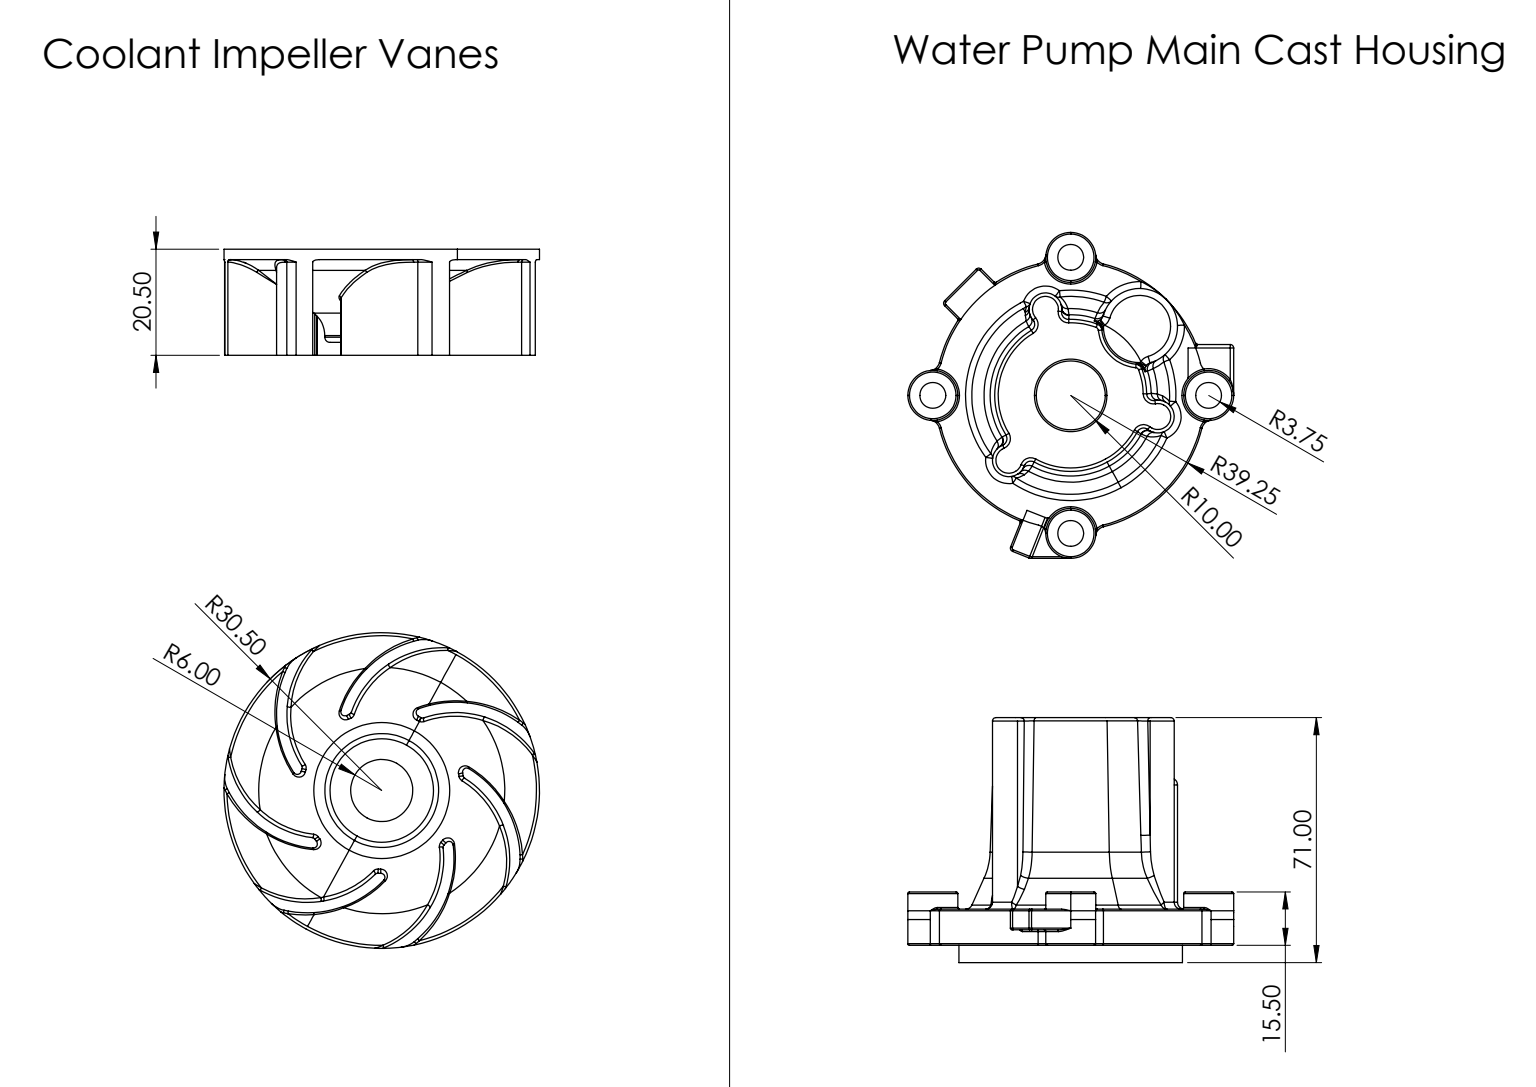
ISO-10303-21;
HEADER;
FILE_DESCRIPTION (('STEP AP214'),
    '1' );
FILE_NAME ('Coolant Impeller Vanes.step',
    '2026-10-09T13:19:41',
    ( '' ),
    ( '' ),
    'SwSTEP 2.0',
    'SolidWorks 2026',
    '' );
FILE_SCHEMA (( 'AUTOMOTIVE_DESIGN' ));
ENDSEC;

DATA;
#1=CARTESIAN_POINT ( 'NONE',  ( 13.86303783279999990, -99.69348480060000384, -10.38524229410000110 ) ) ;
#3=CARTESIAN_POINT ( 'NONE',  ( -4.209215656141860329, -99.16821844303207456, -18.57953415105935946 ) ) ;
#9=DIRECTION ( 'NONE',  ( 0.4377874319499604483, 0.000000000000000000, 0.8990785084889187928 ) ) ;
#10=CARTESIAN_POINT ( 'NONE',  ( 6.195449712719999447, -93.01125874769999768, -25.86806793289999717 ) ) ;
#12=CARTESIAN_POINT ( 'NONE',  ( -0.4517124965758896882, -92.59735406128710622, -30.49666433008702171 ) ) ;
#16=CARTESIAN_POINT ( 'NONE',  ( 0.000000000000000000, -101.2530993010000060, 0.000000000000000000 ) ) ;
#17=AXIS2_PLACEMENT_3D ( 'NONE', #8871, #7009, #22746 ) ;
#25=ORIENTED_EDGE ( 'NONE', *, *, #2852, .T. ) ;
#26=CARTESIAN_POINT ( 'NONE',  ( -13.83118819819999956, -93.00000000000000000, 21.42307711379999802 ) ) ;
#27=CARTESIAN_POINT ( 'NONE',  ( -6.649694310500000149, -97.57347470069998963, -20.16533349119999841 ) ) ;
#28=CARTESIAN_POINT ( 'NONE',  ( 7.286238495500000134, -101.2500498790000023, 13.33737010350000141 ) ) ;
#34=CARTESIAN_POINT ( 'NONE',  ( 6.962673371610000217, -93.00000450890000536, -28.64060071930000007 ) ) ;
#36=DIRECTION ( 'NONE',  ( 0.000000000000000000, 1.000000000000000000, 0.000000000000000000 ) ) ;
#37=CARTESIAN_POINT ( 'NONE',  ( -13.16349300034329239, -92.74292563041959170, 27.51314017236756015 ) ) ;
#41=CARTESIAN_POINT ( 'NONE',  ( -14.41816450560000007, -92.76166464580001048, 26.16031912729999931 ) ) ;
#42=DIRECTION ( 'NONE',  ( 0.4794255386042040601, 0.000000000000000000, 0.8775825618903719816 ) ) ;
#45=DIRECTION ( 'NONE',  ( 0.000000000000000000, -1.000000000000000000, 0.000000000000000000 ) ) ;
#48=CARTESIAN_POINT ( 'NONE',  ( 0.8512941674849999751, -100.5027207520000019, -16.22949194299999931 ) ) ;
#56=CARTESIAN_POINT ( 'NONE',  ( 28.37844821513105131, -92.77481473400868595, 11.17671000879152565 ) ) ;
#58=CARTESIAN_POINT ( 'NONE',  ( -4.347883707720000324, -95.85308664729998895, 22.07540195419999662 ) ) ;
#60=AXIS2_PLACEMENT_3D ( 'NONE', #11546, #27165, #75 ) ;
#61=CARTESIAN_POINT ( 'NONE',  ( 23.72908286170881098, -92.68577957607949713, -19.16202722645927281 ) ) ;
#62=CARTESIAN_POINT ( 'NONE',  ( 18.43702196799999982, -93.96464232210000489, 16.73647664110000122 ) ) ;
#67=CARTESIAN_POINT ( 'NONE',  ( -7.081475122079999629, -101.0678230150000019, 14.15032671260000008 ) ) ;
#70=CARTESIAN_POINT ( 'NONE',  ( -13.19299550116862640, -100.0559847774924549, -11.12607270767140477 ) ) ;
#75=DIRECTION ( 'NONE',  ( 1.000000000000000000, 0.000000000000000000, 0.000000000000000000 ) ) ;
#78=CARTESIAN_POINT ( 'NONE',  ( 11.12836528380000090, -101.0356131030000029, -10.75380786670000077 ) ) ;
#79=CARTESIAN_POINT ( 'NONE',  ( 16.21749840157504963, -94.69376227371040500, 17.23632262694635386 ) ) ;
#81=EDGE_CURVE ( 'NONE', #22088, #1149, #28672, .T. ) ;
#82=CARTESIAN_POINT ( 'NONE',  ( 26.66586753799999698, -92.50000000000000000, 13.56661073689999952 ) ) ;
#83=FACE_OUTER_BOUND ( 'NONE', #27486, .T. ) ;
#85=CARTESIAN_POINT ( 'NONE',  ( 21.68645939410062340, -94.27895761509498129, 13.53905968357343781 ) ) ;
#88=CIRCLE ( 'NONE', #11209, 30.50000000000000000 ) ;
#91=EDGE_CURVE ( 'NONE', #19757, #9289, #15248, .T. ) ;
#92=EDGE_LOOP ( 'NONE', ( #10026, #14439, #14720, #4638 ) ) ;
#95=CARTESIAN_POINT ( 'NONE',  ( -26.59811871830000030, -93.01125874769999768, -0.2839302173490000358 ) ) ;
#97=CARTESIAN_POINT ( 'NONE',  ( -13.14566783280000095, -99.53431386179998697, -11.42099844400000030 ) ) ;
#99=EDGE_LOOP ( 'NONE', ( #14663, #18599, #4684, #25899 ) ) ;
#104=AXIS2_PLACEMENT_3D ( 'NONE', #11589, #3684, #25016 ) ;
#106=ORIENTED_EDGE ( 'NONE', *, *, #502, .T. ) ;
#111=PLANE ( 'NONE',  #8405 ) ;
#112=CARTESIAN_POINT ( 'NONE',  ( 24.26002557130000170, -94.09272382170000526, -9.010767759849999337 ) ) ;
#115=CARTESIAN_POINT ( 'NONE',  ( -16.09522089960879399, -99.28262727489575923, 7.457865879375452423 ) ) ;
#116=B_SPLINE_SURFACE_WITH_KNOTS ( 'NONE', 5, 5, ( 
 ( #14625, #23526, #3562, #12417, #21334, #1390 ),
 ( #10232, #9826, #23801, #19147, #20920, #18734 ),
 ( #5874, #28035, #8074, #16964, #25852, #14753 ),
 ( #26709, #28718, #17525, #19703, #28300, #6299 ),
 ( #19988, #58, #13133, #10789, #8906, #15459 ),
 ( #11070, #6601, #22187, #4412, #6443, #17235 ) ),
 .UNSPECIFIED., .F., .F., .F.,
 ( 6, 6 ),
 ( 6, 6 ),
 ( 15.82769160610000014, 30.79604198849999719 ),
 ( 0.000000000000000000, 0.5000000000000000000 ),
 .UNSPECIFIED. ) ;
#118=CARTESIAN_POINT ( 'NONE',  ( -15.38823321699999980, -101.6484610359999863, 4.383952149800000697 ) ) ;
#124=ORIENTED_EDGE ( 'NONE', *, *, #22234, .T. ) ;
#126=CARTESIAN_POINT ( 'NONE',  ( 26.73456646982424445, -92.62800705135703083, -14.68054035958608772 ) ) ;
#129=EDGE_CURVE ( 'NONE', #4293, #10101, #28625, .T. ) ;
#130=EDGE_CURVE ( 'NONE', #14037, #19059, #13032, .T. ) ;
#137=CARTESIAN_POINT ( 'NONE',  ( 25.95077523760000204, -92.66001738319999959, 10.56845450099999972 ) ) ;
#139=VERTEX_POINT ( 'NONE', #26948 ) ;
#145=CARTESIAN_POINT ( 'NONE',  ( -12.45428620100000039, -94.22485739629999557, -21.30780079690000406 ) ) ;
#148=DIRECTION ( 'NONE',  ( 0.000000000000000000, 1.000000000000000000, 0.000000000000000000 ) ) ;
#149=CARTESIAN_POINT ( 'NONE',  ( -17.00715350810000004, -99.92967567080000890, 3.484608414699999823 ) ) ;
#154=CARTESIAN_POINT ( 'NONE',  ( 0.9512194931930000319, -99.70407914540000149, -17.16990763940000164 ) ) ;
#158=CARTESIAN_POINT ( 'NONE',  ( -7.593124578350000320, -94.98812656910000385, -22.45811535680000048 ) ) ;
#159=CIRCLE ( 'NONE', #18770, 16.00000000000000000 ) ;
#161=CARTESIAN_POINT ( 'NONE',  ( -23.83924287751435500, -92.80442066021429071, -19.02474555443098936 ) ) ;
#164=CARTESIAN_POINT ( 'NONE',  ( -14.62576901236522886, -101.1449112445098564, 4.605366063130757581 ) ) ;
#168=B_SPLINE_CURVE_WITH_KNOTS ( 'NONE', 3,
 ( #1213, #18961, #8023, #3928, #12792, #23335 ),
 .UNSPECIFIED., .F., .F.,
 ( 4, 2, 4 ),
 ( 0.000000000000000000, 0.5000000000000000000, 1.000000000000000000 ),
 .UNSPECIFIED. ) ;
#170=CIRCLE ( 'NONE', #22027, 0.8000000000000003775 ) ;
#179=CARTESIAN_POINT ( 'NONE',  ( 16.44117324919999845, -94.63960161729998788, 17.12038106740000032 ) ) ;
#180=CIRCLE ( 'NONE', #4826, 30.50000000000000000 ) ;
#181=CARTESIAN_POINT ( 'NONE',  ( 7.155402402981435372, -93.74885977083570765, -25.65720728536609840 ) ) ;
#182=CARTESIAN_POINT ( 'NONE',  ( -24.61280144410000048, -93.91547326130000783, -2.656926711870000180 ) ) ;
#185=CARTESIAN_POINT ( 'NONE',  ( 11.60289000694941208, -98.08323605844854853, -16.85433682801441435 ) ) ;
#186=ORIENTED_EDGE ( 'NONE', *, *, #11011, .T. ) ;
#189=CARTESIAN_POINT ( 'NONE',  ( -12.62382144519470906, -92.54938211474033949, 27.76503023812927395 ) ) ;
#194=CARTESIAN_POINT ( 'NONE',  ( 4.794255386040000566, -108.5000000000000000, 8.775825618900000791 ) ) ;
#196=EDGE_CURVE ( 'NONE', #27670, #21621, #4916, .T. ) ;
#198=CARTESIAN_POINT ( 'NONE',  ( 1.100347978140000071, -100.4792519539999915, -16.15648718290000119 ) ) ;
#210=DIRECTION ( 'NONE',  ( 0.000000000000000000, 1.000000000000000000, 0.000000000000000000 ) ) ;
#211=CARTESIAN_POINT ( 'NONE',  ( 14.90405967080000060, -97.14975741390000508, 15.22359678429999974 ) ) ;
#215=CARTESIAN_POINT ( 'NONE',  ( 18.38937822269999955, -93.75379239730000336, 16.85123465680000265 ) ) ;
#216=CARTESIAN_POINT ( 'NONE',  ( 0.000000000000000000, -108.5000000000000000, 0.000000000000000000 ) ) ;
#217=EDGE_CURVE ( 'NONE', #3543, #26971, #14750, .T. ) ;
#221=CARTESIAN_POINT ( 'NONE',  ( -12.45669907782013119, -101.5026031439933831, -10.21990696985948333 ) ) ;
#224=CARTESIAN_POINT ( 'NONE',  ( 7.375300558930000250, -99.32951138629999832, 16.07022401509999909 ) ) ;
#225=AXIS2_PLACEMENT_3D ( 'NONE', #24981, #531, #7212 ) ;
#229=CARTESIAN_POINT ( 'NONE',  ( 13.12744653600000078, -94.59276292389999696, -19.84842857619999990 ) ) ;
#233=CARTESIAN_POINT ( 'NONE',  ( 10.26951296328627450, -97.66504487118385214, 16.98417627201420643 ) ) ;
#235=CARTESIAN_POINT ( 'NONE',  ( 16.83483077069999823, -101.1889999979999999, 4.239603657359999112 ) ) ;
#240=CARTESIAN_POINT ( 'NONE',  ( 14.95019707169999990, -101.2530993000000024, 2.710463435110000319 ) ) ;
#244=DIRECTION ( 'NONE',  ( 1.000000000000000000, 0.000000000000000000, 0.000000000000000000 ) ) ;
#257=CARTESIAN_POINT ( 'NONE',  ( 15.94061401059999916, -100.1275643909999928, 4.799433088389999824 ) ) ;
#261=CARTESIAN_POINT ( 'NONE',  ( -19.90122868539999956, -97.01677120260001175, -7.153572992790000029 ) ) ;
#263=CARTESIAN_POINT ( 'NONE',  ( -30.47294111744043832, -92.56492639277982448, 1.288063236097679587 ) ) ;
#264=LINE ( 'NONE', #16101, #15060 ) ;
#272=CARTESIAN_POINT ( 'NONE',  ( -17.52930755215682268, -96.09960287657678180, 13.04485788190981488 ) ) ;
#273=ORIENTED_EDGE ( 'NONE', *, *, #13276, .F. ) ;
#274=DIRECTION ( 'NONE',  ( 0.000000000000000000, -1.000000000000000000, 0.000000000000000000 ) ) ;
#275=CARTESIAN_POINT ( 'NONE',  ( -3.794472973536972216, -98.68740021267650775, 19.30576947772378560 ) ) ;
#276=CARTESIAN_POINT ( 'NONE',  ( -12.75146816829999885, -100.4650220110000021, -10.99189795709999906 ) ) ;
#282=CARTESIAN_POINT ( 'NONE',  ( -1.332267629549999902E-15, -101.6484611540000031, 3.552713678799999608E-15 ) ) ;
#283=CARTESIAN_POINT ( 'NONE',  ( 0.3059185938709999553, -101.1889999979999999, 14.72672055670000013 ) ) ;
#284=CARTESIAN_POINT ( 'NONE',  ( 10.50737348100000013, -92.95010077049998642, 27.57035790109999596 ) ) ;
#286=B_SPLINE_CURVE_WITH_KNOTS ( 'NONE', 3,
 ( #13483, #9260, #22391, #17872, #13330, #22237 ),
 .UNSPECIFIED., .F., .F.,
 ( 4, 2, 4 ),
 ( 0.000000000000000000, 0.5000000000000000000, 1.000000000000000000 ),
 .UNSPECIFIED. ) ;
#289=CARTESIAN_POINT ( 'NONE',  ( -27.35150891653901084, -93.48480241393187384, -0.1005241429990150898 ) ) ;
#290=CARTESIAN_POINT ( 'NONE',  ( 19.72730657420000000, -94.57749572790000059, 14.01459989379999982 ) ) ;
#292=ORIENTED_EDGE ( 'NONE', *, *, #16592, .T. ) ;
#294=CARTESIAN_POINT ( 'NONE',  ( -25.34933364415341472, -93.66270333196791853, -5.750320990542998167 ) ) ;
#295=EDGE_CURVE ( 'NONE', #9549, #16619, #7522, .T. ) ;
#296=DIRECTION ( 'NONE',  ( -0.2162432783070587228, 0.000000000000000000, -0.9763395129702658881 ) ) ;
#298=CARTESIAN_POINT ( 'NONE',  ( -12.52668430659999999, -94.45168166330000759, -21.51447599709999992 ) ) ;
#299=CARTESIAN_POINT ( 'NONE',  ( -24.12300379919877713, -94.89420224095245260, -4.133214399626305102 ) ) ;
#303=CARTESIAN_POINT ( 'NONE',  ( -16.99615325119999909, -99.69348474340000621, 3.341833029000000010 ) ) ;
#306=CARTESIAN_POINT ( 'NONE',  ( -9.444188748147608337, -96.12507615671063377, -21.04386775914182905 ) ) ;
#308=CARTESIAN_POINT ( 'NONE',  ( 0.5505338958400000093, -101.0875971110000080, -15.39929819530000010 ) ) ;
#310=CARTESIAN_POINT ( 'NONE',  ( -11.92805169729999903, -93.25168459629999518, -23.54816055649999740 ) ) ;
#313=CARTESIAN_POINT ( 'NONE',  ( -23.96181287727355880, -92.68577957613881324, -18.87019301755865186 ) ) ;
#320=CARTESIAN_POINT ( 'NONE',  ( 17.35878545119999927, -99.60591458940000109, 0.7490350149880000696 ) ) ;
#325=CARTESIAN_POINT ( 'NONE',  ( 0.000000000000000000, -102.8486084350000027, 0.000000000000000000 ) ) ;
#327=EDGE_CURVE ( 'NONE', #28629, #9768, #11659, .T. ) ;
#328=CARTESIAN_POINT ( 'NONE',  ( 4.957296131405555251, -93.25521310932876418, -27.72106811766053980 ) ) ;
#335=CARTESIAN_POINT ( 'NONE',  ( 7.189062418559999834, -92.50000460620000808, -28.89817089330000144 ) ) ;
#337=CARTESIAN_POINT ( 'NONE',  ( -13.21000303337382675, -92.77521214512354675, 27.49085673672507468 ) ) ;
#340=CARTESIAN_POINT ( 'NONE',  ( -15.46453744689999965, -92.60980597189998775, 23.68301408729999835 ) ) ;
#343=CARTESIAN_POINT ( 'NONE',  ( -17.63662366879999865, -94.54719310779999830, 16.06392309460000334 ) ) ;
#344=CARTESIAN_POINT ( 'NONE',  ( 0.9125455711469999676, -100.1785804069999983, -16.62377051789999882 ) ) ;
#348=CARTESIAN_POINT ( 'NONE',  ( 6.888451995309999631, -99.53431386179998697, 15.99365561480000153 ) ) ;
#349=ORIENTED_EDGE ( 'NONE', *, *, #6891, .T. ) ;
#350=CARTESIAN_POINT ( 'NONE',  ( -17.51528407220000361, -94.37182379849998881, 16.53944417690000179 ) ) ;
#351=CARTESIAN_POINT ( 'NONE',  ( 15.38595020189201179, -101.1586404113103015, 2.789465265516761772 ) ) ;
#353=CARTESIAN_POINT ( 'NONE',  ( 19.89028060919999774, -94.80026829410000744, 14.17835456439999930 ) ) ;
#355=CARTESIAN_POINT ( 'NONE',  ( 23.48150327141549099, -92.56772982771099123, -19.46465348493570957 ) ) ;
#358=B_SPLINE_SURFACE_WITH_KNOTS ( 'NONE', 5, 5, ( 
 ( #10209, #18565, #20758, #23504, #23087, #27741, #25691, #27609, #3542 ),
 ( #25277, #12127, #816, #21309, #7649, #19123, #16212, #964, #25125 ),
 ( #5159, #25412, #3402, #14040, #9658, #22946, #14328, #16367, #23222 ),
 ( #11846, #27457, #5305, #3131, #20898, #16516, #5443, #3270, #21043 ),
 ( #1100, #7777, #16650, #25544, #14467, #23361, #23634, #1928, #28278 ),
 ( #19396, #15144, #19819, #4092, #28424, #23917, #3954, #12678, #10767 ) ),
 .UNSPECIFIED., .F., .F., .F.,
 ( 6, 6 ),
 ( 6, 3, 6 ),
 ( 10.27983419480000116, 28.98451109560000205 ),
 ( 0.000000000000000000, 0.2500000000000000000, 0.5000000000000000000 ),
 .UNSPECIFIED. ) ;
#362=CARTESIAN_POINT ( 'NONE',  ( -12.45203970512436165, -101.4728631013286559, -10.26186846076686443 ) ) ;
#373=CYLINDRICAL_SURFACE ( 'NONE', #27643, 15.99999999999999822 ) ;
#374=CARTESIAN_POINT ( 'NONE',  ( -14.95854026159999961, -100.9763033870000015, 4.709388778109999230 ) ) ;
#375=CARTESIAN_POINT ( 'NONE',  ( -17.31644382271060323, -99.07183861590023355, -8.238310338614811101 ) ) ;
#379=CARTESIAN_POINT ( 'NONE',  ( 0.000000000000000000, -101.6484611540000031, 0.000000000000000000 ) ) ;
#380=CARTESIAN_POINT ( 'NONE',  ( 24.72812962333588160, -93.39299082536693675, -12.36525841036616313 ) ) ;
#382=ORIENTED_EDGE ( 'NONE', *, *, #3847, .F. ) ;
#386=CARTESIAN_POINT ( 'NONE',  ( 23.63616061750000341, -94.63960162979999780, -2.179844042860000108 ) ) ;
#389=CARTESIAN_POINT ( 'NONE',  ( 29.11677867130000052, -92.50000000000000000, 6.880015861159999524 ) ) ;
#391=ADVANCED_FACE ( 'NONE', ( #7256 ), #13212, .F. ) ;
#393=CARTESIAN_POINT ( 'NONE',  ( 16.66712582699999956, -100.0994409990000094, 4.341523580040000496 ) ) ;
#397=EDGE_CURVE ( 'NONE', #15581, #14037, #15975, .T. ) ;
#399=CARTESIAN_POINT ( 'NONE',  ( -20.09682587570000223, -97.23151480800000002, -7.274462301079999804 ) ) ;
#401=CARTESIAN_POINT ( 'NONE',  ( -30.44002477821454633, -92.69183043801065480, 1.913949942781201674 ) ) ;
#402=DIRECTION ( 'NONE',  ( 0.6184463001828860440, 0.000000000000000000, 0.7858270635388550085 ) ) ;
#403=DIRECTION ( 'NONE',  ( 0.4794255386042042266, 0.000000000000000000, 0.8775825618903720926 ) ) ;
#406=CARTESIAN_POINT ( 'NONE',  ( 22.78264864029999970, -94.59276292120000562, -6.873201003520000185 ) ) ;
#407=TOROIDAL_SURFACE ( 'NONE', #6924, 18.14285714289999873, 0.5000000000000000000 ) ;
#410=CARTESIAN_POINT ( 'NONE',  ( 13.82833792859999811, -99.73367660430000115, -10.41122475269999903 ) ) ;
#411=ORIENTED_EDGE ( 'NONE', *, *, #8688, .T. ) ;
#415=CARTESIAN_POINT ( 'NONE',  ( -13.27698888679999989, -99.83167681540000160, -11.13684395419999973 ) ) ;
#416=CARTESIAN_POINT ( 'NONE',  ( -12.76745321220000129, -101.1364147039999892, -8.514038431850000421 ) ) ;
#417=CARTESIAN_POINT ( 'NONE',  ( 16.58537890990000108, -94.98812477769999418, 16.93952572510000110 ) ) ;
#427=CARTESIAN_POINT ( 'NONE',  ( 10.51978096080000213, -92.52763213160000078, 27.11043680749999751 ) ) ;
#430=CIRCLE ( 'NONE', #7407, 0.4999999999999993339 ) ;
#435=ORIENTED_EDGE ( 'NONE', *, *, #15676, .F. ) ;
#438=DIRECTION ( 'NONE',  ( 1.000000000000000000, 0.000000000000000000, 0.000000000000000000 ) ) ;
#439=CARTESIAN_POINT ( 'NONE',  ( -14.10155798110000092, -93.81709628049999594, -21.57370430179999943 ) ) ;
#440=CARTESIAN_POINT ( 'NONE',  ( -24.00582547640926379, -94.71481465629901209, -4.132763972591003032 ) ) ;
#441=ORIENTED_EDGE ( 'NONE', *, *, #13396, .T. ) ;
#443=CARTESIAN_POINT ( 'NONE',  ( -17.09009608839999927, -99.55609322370000314, 3.193624944930000265 ) ) ;
#446=ORIENTED_EDGE ( 'NONE', *, *, #18563, .T. ) ;
#447=B_SPLINE_CURVE_WITH_KNOTS ( 'NONE', 3,
 ( #7135, #24608, #16144, #11221, #2517, #21773, #21492, #4538, #15745, #9188 ),
 .UNSPECIFIED., .F., .F.,
 ( 4, 2, 2, 2, 4 ),
 ( 0.000000000000000000, 0.2500000000000000000, 0.5000000000000000000, 0.7500000000000000000, 1.000000000000000000 ),
 .UNSPECIFIED. ) ;
#449=DIRECTION ( 'NONE',  ( 0.000000000000000000, 1.000000000000000000, 0.000000000000000000 ) ) ;
#450=DIRECTION ( 'NONE',  ( 0.000000000000000000, -1.000000000000000000, 0.000000000000000000 ) ) ;
#457=AXIS2_PLACEMENT_3D ( 'NONE', #1882, #15240, #28107 ) ;
#460=CARTESIAN_POINT ( 'NONE',  ( 15.94843830448696487, -101.0147714271772088, 4.203990814596493486 ) ) ;
#465=B_SPLINE_CURVE_WITH_KNOTS ( 'NONE', 5,
 ( #5943, #23459, #23728, #10162, #18944, #17165, #14693, #26054, #14961, #21544, #25785, #21403 ),
 .UNSPECIFIED., .F., .F.,
 ( 6, 3, 3, 6 ),
 ( 0.000000000000000000, 0.4964111757582199136, 0.7833083924326244007, 1.000000000000000000 ),
 .UNSPECIFIED. ) ;
#475=CARTESIAN_POINT ( 'NONE',  ( 9.119802927630001221, -98.28914429610000525, 16.69368728350000097 ) ) ;
#485=CARTESIAN_POINT ( 'NONE',  ( 11.45574570990000041, -93.13207089280000162, -23.61394595179999811 ) ) ;
#487=CARTESIAN_POINT ( 'NONE',  ( -13.33479272893357859, -92.93978723899297734, 27.43052168310984840 ) ) ;
#491=CARTESIAN_POINT ( 'NONE',  ( 14.34373124439999891, -102.5000000000000000, 26.25602392650000283 ) ) ;
#493=CARTESIAN_POINT ( 'NONE',  ( -18.48642635659999911, -96.07607726710000406, 13.72266607319999920 ) ) ;
#494=CARTESIAN_POINT ( 'NONE',  ( 0.6457915530089999301, -99.58396362730000817, -17.35065848859999704 ) ) ;
#502=EDGE_CURVE ( 'NONE', #19526, #5924, #14185, .T. ) ;
#508=CARTESIAN_POINT ( 'NONE',  ( 10.14179094049999819, -99.62155479429999616, 14.52072615979999881 ) ) ;
#511=CARTESIAN_POINT ( 'NONE',  ( 26.37318048140000215, -93.00000450890000536, 13.16123783449999962 ) ) ;
#512=DIRECTION ( 'NONE',  ( 0.000000000000000000, 1.000000000000000000, 0.000000000000000000 ) ) ;
#514=CARTESIAN_POINT ( 'NONE',  ( -6.885095864830000245, -101.1417990620000040, 14.17428525849999943 ) ) ;
#516=CARTESIAN_POINT ( 'NONE',  ( -12.61948338259999858, -101.6484611540000031, -9.836088610590000059 ) ) ;
#520=CIRCLE ( 'NONE', #16773, 5.000000000000000888 ) ;
#521=CARTESIAN_POINT ( 'NONE',  ( 7.321257786130000333, -99.28585527969998736, 16.15667156069999777 ) ) ;
#523=CARTESIAN_POINT ( 'NONE',  ( -3.773308002759999891, -96.65227117080000596, -20.92579437230000039 ) ) ;
#531=DIRECTION ( 'NONE',  ( 0.000000000000000000, 1.000000000000000000, 0.000000000000000000 ) ) ;
#539=CIRCLE ( 'NONE', #15843, 30.50000000000000000 ) ;
#542=CARTESIAN_POINT ( 'NONE',  ( -19.01557598121447157, -92.50000000001456613, 22.91712378798360916 ) ) ;
#543=CARTESIAN_POINT ( 'NONE',  ( 28.83687378200000140, -92.50000647099999185, 7.262115126140000321 ) ) ;
#545=CARTESIAN_POINT ( 'NONE',  ( -19.98788946392987853, -95.81531090358907932, 9.701109111489476078 ) ) ;
#547=ORIENTED_EDGE ( 'NONE', *, *, #12350, .T. ) ;
#549=CARTESIAN_POINT ( 'NONE',  ( -24.15517241699999929, -94.98812769030000425, -4.102690932189999806 ) ) ;
#551=CARTESIAN_POINT ( 'NONE',  ( 8.639505966715979923, -92.69183043846588532, 29.25093587448420962 ) ) ;
#552=CARTESIAN_POINT ( 'NONE',  ( 0.3872056760440000245, -99.92967571559999840, -17.35614698070000017 ) ) ;
#557=DIRECTION ( 'NONE',  ( 0.9982579106777251798, 0.000000000000000000, -0.05900121837168281064 ) ) ;
#558=CIRCLE ( 'NONE', #25661, 18.64285714289999873 ) ;
#562=CARTESIAN_POINT ( 'NONE',  ( 14.21256893470000193, -98.58303758080000989, -12.13706782569999909 ) ) ;
#567=CARTESIAN_POINT ( 'NONE',  ( 7.891778559019607009, -101.5538022607323683, 14.00007649551812072 ) ) ;
#571=ADVANCED_FACE ( 'NONE', ( #26925 ), #15677, .T. ) ;
#572=CARTESIAN_POINT ( 'NONE',  ( 26.38387423984804769, -92.80045754842753070, -15.30171679607595259 ) ) ;
#573=ORIENTED_EDGE ( 'NONE', *, *, #1821, .F. ) ;
#576=CARTESIAN_POINT ( 'NONE',  ( -4.045235864600000397, -98.43722212099999069, 19.19069134749999961 ) ) ;
#578=CARTESIAN_POINT ( 'NONE',  ( 8.074115162410000934, -92.66424957140000629, 26.74225754210000261 ) ) ;
#589=EDGE_CURVE ( 'NONE', #21458, #13839, #9040, .T. ) ;
#590=CARTESIAN_POINT ( 'NONE',  ( 7.367077158260816994, -101.1416252679887577, 13.68480675837215799 ) ) ;
#596=CARTESIAN_POINT ( 'NONE',  ( -16.91403943069999727, -99.72583475830001021, 3.025870399720000048 ) ) ;
#602=CARTESIAN_POINT ( 'NONE',  ( 0.7331063123750001242, -99.53431386179998697, -17.39857302659999760 ) ) ;
#606=CARTESIAN_POINT ( 'NONE',  ( -9.465083148179999739, -93.62676565499999981, -23.38439984080000045 ) ) ;
#610=CARTESIAN_POINT ( 'NONE',  ( 16.28778070538160350, -100.5550990449209223, 4.345266980774773913 ) ) ;
#612=ORIENTED_EDGE ( 'NONE', *, *, #9543, .F. ) ;
#620=ORIENTED_EDGE ( 'NONE', *, *, #6006, .F. ) ;
#621=CARTESIAN_POINT ( 'NONE',  ( 0.000000000000000000, -102.5000000000000000, 0.000000000000000000 ) ) ;
#622=CARTESIAN_POINT ( 'NONE',  ( 9.335817441747641610, -98.58684426249028832, 16.46450815360437048 ) ) ;
#627=CARTESIAN_POINT ( 'NONE',  ( -22.27191869549999836, -94.59276292389999696, -8.381623179300000004 ) ) ;
#629=CARTESIAN_POINT ( 'NONE',  ( -18.14789115860000024, -98.53904439360000822, 4.701750000830000609 ) ) ;
#630=CARTESIAN_POINT ( 'NONE',  ( -0.5455113252076949637, -98.53908159007990264, -18.73906669024530913 ) ) ;
#632=EDGE_LOOP ( 'NONE', ( #19632, #17486, #11324, #22339 ) ) ;
#633=CARTESIAN_POINT ( 'NONE',  ( 13.03263341399999931, -94.63960343439998724, -19.83860458410000049 ) ) ;
#641=CARTESIAN_POINT ( 'NONE',  ( -18.40263696530000104, -95.90090461900000207, 13.63749173159999906 ) ) ;
#642=CARTESIAN_POINT ( 'NONE',  ( 0.7331063045040000503, -99.53431386179998697, -17.39857310140000024 ) ) ;
#649=ORIENTED_EDGE ( 'NONE', *, *, #27398, .T. ) ;
#652=CARTESIAN_POINT ( 'NONE',  ( 8.185345124539999517, -101.3150701389999995, 14.03998254610000096 ) ) ;
#653=ORIENTED_EDGE ( 'NONE', *, *, #17240, .T. ) ;
#657=CARTESIAN_POINT ( 'NONE',  ( -7.569816714379999922, -100.7776802639999971, 13.87827956499999971 ) ) ;
#658=CARTESIAN_POINT ( 'NONE',  ( -12.66558680574216922, -93.40492137171338527, -23.55307789253798845 ) ) ;
#661=CARTESIAN_POINT ( 'NONE',  ( 7.318052426040000391, -101.1822553929999913, 13.41977313900000013 ) ) ;
#662=ORIENTED_EDGE ( 'NONE', *, *, #22175, .F. ) ;
#667=ORIENTED_EDGE ( 'NONE', *, *, #3117, .T. ) ;
#670=CARTESIAN_POINT ( 'NONE',  ( 11.85549584000000145, -101.3350617309999961, -10.77753387699999976 ) ) ;
#672=CARTESIAN_POINT ( 'NONE',  ( 15.48878798707903925, -95.04305759974297985, 17.29288121155813585 ) ) ;
#679=CARTESIAN_POINT ( 'NONE',  ( -14.88706571849999882, -101.2269841009999993, 3.209819282999999857 ) ) ;
#683=CARTESIAN_POINT ( 'NONE',  ( -18.13877362739999910, -92.50000000000000000, -23.79298866759999598 ) ) ;
#685=CARTESIAN_POINT ( 'NONE',  ( 21.27776255609999723, -96.58372173029999885, 1.059637706860000028 ) ) ;
#690=CARTESIAN_POINT ( 'NONE',  ( 0.4125572470530000091, -92.84292833370000153, -30.36594662649999776 ) ) ;
#692=CARTESIAN_POINT ( 'NONE',  ( 16.40194905730000130, -100.1981337080000003, 4.404945126920000398 ) ) ;
#695=CARTESIAN_POINT ( 'NONE',  ( 8.185346967789998374, -101.3150701389999995, 14.03998109830000018 ) ) ;
#696=CARTESIAN_POINT ( 'NONE',  ( -22.25469472199999998, -96.07623048470000526, -5.897558151980000218 ) ) ;
#697=ORIENTED_EDGE ( 'NONE', *, *, #27258, .F. ) ;
#698=CARTESIAN_POINT ( 'NONE',  ( -30.48402335599918800, -92.52498922770503498, 0.9899291096564720727 ) ) ;
#701=DIRECTION ( 'NONE',  ( 0.000000000000000000, -1.000000000000000000, 0.000000000000000000 ) ) ;
#709=CARTESIAN_POINT ( 'NONE',  ( 14.00782577689999897, -96.65227117100000953, -15.99711037630000021 ) ) ;
#715=CARTESIAN_POINT ( 'NONE',  ( 11.77298154309999845, -101.2530993010000060, -9.604785791470000333 ) ) ;
#722=CARTESIAN_POINT ( 'NONE',  ( 2.631283596650000334, -94.29487537309999823, 25.29847487550000196 ) ) ;
#724=CARTESIAN_POINT ( 'NONE',  ( -11.18835776723661724, -94.77533639018899692, -20.78536094536529077 ) ) ;
#725=CIRCLE ( 'NONE', #16980, 18.64285714289999518 ) ;
#726=VERTEX_POINT ( 'NONE', #19037 ) ;
#727=CARTESIAN_POINT ( 'NONE',  ( -26.32546053305905076, -93.86130746203110675, -1.655768764585977548 ) ) ;
#740=CYLINDRICAL_SURFACE ( 'NONE', #28427, 5.000000000000000000 ) ;
#744=CARTESIAN_POINT ( 'NONE',  ( -15.62495981729999883, -101.3646851630000043, 3.472370199919999845 ) ) ;
#747=EDGE_LOOP ( 'NONE', ( #26424, #26914 ) ) ;
#749=CARTESIAN_POINT ( 'NONE',  ( -13.83118819819999956, -93.00000000000000000, 21.42307711379999802 ) ) ;
#752=DIRECTION ( 'NONE',  ( 1.000000000000000000, 0.000000000000000000, 0.000000000000000000 ) ) ;
#755=CARTESIAN_POINT ( 'NONE',  ( 15.63673621517384227, -101.5526869446983511, 3.723052656565844831 ) ) ;
#763=CARTESIAN_POINT ( 'NONE',  ( 2.113568700161239988, -94.60931859130616317, 24.93618714997996122 ) ) ;
#769=CARTESIAN_POINT ( 'NONE',  ( -5.360408304419999936, -101.0356131030000029, 14.51726283890000069 ) ) ;
#772=ADVANCED_FACE ( 'NONE', ( #13764 ), #9092, .T. ) ;
#784=CARTESIAN_POINT ( 'NONE',  ( 15.50655985760000100, -100.4792519539999915, 4.667916574389999518 ) ) ;
#788=CARTESIAN_POINT ( 'NONE',  ( -12.40956463280000044, -101.1716782170000073, -9.672470230850001016 ) ) ;
#791=CARTESIAN_POINT ( 'NONE',  ( -16.41347552970000123, -99.62149529559999905, 6.656434160910000841 ) ) ;
#795=DIRECTION ( 'NONE',  ( 1.000000000000000000, 0.000000000000000000, 0.000000000000000000 ) ) ;
#801=CARTESIAN_POINT ( 'NONE',  ( 12.48171397640000180, -98.43722862079999913, 15.12788944299999905 ) ) ;
#802=ORIENTED_EDGE ( 'NONE', *, *, #21545, .T. ) ;
#805=CARTESIAN_POINT ( 'NONE',  ( -11.67423268237357448, -95.07100787631300420, -21.41835470664000596 ) ) ;
#807=CARTESIAN_POINT ( 'NONE',  ( -17.09958374329999842, -92.50686295190000408, -23.80106955060000118 ) ) ;
#808=CARTESIAN_POINT ( 'NONE',  ( -7.939103275319999042, -100.2511768809999921, 14.67510867289999865 ) ) ;
#811=CYLINDRICAL_SURFACE ( 'NONE', #10352, 0.7499999999999991118 ) ;
#815=FACE_OUTER_BOUND ( 'NONE', #4729, .T. ) ;
#816=CARTESIAN_POINT ( 'NONE',  ( 12.08846704350000145, -99.82967635420000363, -13.24263972569999837 ) ) ;
#821=CARTESIAN_POINT ( 'NONE',  ( -18.09364012780129372, -92.54687141712491893, 24.55341606856252312 ) ) ;
#824=DIRECTION ( 'NONE',  ( 0.000000000000000000, -1.000000000000000000, 0.000000000000000000 ) ) ;
#825=CARTESIAN_POINT ( 'NONE',  ( -17.12548553040000243, -99.53431416519998720, 3.156821174210000081 ) ) ;
#828=CYLINDRICAL_SURFACE ( 'NONE', #23410, 16.00000000000000000 ) ;
#829=CARTESIAN_POINT ( 'NONE',  ( 7.493565752170000316, -101.1298585160000130, 13.45843171979999831 ) ) ;
#837=CARTESIAN_POINT ( 'NONE',  ( 13.81100091409999919, -101.1889999979999999, -10.51865105429999936 ) ) ;
#838=DIRECTION ( 'NONE',  ( 1.000000000000000000, 0.000000000000000000, 0.000000000000000000 ) ) ;
#840=CARTESIAN_POINT ( 'NONE',  ( -5.459548099580000091, -101.1364147039999892, 14.34189828759999941 ) ) ;
#841=CARTESIAN_POINT ( 'NONE',  ( -20.16249632440000283, -93.14733754460000625, 18.54048584069999706 ) ) ;
#842=VERTEX_POINT ( 'NONE', #27887 ) ;
#843=CARTESIAN_POINT ( 'NONE',  ( -30.43382723913022403, -92.71525149887465034, 2.010643618899957019 ) ) ;
#844=CARTESIAN_POINT ( 'NONE',  ( 0.5993989555620130583, -100.8061861239892067, -16.64687443652875132 ) ) ;
#848=CARTESIAN_POINT ( 'NONE',  ( 23.34631240599999913, -94.16701134370001114, -7.441733273619999700 ) ) ;
#850=CARTESIAN_POINT ( 'NONE',  ( 23.87011249777025412, -92.83160374581406415, -18.98598802258993246 ) ) ;
#856=CARTESIAN_POINT ( 'NONE',  ( 8.125631349740000786, -111.0000000000000000, 24.17072847820000092 ) ) ;
#857=CARTESIAN_POINT ( 'NONE',  ( 15.34608781240000042, -101.0356131030000029, 1.995616791270000023 ) ) ;
#866=CARTESIAN_POINT ( 'NONE',  ( -4.870171913750000137, -99.56347590840000805, 16.86609011349999676 ) ) ;
#867=CARTESIAN_POINT ( 'NONE',  ( 1.495931207609999980, -94.52292840100000149, 23.88472403519999787 ) ) ;
#869=ORIENTED_EDGE ( 'NONE', *, *, #25177, .F. ) ;
#874=CARTESIAN_POINT ( 'NONE',  ( -2.903039748510000351, -94.98812477769999418, 23.52859306979999943 ) ) ;
#877=DIRECTION ( 'NONE',  ( 0.000000000000000000, -1.000000000000000000, 0.000000000000000000 ) ) ;
#878=ORIENTED_EDGE ( 'NONE', *, *, #8574, .T. ) ;
#884=CARTESIAN_POINT ( 'NONE',  ( -15.68327981119999670, -101.1552388829999956, 3.291924952050000019 ) ) ;
#895=CARTESIAN_POINT ( 'NONE',  ( 16.39931659300885514, -100.4166221066841587, 4.355705164862286871 ) ) ;
#901=AXIS2_PLACEMENT_3D ( 'NONE', #9797, #12393, #21304 ) ;
#906=CARTESIAN_POINT ( 'NONE',  ( 3.767790178086171782, -94.00299386466799945, 25.81181420351906297 ) ) ;
#909=CARTESIAN_POINT ( 'NONE',  ( 22.85993602570000149, -94.54719592029999831, -6.820848577220000486 ) ) ;
#913=CARTESIAN_POINT ( 'NONE',  ( -5.598527377420000839, -101.2141467319999890, 14.18131542549999935 ) ) ;
#915=FACE_OUTER_BOUND ( 'NONE', #3176, .T. ) ;
#918=CARTESIAN_POINT ( 'NONE',  ( 23.52740994132569341, -94.89420224091314537, -6.742681588792337699 ) ) ;
#924=CARTESIAN_POINT ( 'NONE',  ( 19.88643906569999942, -97.93128678309999202, 2.148978528179999792 ) ) ;
#925=CARTESIAN_POINT ( 'NONE',  ( -20.57672323510000112, -92.65509245750000389, 18.55002133529999853 ) ) ;
#926=CARTESIAN_POINT ( 'NONE',  ( 14.80905440220000102, -101.2358105800000061, 3.500992360309999718 ) ) ;
#927=VERTEX_POINT ( 'NONE', #21470 ) ;
#932=CARTESIAN_POINT ( 'NONE',  ( -17.06681816329999890, -98.24294206849999966, 8.836829391780000265 ) ) ;
#941=EDGE_CURVE ( 'NONE', #25484, #19516, #6323, .T. ) ;
#950=CARTESIAN_POINT ( 'NONE',  ( 7.584268328590000330, -101.6484612600000048, 14.08825304710000026 ) ) ;
#955=CARTESIAN_POINT ( 'NONE',  ( -7.808702190560000034, -100.5027207520000019, 14.25290428609999971 ) ) ;
#959=LINE ( 'NONE', #23355, #1352 ) ;
#964=CARTESIAN_POINT ( 'NONE',  ( 11.50033716490000124, -99.57131247680000286, -13.08529392099999988 ) ) ;
#967=CYLINDRICAL_SURFACE ( 'NONE', #8348, 16.00000000000000711 ) ;
#974=CARTESIAN_POINT ( 'NONE',  ( -16.13894939720000110, -100.3684138120000000, 2.534589637169999854 ) ) ;
#976=EDGE_CURVE ( 'NONE', #2923, #24336, #19701, .T. ) ;
#977=B_SPLINE_CURVE_WITH_KNOTS ( 'NONE', 5,
 ( #1268, #16978, #25726, #6621, #28740, #10949, #22067, #6463, #6321, #3993, #21918, #12853 ),
 .UNSPECIFIED., .F., .F.,
 ( 6, 3, 3, 6 ),
 ( 0.000000000000000000, 0.4964111757593155927, 0.7833083924321462277, 1.000000000000000000 ),
 .UNSPECIFIED. ) ;
#978=CARTESIAN_POINT ( 'NONE',  ( 6.983903848129999758, -101.1716782170000073, 14.09890285740000060 ) ) ;
#980=CARTESIAN_POINT ( 'NONE',  ( -11.71812394180000005, -95.05064612279998926, -21.42448367849999968 ) ) ;
#983=CARTESIAN_POINT ( 'NONE',  ( 26.73328265790000202, -93.00000450890000536, -12.41349335419999989 ) ) ;
#987=ORIENTED_EDGE ( 'NONE', *, *, #21643, .T. ) ;
#988=CARTESIAN_POINT ( 'NONE',  ( -17.05934341600000081, -99.58396357329999660, 3.231284207160000310 ) ) ;
#992=CARTESIAN_POINT ( 'NONE',  ( 0.5973072979270338534, -100.4166221066882656, -16.95738706857987310 ) ) ;
#995=CARTESIAN_POINT ( 'NONE',  ( -12.53380938399999955, -99.91102932029998840, -11.37771751150000021 ) ) ;
#997=CARTESIAN_POINT ( 'NONE',  ( -6.754619094799999779, -97.17811284689999241, -19.41490638410000003 ) ) ;
#998=CARTESIAN_POINT ( 'NONE',  ( 13.90581089109999979, -96.83679385050000121, -16.07632342850000029 ) ) ;
#1002=EDGE_CURVE ( 'NONE', #1715, #20804, #12259, .T. ) ;
#1003=FILL_AREA_STYLE_COLOUR ( '', #22561 ) ;
#1004=AXIS2_PLACEMENT_3D ( 'NONE', #7236, #15807, #16248 ) ;
#1011=CARTESIAN_POINT ( 'NONE',  ( -2.163692630959999974, -97.01506441819999793, 20.66419130159999895 ) ) ;
#1013=VERTEX_POINT ( 'NONE', #20588 ) ;
#1015=CARTESIAN_POINT ( 'NONE',  ( -28.90627101076691119, -93.08694455166653370, 3.225356627808906751 ) ) ;
#1017=CARTESIAN_POINT ( 'NONE',  ( 1.535001344007000501, -93.33134965528456917, 26.92859106544546677 ) ) ;
#1019=CIRCLE ( 'NONE', #13531, 23.79684788999999867 ) ;
#1020=DIRECTION ( 'NONE',  ( 0.4794255386042041156, 0.000000000000000000, 0.8775825618903722036 ) ) ;
#1021=DIRECTION ( 'NONE',  ( 0.000000000000000000, -1.000000000000000000, 0.000000000000000000 ) ) ;
#1026=CARTESIAN_POINT ( 'NONE',  ( 7.525098751867413505, -101.3051320485135989, 13.97834179997459891 ) ) ;
#1029=PRODUCT_DEFINITION ( 'UNKNOWN', '', #24580, #27815 ) ;
#1034=CARTESIAN_POINT ( 'NONE',  ( -14.98642683749999982, -101.1746813909999929, 3.063272132379999846 ) ) ;
#1041=CARTESIAN_POINT ( 'NONE',  ( -7.919443313535407647, -100.1406256087997946, 15.25681078078310193 ) ) ;
#1043=EDGE_CURVE ( 'NONE', #4106, #10296, #15561, .T. ) ;
#1045=CARTESIAN_POINT ( 'NONE',  ( 15.73209904307306495, -101.3586211804324364, 3.965908164571182670 ) ) ;
#1047=ORIENTED_EDGE ( 'NONE', *, *, #26762, .F. ) ;
#1050=AXIS2_PLACEMENT_3D ( 'NONE', #23123, #18318, #2882 ) ;
#1051=CARTESIAN_POINT ( 'NONE',  ( 6.505013304209224856, -93.40023634520538565, 26.84593531204708938 ) ) ;
#1052=EDGE_LOOP ( 'NONE', ( #19310, #18086, #18495, #5928 ) ) ;
#1054=VERTEX_POINT ( 'NONE', #22778 ) ;
#1056=CARTESIAN_POINT ( 'NONE',  ( -6.285925807539999965, -101.5369810359999860, 14.71350185169999847 ) ) ;
#1064=CARTESIAN_POINT ( 'NONE',  ( 16.79767991550562201, -99.84800943041638277, 4.262183576306437516 ) ) ;
#1071=CARTESIAN_POINT ( 'NONE',  ( 24.01308097620000126, -92.92146929989999649, -18.61461950569999857 ) ) ;
#1076=ADVANCED_FACE ( 'NONE', ( #16501 ), #12110, .F. ) ;
#1079=CARTESIAN_POINT ( 'NONE',  ( -8.209463884390000743, -99.53431386179998697, 15.35748973489999969 ) ) ;
#1083=AXIS2_PLACEMENT_3D ( 'NONE', #14215, #2856, #27761 ) ;
#1095=CARTESIAN_POINT ( 'NONE',  ( 7.294752286439998734, -101.1411471520000021, 13.55045874839999875 ) ) ;
#1100=CARTESIAN_POINT ( 'NONE',  ( 10.68340813570000059, -96.16784750930000314, -20.42747610590000207 ) ) ;
#1101=EDGE_LOOP ( 'NONE', ( #18516, #25126, #4373, #25716 ) ) ;
#1103=B_SPLINE_CURVE_WITH_KNOTS ( 'NONE', 3,
 ( #9770, #5554, #23742, #18682, #27581, #25387, #8018, #5415, #3375, #10178, #3240, #19095, #16908, #25801, #5827, #6247, #3923, #15110, #4358, #6542, #4056, #26358, #12787, #14974, #12922, #28246, #1743, #1892, #15250, #21839, #24171, #21695, #10730 ),
 .UNSPECIFIED., .F., .F.,
 ( 4, 2, 1, 1, 2, 2, 1, 1, 1, 2, 2, 2, 1, 1, 2, 2, 1, 1, 2, 2, 4 ),
 ( 0.000000000000000000, 0.06250000000012244372, 0.09375000000017180701, 0.1093750000001865452, 0.1171875000001930262, 0.1250000000001995071, 0.1875000000001214029, 0.2187500000000817679, 0.2343750000000625888, 0.2421875000000536238, 0.2500000000000446310, 0.3750000000000313083, 0.4375000000000246470, 0.4687500000000220379, 0.4843750000000230371, 0.5000000000000239808, 0.6250000000000188738, 0.6875000000000155431, 0.7187500000000137668, 0.7500000000000119904, 1.000000000000000000 ),
 .UNSPECIFIED. ) ;
#1105=CARTESIAN_POINT ( 'NONE',  ( 11.96217641910000040, -101.6484611580000035, -10.62652795770000047 ) ) ;
#1108=CARTESIAN_POINT ( 'NONE',  ( -16.54318588419999969, -93.00000000000000000, 25.62368046950000178 ) ) ;
#1111=CARTESIAN_POINT ( 'NONE',  ( 11.91621941349511360, -101.5902664364218992, -10.74252197561657773 ) ) ;
#1113=CARTESIAN_POINT ( 'NONE',  ( 9.154723059868985047, -100.7167546688124986, 14.37589150456371279 ) ) ;
#1115=VERTEX_POINT ( 'NONE', #11677 ) ;
#1117=CARTESIAN_POINT ( 'NONE',  ( 13.79150630012393286, -97.05288880406236274, -15.91483940542160269 ) ) ;
#1119=CARTESIAN_POINT ( 'NONE',  ( -11.31832638660000079, -94.71194659750000255, -20.80844780490000190 ) ) ;
#1123=DIRECTION ( 'NONE',  ( 0.000000000000000000, 1.000000000000000000, 0.000000000000000000 ) ) ;
#1125=CARTESIAN_POINT ( 'NONE',  ( -18.09563929800284754, -93.31462968090272625, -21.26308191278070936 ) ) ;
#1127=ORIENTED_EDGE ( 'NONE', *, *, #23270, .T. ) ;
#1128=CARTESIAN_POINT ( 'NONE',  ( 8.069590842209999337, -101.0685850230000113, 13.92289867959999938 ) ) ;
#1129=CARTESIAN_POINT ( 'NONE',  ( -17.03413894869999723, -99.61736770250000461, 3.268853260370000235 ) ) ;
#1135=CARTESIAN_POINT ( 'NONE',  ( 0.5079992097761589775, -100.1240332945069724, -17.19565627508607264 ) ) ;
#1136=DIRECTION ( 'NONE',  ( 0.000000000000000000, -1.000000000000000000, 0.000000000000000000 ) ) ;
#1138=CARTESIAN_POINT ( 'NONE',  ( 13.25691510293539821, -92.77521214512113090, 27.46826507470851197 ) ) ;
#1143=CARTESIAN_POINT ( 'NONE',  ( 13.12744029750000152, -94.59276292389999696, -19.84843707589999795 ) ) ;
#1149=VERTEX_POINT ( 'NONE', #23899 ) ;
#1151=EDGE_CURVE ( 'NONE', #12597, #24336, #725, .T. ) ;
#1154=CARTESIAN_POINT ( 'NONE',  ( -28.83106611000000186, -92.65997669530000280, 3.154919777930000002 ) ) ;
#1157=ORIENTED_EDGE ( 'NONE', *, *, #26762, .T. ) ;
#1163=ORIENTED_EDGE ( 'NONE', *, *, #18541, .F. ) ;
#1166=CARTESIAN_POINT ( 'NONE',  ( -14.70126722260000030, -101.0847364069999941, 4.628494549459999163 ) ) ;
#1167=CARTESIAN_POINT ( 'NONE',  ( -16.54766221710000096, -100.0428544680000016, 2.640864489020000150 ) ) ;
#1171=AXIS2_PLACEMENT_3D ( 'NONE', #20331, #24861, #13775 ) ;
#1182=AXIS2_PLACEMENT_3D ( 'NONE', #13757, #17697, #2120 ) ;
#1188=CARTESIAN_POINT ( 'NONE',  ( -17.91520637925930615, -98.72564645249281057, 4.448055852924632347 ) ) ;
#1192=CARTESIAN_POINT ( 'NONE',  ( -5.983771968930000185, -101.2459394079999981, 14.78967057790000084 ) ) ;
#1195=CARTESIAN_POINT ( 'NONE',  ( -4.115583105835526112, -96.89152197809237066, -20.86381302798665160 ) ) ;
#1198=CARTESIAN_POINT ( 'NONE',  ( -13.01174968712481217, -101.6407018583229416, -9.320898687691189011 ) ) ;
#1204=CARTESIAN_POINT ( 'NONE',  ( -20.43643619460000238, -93.49011727610000833, 16.37406953600000037 ) ) ;
#1205=CARTESIAN_POINT ( 'NONE',  ( 16.79922297439999923, -99.53431386179998697, 4.586272525910000120 ) ) ;
#1208=CARTESIAN_POINT ( 'NONE',  ( 14.05983645159999895, -99.53431386179998697, -10.27466725399999881 ) ) ;
#1211=CARTESIAN_POINT ( 'NONE',  ( 7.102042752109999135, -101.6484611540000031, 14.33739825589999839 ) ) ;
#1213=CARTESIAN_POINT ( 'NONE',  ( 6.019093083229999586, -92.50000000000000000, 29.30685818879999971 ) ) ;
#1216=ADVANCED_FACE ( 'NONE', ( #13541 ), #4022, .F. ) ;
#1220=ORIENTED_EDGE ( 'NONE', *, *, #18993, .F. ) ;
#1229=DIRECTION ( 'NONE',  ( 0.000000000000000000, 1.000000000000000000, 0.000000000000000000 ) ) ;
#1230=ORIENTED_EDGE ( 'NONE', *, *, #13863, .F. ) ;
#1232=CARTESIAN_POINT ( 'NONE',  ( -23.87286787420000067, -93.96464232239999603, -7.079520382630000164 ) ) ;
#1238=DIRECTION ( 'NONE',  ( 0.000000000000000000, 1.000000000000000000, 0.000000000000000000 ) ) ;
#1240=DIRECTION ( 'NONE',  ( 0.000000000000000000, -1.000000000000000000, 0.000000000000000000 ) ) ;
#1242=DIRECTION ( 'NONE',  ( 0.3639667172450259391, 0.000000000000000000, -0.9314119543670669188 ) ) ;
#1250=CARTESIAN_POINT ( 'NONE',  ( -11.40589454009999848, -95.08268351149999376, -21.37599873950000173 ) ) ;
#1255=CARTESIAN_POINT ( 'NONE',  ( -18.58238019774981353, -93.25521310994808744, -21.15957345179030469 ) ) ;
#1262=ORIENTED_EDGE ( 'NONE', *, *, #8790, .F. ) ;
#1264=CARTESIAN_POINT ( 'NONE',  ( 0.3228164666304381702, -101.4085864806541650, -16.18225634051029971 ) ) ;
#1267=DIRECTION ( 'NONE',  ( 1.000000000000000000, 0.000000000000000000, 0.000000000000000000 ) ) ;
#1268=CARTESIAN_POINT ( 'NONE',  ( -8.209463884390000743, -99.53431386179998697, 15.35748973489999969 ) ) ;
#1270=CARTESIAN_POINT ( 'NONE',  ( 16.42966103859999905, -94.59276292389999696, 17.21499949629999904 ) ) ;
#1271=DIRECTION ( 'NONE',  ( 0.000000000000000000, -1.000000000000000000, 0.000000000000000000 ) ) ;
#1281=CARTESIAN_POINT ( 'NONE',  ( -28.19807706989999829, -92.76550115769998683, 1.645633876470000034 ) ) ;
#1288=EDGE_LOOP ( 'NONE', ( #18758, #28729, #17531 ) ) ;
#1292=CARTESIAN_POINT ( 'NONE',  ( -14.61698170120000029, -101.1363384779999990, 4.673707807969999628 ) ) ;
#1294=CARTESIAN_POINT ( 'NONE',  ( -15.04689636610000036, -101.1175442680000032, 3.135183322060000499 ) ) ;
#1298=ORIENTED_EDGE ( 'NONE', *, *, #3350, .F. ) ;
#1301=CARTESIAN_POINT ( 'NONE',  ( -7.728319723075819603, -100.8738282916487208, 14.69600823143309576 ) ) ;
#1307=ORIENTED_EDGE ( 'NONE', *, *, #295, .F. ) ;
#1308=EDGE_CURVE ( 'NONE', #23834, #22763, #12324, .T. ) ;
#1310=CARTESIAN_POINT ( 'NONE',  ( 6.719631698796779240, -100.6644468679725009, 15.36513027133983122 ) ) ;
#1312=EDGE_LOOP ( 'NONE', ( #4453, #28583, #27849, #15878 ) ) ;
#1314=CARTESIAN_POINT ( 'NONE',  ( 0.000000000000000000, -101.6484611540000031, 0.000000000000000000 ) ) ;
#1317=CARTESIAN_POINT ( 'NONE',  ( 27.46713810829999858, -92.96321833979999383, 9.765138773850001286 ) ) ;
#1318=CARTESIAN_POINT ( 'NONE',  ( -6.045971696259999639, -101.1411470200000053, 14.15183991680000020 ) ) ;
#1328=ORIENTED_EDGE ( 'NONE', *, *, #25383, .F. ) ;
#1329=CARTESIAN_POINT ( 'NONE',  ( -20.52527758500000132, -95.75647260690000451, -9.198302384599999826 ) ) ;
#1330=CARTESIAN_POINT ( 'NONE',  ( 9.017788245969780903, -92.49999918155076273, -27.43400824161624385 ) ) ;
#1332=CARTESIAN_POINT ( 'NONE',  ( 24.73701769899999903, -93.39359504719999450, -11.28691117220000173 ) ) ;
#1341=CARTESIAN_POINT ( 'NONE',  ( 21.94462607333390380, -96.36359510713519683, -0.1463646804548337788 ) ) ;
#1342=CARTESIAN_POINT ( 'NONE',  ( 23.96368475870000125, -101.1889999979999999, 8.717328305520000598 ) ) ;
#1344=DIRECTION ( 'NONE',  ( 1.000000000000000000, 0.000000000000000000, 0.000000000000000000 ) ) ;
#1350=CARTESIAN_POINT ( 'NONE',  ( -12.36495966000000024, -101.1848541609999899, -8.980491836739998845 ) ) ;
#1352=VECTOR ( 'NONE', #1229, 1000.000000000000000 ) ;
#1354=CARTESIAN_POINT ( 'NONE',  ( 1.673545578960000224, -92.65509162889999573, 27.65323681370000131 ) ) ;
#1358=CARTESIAN_POINT ( 'NONE',  ( 12.66014534235611322, -101.5526869446726153, -9.904007292906472415 ) ) ;
#1359=B_SPLINE_CURVE_WITH_KNOTS ( 'NONE', 3,
 ( #8352, #25446, #12573, #23258, #18890, #3301, #8085, #27772, #21077, #10386, #1138, #25724, #5755, #23538, #9975, #27907, #25588, #5615, #21486, #14496, #28185, #23397, #3439, #12304, #19022, #1544, #16835, #25864, #3575, #11089, #4426, #13297, #3992 ),
 .UNSPECIFIED., .F., .F.,
 ( 4, 2, 1, 1, 2, 2, 1, 1, 1, 2, 2, 2, 1, 1, 2, 2, 1, 1, 2, 2, 4 ),
 ( 0.000000000000000000, 0.06249999999986458055, 0.09374999999978507470, 0.1093749999997540440, 0.1171874999997460920, 0.1249999999997381261, 0.1874999999997520594, 0.2187499999997566669, 0.2343749999997590261, 0.2421874999997645772, 0.2499999999997701283, 0.3749999999998100964, 0.4374999999998272493, 0.4687499999998345768, 0.4843749999998410716, 0.4999999999998475664, 0.6249999999998780975, 0.6874999999998955280, 0.7187499999999057421, 0.7499999999999159561, 1.000000000000000000 ),
 .UNSPECIFIED. ) ;
#1362=CARTESIAN_POINT ( 'NONE',  ( 0.3059185938709999553, -93.00000000000000000, 14.72672055670000013 ) ) ;
#1366=CARTESIAN_POINT ( 'NONE',  ( 11.50679452860000040, -101.1848541609999899, -10.05659687459999851 ) ) ;
#1372=DIRECTION ( 'NONE',  ( 0.000000000000000000, -1.000000000000000000, 0.000000000000000000 ) ) ;
#1374=CARTESIAN_POINT ( 'NONE',  ( 0.002146109654809999837, -101.6311724339999927, -16.01369408300000075 ) ) ;
#1382=CIRCLE ( 'NONE', #17641, 5.000000000000000888 ) ;
#1384=CARTESIAN_POINT ( 'NONE',  ( 6.719470054089999422, -100.4650220110000021, 15.43601254670000067 ) ) ;
#1385=CARTESIAN_POINT ( 'NONE',  ( 15.64536997099999915, -101.3878691800000098, 3.811131059900000118 ) ) ;
#1387=CARTESIAN_POINT ( 'NONE',  ( -11.63405728910000114, -94.86303146849999735, -21.38493624129999660 ) ) ;
#1389=CARTESIAN_POINT ( 'NONE',  ( 5.376469156563769225, -92.59033770611050329, -30.02271131604222987 ) ) ;
#1390=CARTESIAN_POINT ( 'NONE',  ( -8.209474437350001708, -99.53431242750001218, 15.35746870819999899 ) ) ;
#1391=CARTESIAN_POINT ( 'NONE',  ( 8.067175576580000396, -93.91547326120000605, -23.40448531159999845 ) ) ;
#1393=ORIENTED_EDGE ( 'NONE', *, *, #27899, .F. ) ;
#1396=CARTESIAN_POINT ( 'NONE',  ( 6.114061450880000415, -111.0000000000000000, -13.40104985119999981 ) ) ;
#1399=ORIENTED_EDGE ( 'NONE', *, *, #11498, .F. ) ;
#1402=CARTESIAN_POINT ( 'NONE',  ( 0.3445358076898260014, -101.3846248973681838, -16.20041589813614280 ) ) ;
#1403=CARTESIAN_POINT ( 'NONE',  ( 6.018657797749999538, -100.4792519539999915, 15.03391506150000012 ) ) ;
#1406=EDGE_CURVE ( 'NONE', #18883, #9768, #15708, .T. ) ;
#1409=DIRECTION ( 'NONE',  ( 0.000000000000000000, 1.000000000000000000, 0.000000000000000000 ) ) ;
#1410=CARTESIAN_POINT ( 'NONE',  ( 24.33297166435627190, -93.99439547207676071, -9.447863160898569035 ) ) ;
#1415=ORIENTED_EDGE ( 'NONE', *, *, #25728, .T. ) ;
#1428=EDGE_CURVE ( 'NONE', #22101, #2397, #23522, .T. ) ;
#1432=AXIS2_PLACEMENT_3D ( 'NONE', #23804, #12705, #1805 ) ;
#1433=CARTESIAN_POINT ( 'NONE',  ( -22.25450259269999975, -94.89197151650000706, -8.089821617090001027 ) ) ;
#1437=CARTESIAN_POINT ( 'NONE',  ( 0.000000000000000000, -107.1975888269999899, 0.000000000000000000 ) ) ;
#1438=CARTESIAN_POINT ( 'NONE',  ( -14.34373124439999891, -92.50000000000000000, -26.25602392650000283 ) ) ;
#1439=ORIENTED_EDGE ( 'NONE', *, *, #13143, .F. ) ;
#1443=CARTESIAN_POINT ( 'NONE',  ( -7.681814765061617756, -100.9570234913570488, 14.64644060644491574 ) ) ;
#1446=DIRECTION ( 'NONE',  ( 0.000000000000000000, 1.000000000000000000, 0.000000000000000000 ) ) ;
#1450=CARTESIAN_POINT ( 'NONE',  ( 6.659152648053978218, -101.1248211537192958, 14.99462091354799220 ) ) ;
#1455=AXIS2_PLACEMENT_3D ( 'NONE', #12126, #21042, #8048 ) ;
#1458=CARTESIAN_POINT ( 'NONE',  ( 27.17390343950000187, -92.54807936089999032, 9.505859965289999991 ) ) ;
#1462=CARTESIAN_POINT ( 'NONE',  ( -3.292855076097166656, -97.38870237746982639, -20.36241341912896985 ) ) ;
#1466=CARTESIAN_POINT ( 'NONE',  ( 16.83483077069999823, -99.92967571559999840, 4.239603657359999112 ) ) ;
#1470=EDGE_CURVE ( 'NONE', #1149, #13839, #11901, .T. ) ;
#1471=CARTESIAN_POINT ( 'NONE',  ( 15.83524192907358596, -101.5839620086842956, 2.606923154417748467 ) ) ;
#1472=CARTESIAN_POINT ( 'NONE',  ( -20.27478635940000373, -94.70873263889998839, 12.26043739520000031 ) ) ;
#1473=CARTESIAN_POINT ( 'NONE',  ( 23.55422583189999841, -93.65023553250000532, -9.043238345449999827 ) ) ;
#1479=AXIS2_PLACEMENT_3D ( 'NONE', #19800, #8292, #21709 ) ;
#1480=CARTESIAN_POINT ( 'NONE',  ( -15.21246488650000117, -100.9405327639999967, 4.776672761669999545 ) ) ;
#1482=CARTESIAN_POINT ( 'NONE',  ( 20.52749306944123830, -97.43022994675339987, 1.376655802589148880 ) ) ;
#1485=FACE_OUTER_BOUND ( 'NONE', #1288, .T. ) ;
#1487=SHAPE_REPRESENTATION_RELATIONSHIP ( 'NONE' , 'NONE' ,  #10908, #15419 ) ;
#1488=VERTEX_POINT ( 'NONE', #20921 ) ;
#1496=CARTESIAN_POINT ( 'NONE',  ( -12.54641657280000011, -101.1292389600000092, -9.112281375189999366 ) ) ;
#1498=CARTESIAN_POINT ( 'NONE',  ( -7.903212057390000211, -99.83167681540000160, 15.42228797350000136 ) ) ;
#1500=CARTESIAN_POINT ( 'NONE',  ( -2.986711171310000079, -94.79581646409999962, 23.48470800579999818 ) ) ;
#1503=DIRECTION ( 'NONE',  ( 0.000000000000000000, -1.000000000000000000, 0.000000000000000000 ) ) ;
#1505=CARTESIAN_POINT ( 'NONE',  ( 12.88080974073147189, -101.3846248973631958, -9.831425157082634314 ) ) ;
#1506=PLANE ( 'NONE',  #14915 ) ;
#1507=CARTESIAN_POINT ( 'NONE',  ( -16.91430575710000284, -100.0771588430000065, 3.341621066080000091 ) ) ;
#1513=ORIENTED_EDGE ( 'NONE', *, *, #4915, .T. ) ;
#1514=CYLINDRICAL_SURFACE ( 'NONE', #7223, 18.64285714290000229 ) ;
#1520=ORIENTED_EDGE ( 'NONE', *, *, #196, .T. ) ;
#1521=CARTESIAN_POINT ( 'NONE',  ( 6.649881675840000561, -101.0405520670000072, 14.82396520390000028 ) ) ;
#1522=CARTESIAN_POINT ( 'NONE',  ( 15.60420274139999997, -101.2927714249999980, 3.777748170229999758 ) ) ;
#1525=CARTESIAN_POINT ( 'NONE',  ( 3.787197165510000296, -93.00000000000000000, -30.26395773239999798 ) ) ;
#1526=CARTESIAN_POINT ( 'NONE',  ( 3.355978770230000130, -90.50000000000000000, 6.143077933229999843 ) ) ;
#1528=CARTESIAN_POINT ( 'NONE',  ( 3.263855493430000365, -92.57423544259999915, -28.67967719789999848 ) ) ;
#1531=CARTESIAN_POINT ( 'NONE',  ( -1.869200974745226063, -93.63284908718598842, 25.01357699951009295 ) ) ;
#1533=CIRCLE ( 'NONE', #3842, 18.64285714289999873 ) ;
#1537=EDGE_CURVE ( 'NONE', #23472, #19113, #3292, .T. ) ;
#1540=ORIENTED_EDGE ( 'NONE', *, *, #12604, .F. ) ;
#1541=CARTESIAN_POINT ( 'NONE',  ( -0.7205257404120000153, -101.5369810359999860, -15.98376809940000065 ) ) ;
#1544=CARTESIAN_POINT ( 'NONE',  ( 13.83675081990681122, -92.54938211476543586, 27.18091423687219788 ) ) ;
#1548=VECTOR ( 'NONE', #13237, 1000.000000000000000 ) ;
#1552=CARTESIAN_POINT ( 'NONE',  ( 14.28941763439999946, -93.00000000000000000, -3.575252188409999921 ) ) ;
#1555=CIRCLE ( 'NONE', #27139, 15.19391340349999986 ) ;
#1561=DIRECTION ( 'NONE',  ( 0.000000000000000000, -1.000000000000000000, 0.000000000000000000 ) ) ;
#1564=ADVANCED_FACE ( 'NONE', ( #16388 ), #3011, .T. ) ;
#1565=CARTESIAN_POINT ( 'NONE',  ( 15.35943464070000175, -100.7833805400000102, 4.159771655669999291 ) ) ;
#1573=AXIS2_PLACEMENT_3D ( 'NONE', #13511, #6979, #438 ) ;
#1578=ORIENTED_EDGE ( 'NONE', *, *, #18993, .T. ) ;
#1579=CARTESIAN_POINT ( 'NONE',  ( 22.83659466689194062, -95.90275867365805595, -4.923095664741855337 ) ) ;
#1580=CARTESIAN_POINT ( 'NONE',  ( -11.69640386740000082, -101.0875971110000080, -10.03173011250000002 ) ) ;
#1582=CARTESIAN_POINT ( 'NONE',  ( -7.501065465934297016, -101.2145573445136222, 14.51273970916295752 ) ) ;
#1588=VERTEX_POINT ( 'NONE', #25714 ) ;
#1589=ADVANCED_FACE ( 'NONE', ( #13916 ), #28211, .T. ) ;
#1592=EDGE_CURVE ( 'NONE', #16528, #28629, #10836, .T. ) ;
#1593=DIRECTION ( 'NONE',  ( 0.000000000000000000, 1.000000000000000000, 0.000000000000000000 ) ) ;
#1597=DIRECTION ( 'NONE',  ( 0.000000000000000000, -1.000000000000000000, 0.000000000000000000 ) ) ;
#1605=CARTESIAN_POINT ( 'NONE',  ( -14.15498507100000047, -93.99830544900000007, -21.64661225829999935 ) ) ;
#1608=CARTESIAN_POINT ( 'NONE',  ( -18.71306389469999942, -96.65227117089999354, -10.09692839740000103 ) ) ;
#1609=CARTESIAN_POINT ( 'NONE',  ( 13.51933813770000015, -100.3517545579999961, -9.891026358559999565 ) ) ;
#1611=CARTESIAN_POINT ( 'NONE',  ( 23.80455697029999840, -93.92589062420000801, -8.153550017880000667 ) ) ;
#1616=VERTEX_POINT ( 'NONE', #15913 ) ;
#1620=CARTESIAN_POINT ( 'NONE',  ( 20.65093475452214022, -97.34036579196893513, 1.255409981387750173 ) ) ;
#1623=CARTESIAN_POINT ( 'NONE',  ( 29.11677867130000052, -92.50000000000000000, 6.880015861159999524 ) ) ;
#1629=ORIENTED_EDGE ( 'NONE', *, *, #14978, .T. ) ;
#1632=ORIENTED_EDGE ( 'NONE', *, *, #14850, .F. ) ;
#1634=CARTESIAN_POINT ( 'NONE',  ( -13.23436873610000042, -101.5317765570000006, -9.147552046289998628 ) ) ;
#1635=DIRECTION ( 'NONE',  ( 0.9863585068926603583, 0.000000000000000000, 0.1646113479699432003 ) ) ;
#1642=CYLINDRICAL_SURFACE ( 'NONE', #4136, 20.64285714289999163 ) ;
#1644=CARTESIAN_POINT ( 'NONE',  ( 12.60821841358252193, -101.5829753080987814, -9.932320047300365218 ) ) ;
#1645=DIRECTION ( 'NONE',  ( 0.000000000000000000, 1.000000000000000000, 0.000000000000000000 ) ) ;
#1647=CARTESIAN_POINT ( 'NONE',  ( 7.181689689069999716, -99.92967571559999840, 15.80535034289999885 ) ) ;
#1648=ORIENTED_EDGE ( 'NONE', *, *, #18541, .T. ) ;
#1653=CARTESIAN_POINT ( 'NONE',  ( -20.59421057834115842, -93.07145594888166329, 16.81328959876951856 ) ) ;
#1658=CARTESIAN_POINT ( 'NONE',  ( 15.76644911200000188, -101.6484611580000035, 2.726874312449999671 ) ) ;
#1662=CARTESIAN_POINT ( 'NONE',  ( 6.540410660740000104, -100.9364576079999978, 14.54829053200000111 ) ) ;
#1663=CARTESIAN_POINT ( 'NONE',  ( -15.61689027843468480, -92.57936004669802799, -24.03289022899482674 ) ) ;
#1664=ADVANCED_FACE ( 'NONE', ( #15461 ), #15415, .F. ) ;
#1669=CARTESIAN_POINT ( 'NONE',  ( 9.010434747179999704, -94.45168166339999516, -23.20781253819999890 ) ) ;
#1671=CARTESIAN_POINT ( 'NONE',  ( 6.954809927569434613, -101.6297509123136535, 14.42559876608666514 ) ) ;
#1672=CARTESIAN_POINT ( 'NONE',  ( 1.673548719218163061, -92.65509297688285528, 27.65323130849352395 ) ) ;
#1675=CARTESIAN_POINT ( 'NONE',  ( -12.73945486129048454, -100.6338045024292995, -10.94379842081711551 ) ) ;
#1676=ORIENTED_EDGE ( 'NONE', *, *, #12743, .T. ) ;
#1677=CARTESIAN_POINT ( 'NONE',  ( -1.283022169079999886, -101.3150705500000157, -16.20107500659999644 ) ) ;
#1678=DIRECTION ( 'NONE',  ( 1.000000000000000000, 0.000000000000000000, 0.000000000000000000 ) ) ;
#1679=B_SPLINE_CURVE_WITH_KNOTS ( 'NONE', 5,
 ( #23387, #16240, #20639, #25153, #20785, #1128, #14068, #12155, #695 ),
 .UNSPECIFIED., .F., .F.,
 ( 6, 3, 6 ),
 ( 0.000000000000000000, 0.5000000000000000000, 1.000000000000000000 ),
 .UNSPECIFIED. ) ;
#1681=CARTESIAN_POINT ( 'NONE',  ( 16.15437062272748037, -94.72386903546126291, 17.24227625337255176 ) ) ;
#1684=CARTESIAN_POINT ( 'NONE',  ( -15.39276618183619583, -101.4254873439999329, 4.250919977501043334 ) ) ;
#1688=DIRECTION ( 'NONE',  ( 0.000000000000000000, 1.000000000000000000, 0.000000000000000000 ) ) ;
#1690=DIRECTION ( 'NONE',  ( 1.000000000000000000, 0.000000000000000000, 0.000000000000000000 ) ) ;
#1693=ADVANCED_FACE ( 'NONE', ( #13878 ), #7601, .F. ) ;
#1694=ORIENTED_EDGE ( 'NONE', *, *, #22234, .F. ) ;
#1696=CARTESIAN_POINT ( 'NONE',  ( -29.44685991679999759, -92.54628605920001405, 6.396492330759999234 ) ) ;
#1700=VERTEX_POINT ( 'NONE', #25115 ) ;
#1707=CARTESIAN_POINT ( 'NONE',  ( -15.29947873360000088, -101.1716782170000073, 3.671501766180000459 ) ) ;
#1708=CARTESIAN_POINT ( 'NONE',  ( -22.00137621023848666, -95.57586223585661855, -5.105060933739808959 ) ) ;
#1710=VERTEX_POINT ( 'NONE', #9929 ) ;
#1712=CARTESIAN_POINT ( 'NONE',  ( -12.58639594889999991, -100.8746138070000029, -10.82789256390000077 ) ) ;
#1713=EDGE_CURVE ( 'NONE', #19059, #1149, #27914, .T. ) ;
#1715=VERTEX_POINT ( 'NONE', #25265 ) ;
#1717=CARTESIAN_POINT ( 'NONE',  ( -0.9302893022191279782, -101.6077248516953091, -16.00345022493254632 ) ) ;
#1720=ORIENTED_EDGE ( 'NONE', *, *, #25096, .T. ) ;
#1723=CARTESIAN_POINT ( 'NONE',  ( 6.669678980424931680, -101.2145573445209408, 14.91311433900129124 ) ) ;
#1725=EDGE_LOOP ( 'NONE', ( #14448, #4958, #14088, #20508 ) ) ;
#1726=CARTESIAN_POINT ( 'NONE',  ( -19.97841359259663463, -95.83493812764778852, 9.662536293482050453 ) ) ;
#1731=CARTESIAN_POINT ( 'NONE',  ( -3.236852559049167244, -97.42330309947865885, -20.32638677250028891 ) ) ;
#1733=EDGE_LOOP ( 'NONE', ( #13344, #12764, #17680, #18232 ) ) ;
#1736=CARTESIAN_POINT ( 'NONE',  ( -18.26810397560000254, -94.98812477769999418, 16.32728546869999775 ) ) ;
#1739=CARTESIAN_POINT ( 'NONE',  ( 12.67716433170000023, -100.8815367389999977, -9.218731588149999823 ) ) ;
#1743=CARTESIAN_POINT ( 'NONE',  ( 29.90142803373326430, -92.53260370668940027, 6.013043342471341646 ) ) ;
#1751=CARTESIAN_POINT ( 'NONE',  ( 0.04581334808960710325, -92.83865970263813949, -30.49996578665741964 ) ) ;
#1754=AXIS2_PLACEMENT_3D ( 'NONE', #18412, #27301, #9794 ) ;
#1764=CARTESIAN_POINT ( 'NONE',  ( -13.00841234930000034, -100.9763228559999959, -8.758810206009998822 ) ) ;
#1765=B_SPLINE_SURFACE_WITH_KNOTS ( 'NONE', 5, 5, ( 
 ( #27754, #27623, #7793, #23237, #978, #18727, #20772, #16084, #5018 ),
 ( #24985, #13907, #25428, #20624, #12140, #27474, #5458, #7520, #14341 ),
 ( #5321, #16664, #3284, #9531, #25562, #14478, #18433, #27322, #25291 ),
 ( #7363, #16226, #3142, #25140, #14209, #14054, #3003, #23101, #11998 ),
 ( #28030, #12832, #19003, #7928, #25848, #17377, #26270, #6292, #4108 ),
 ( #3692, #15159, #28294, #27883, #1662, #14748, #10365, #19279, #12554 ),
 ( #24068, #17085, #1521, #21744, #28167, #16812, #5735, #1793, #23933 ),
 ( #8066, #16957, #12979, #14619, #21891, #3972, #19138, #3831, #8328 ),
 ( #25708, #1384, #5869, #8199, #10500, #19414, #23649, #21466, #25978 ),
 ( #6004, #14884, #26121, #10639, #10085, #12411, #23520, #8475, #23793 ),
 ( #19551, #12693, #17230, #21607, #3556, #21325, #10227, #6149, #15019 ),
 ( #28440, #2524, #15903, #24662, #4693, #9193, #15301, #27001, #348 ) ),
 .UNSPECIFIED., .F., .F., .F.,
 ( 6, 3, 3, 6 ),
 ( 6, 3, 6 ),
 ( 0.8942436407639999807, 1.876087175710000166, 3.176036816339999902, 5.425307607549999744 ),
 ( 0.000000000000000000, 0.2500000000000000000, 0.5000000000000000000 ),
 .UNSPECIFIED. ) ;
#1767=CARTESIAN_POINT ( 'NONE',  ( 8.185346967789998374, -101.1889999979999999, 14.03998109830000018 ) ) ;
#1770=CARTESIAN_POINT ( 'NONE',  ( -29.74546239500669031, -92.83865970263998690, 6.742216160683305759 ) ) ;
#1774=CARTESIAN_POINT ( 'NONE',  ( 13.62782804938226100, -100.4211561362012333, -10.10291547818408908 ) ) ;
#1777=CARTESIAN_POINT ( 'NONE',  ( -15.69013080879999933, -101.5700432450000079, 3.430602099230000146 ) ) ;
#1778=ORIENTED_EDGE ( 'NONE', *, *, #20203, .T. ) ;
#1784=ADVANCED_FACE ( 'NONE', ( #5432 ), #27992, .T. ) ;
#1787=CARTESIAN_POINT ( 'NONE',  ( -0.1068060827170000116, -101.3256027139999986, -15.90648277770000085 ) ) ;
#1789=CARTESIAN_POINT ( 'NONE',  ( 14.95019707159999989, -101.2530993000000024, 2.710463435300000334 ) ) ;
#1792=ORIENTED_EDGE ( 'NONE', *, *, #3223, .F. ) ;
#1793=CARTESIAN_POINT ( 'NONE',  ( 6.130772363030000172, -100.7776802639999971, 14.57128679989999931 ) ) ;
#1794=CARTESIAN_POINT ( 'NONE',  ( 15.61826386989999982, -101.5964542560000012, 3.655520785480000256 ) ) ;
#1796=AXIS2_PLACEMENT_3D ( 'NONE', #16588, #449, #9298 ) ;
#1799=CARTESIAN_POINT ( 'NONE',  ( 4.060520888432426645, -92.92035259772417533, -30.22975431335808594 ) ) ;
#1803=CARTESIAN_POINT ( 'NONE',  ( 6.508840722400000445, -93.07154530319999708, -26.20378082560000266 ) ) ;
#1804=ADVANCED_FACE ( 'NONE', ( #10471 ), #5652, .T. ) ;
#1805=DIRECTION ( 'NONE',  ( 1.000000000000000000, 0.000000000000000000, 0.000000000000000000 ) ) ;
#1806=CARTESIAN_POINT ( 'NONE',  ( -6.863006950479999979, -101.6484611540000031, 14.45362438769999969 ) ) ;
#1807=ORIENTED_EDGE ( 'NONE', *, *, #16120, .T. ) ;
#1811=CARTESIAN_POINT ( 'NONE',  ( 25.50885178510000273, -93.36531860459999166, -5.860088577239999985 ) ) ;
#1812=CARTESIAN_POINT ( 'NONE',  ( -1.303833584549999980, -101.1364147039999892, -15.29041300709999796 ) ) ;
#1821=EDGE_CURVE ( 'NONE', #15112, #10772, #1555, .T. ) ;
#1822=CARTESIAN_POINT ( 'NONE',  ( 0.000000000000000000, -94.59276292389999696, 0.000000000000000000 ) ) ;
#1831=EDGE_CURVE ( 'NONE', #6421, #3937, #6162, .T. ) ;
#1836=CARTESIAN_POINT ( 'NONE',  ( -25.52588841249999874, -93.67384740769999496, -2.372690985960000276 ) ) ;
#1841=CARTESIAN_POINT ( 'NONE',  ( 15.73597609990000024, -101.0405520670000072, 4.043504278899999527 ) ) ;
#1844=CARTESIAN_POINT ( 'NONE',  ( -13.14229048259999999, -100.8869813350000015, -8.528548640909999534 ) ) ;
#1845=ORIENTED_EDGE ( 'NONE', *, *, #10335, .T. ) ;
#1850=B_SPLINE_CURVE_WITH_KNOTS ( 'NONE', 5,
 ( #10509, #3704, #1672, #1953, #1531, #10376 ),
 .UNSPECIFIED., .F., .F.,
 ( 6, 6 ),
 ( 0.000000000000000000, 1.000000000000000000 ),
 .UNSPECIFIED. ) ;
#1851=EDGE_CURVE ( 'NONE', #17518, #1013, #13144, .T. ) ;
#1858=CARTESIAN_POINT ( 'NONE',  ( -12.49636764419999935, -101.4908759489999994, -10.04157132919999995 ) ) ;
#1859=CARTESIAN_POINT ( 'NONE',  ( -29.71161737690000137, -93.00000000000000000, 6.352311025380000586 ) ) ;
#1860=ORIENTED_EDGE ( 'NONE', *, *, #26039, .T. ) ;
#1861=AXIS2_PLACEMENT_3D ( 'NONE', #17056, #5971, #17345 ) ;
#1862=CIRCLE ( 'NONE', #27464, 0.8000000000000003775 ) ;
#1863=CARTESIAN_POINT ( 'NONE',  ( -0.9821106753968790182, -101.5839620086842814, -16.01831432786889664 ) ) ;
#1867=CARTESIAN_POINT ( 'NONE',  ( -5.390285367900000679, -100.8869813350000015, 14.71056643040000012 ) ) ;
#1870=CARTESIAN_POINT ( 'NONE',  ( -19.26625410581794995, -97.04909278841957132, 7.359652529508150742 ) ) ;
#1873=CARTESIAN_POINT ( 'NONE',  ( -15.43525743989999910, -101.1461852590000063, 4.782895807790000120 ) ) ;
#1882=CARTESIAN_POINT ( 'NONE',  ( -14.42556421679999978, -92.50000000000000000, -2.978755036369999942 ) ) ;
#1885=CARTESIAN_POINT ( 'NONE',  ( -18.77234060500000012, -92.65715406920001840, -20.69363841459999875 ) ) ;
#1886=CARTESIAN_POINT ( 'NONE',  ( -15.94434063720000161, -93.10431551199999944, 24.00277150759999856 ) ) ;
#1887=ORIENTED_EDGE ( 'NONE', *, *, #6683, .T. ) ;
#1888=EDGE_CURVE ( 'NONE', #4529, #22228, #12584, .T. ) ;
#1889=CARTESIAN_POINT ( 'NONE',  ( 12.67342850500000040, -100.8685038539999965, -9.320488510950001526 ) ) ;
#1892=CARTESIAN_POINT ( 'NONE',  ( 29.91164248172746198, -92.52640451552758805, 5.961874894218010645 ) ) ;
#1896=FACE_OUTER_BOUND ( 'NONE', #24576, .T. ) ;
#1897=CARTESIAN_POINT ( 'NONE',  ( -24.56259648705387022, -92.50000000000000000, -18.08169719992735480 ) ) ;
#1899=CARTESIAN_POINT ( 'NONE',  ( 0.03433565797716789381, -92.82709422631805296, -30.49998078697906578 ) ) ;
#1905=CARTESIAN_POINT ( 'NONE',  ( 17.67606731260000075, -99.62155223519999936, 1.124352996140000061 ) ) ;
#1910=CARTESIAN_POINT ( 'NONE',  ( 14.91172220540000026, -95.31428172910000285, 17.37540928339999979 ) ) ;
#1913=DIRECTION ( 'NONE',  ( 1.000000000000000000, 0.000000000000000000, 0.000000000000000000 ) ) ;
#1928=CARTESIAN_POINT ( 'NONE',  ( 10.17429874589999983, -95.72998414199999218, -19.97250627529999889 ) ) ;
#1931=CARTESIAN_POINT ( 'NONE',  ( -17.06129450210000087, -93.25667418180000823, 21.77310057969999946 ) ) ;
#1932=CARTESIAN_POINT ( 'NONE',  ( 12.01015229399999917, -101.6484611540000031, -9.798277495349999811 ) ) ;
#1935=CARTESIAN_POINT ( 'NONE',  ( 0.6434015132710000362, -100.4650220110000021, -16.82283554099999989 ) ) ;
#1940=EDGE_LOOP ( 'NONE', ( #1439, #20708, #6249, #12128, #12080 ) ) ;
#1942=CARTESIAN_POINT ( 'NONE',  ( 15.52117313229999951, -101.2902355740000075, 3.579205768200000026 ) ) ;
#1950=CARTESIAN_POINT ( 'NONE',  ( 3.404243284160000105, -93.04780269100000112, -28.95354108839999796 ) ) ;
#1953=CARTESIAN_POINT ( 'NONE',  ( -0.2283525300826651505, -93.01584921915402049, 26.42460210401236154 ) ) ;
#1956=CARTESIAN_POINT ( 'NONE',  ( -13.25237707705474399, -99.99762666416590662, -11.12887180797588194 ) ) ;
#1959=CARTESIAN_POINT ( 'NONE',  ( 25.60466699379999866, -93.13207089229999269, -5.766591832619999636 ) ) ;
#1961=CARTESIAN_POINT ( 'NONE',  ( -1.526197323679999940, -100.8869817940000075, -15.59251925729999932 ) ) ;
#1968=CARTESIAN_POINT ( 'NONE',  ( -14.58939485729999852, -101.2530991829999891, 4.248445246460000213 ) ) ;
#1969=CIRCLE ( 'NONE', #18251, 20.64285714289999873 ) ;
#1972=CARTESIAN_POINT ( 'NONE',  ( 13.78283651632031770, -100.0559847774664775, -10.38643546923515970 ) ) ;
#1974=( NAMED_UNIT ( * ) SI_UNIT ( $, .STERADIAN. ) SOLID_ANGLE_UNIT ( ) );
#1983=CARTESIAN_POINT ( 'NONE',  ( -18.88944331899999796, -101.1889999979999999, -23.13319212550000259 ) ) ;
#1987=EDGE_CURVE ( 'NONE', #10101, #14792, #11184, .T. ) ;
#1999=CARTESIAN_POINT ( 'NONE',  ( -17.58226716778080956, -94.81956704558760407, 15.60250440155592422 ) ) ;
#2001=AXIS2_PLACEMENT_3D ( 'NONE', #9830, #16390, #18737 ) ;
#2004=CARTESIAN_POINT ( 'NONE',  ( -11.86297998370000073, -101.1402801299999936, -9.726116368819999636 ) ) ;
#2013=AXIS2_PLACEMENT_3D ( 'NONE', #7891, #16770, #5693 ) ;
#2017=ORIENTED_EDGE ( 'NONE', *, *, #11344, .F. ) ;
#2019=CARTESIAN_POINT ( 'NONE',  ( -19.74515506783779628, -96.28273967183713467, 8.793340612910874654 ) ) ;
#2020=VERTEX_POINT ( 'NONE', #2939 ) ;
#2021=CARTESIAN_POINT ( 'NONE',  ( 22.10956385849999961, -93.90388243319999617, 13.35155070529999932 ) ) ;
#2027=CARTESIAN_POINT ( 'NONE',  ( 11.99447238389999981, -101.1411470200000053, -9.642266023979999545 ) ) ;
#2028=CARTESIAN_POINT ( 'NONE',  ( -20.38769392570000250, -92.57423544259999915, -20.43327123240000276 ) ) ;
#2032=CARTESIAN_POINT ( 'NONE',  ( 13.24160441829999968, -100.4808658609999981, -9.370009802470001148 ) ) ;
#2040=DIRECTION ( 'NONE',  ( 1.000000000000000000, 0.000000000000000000, 0.000000000000000000 ) ) ;
#2043=CARTESIAN_POINT ( 'NONE',  ( -0.1264782718447538534, -92.71619979444359672, -30.49973804731671478 ) ) ;
#2044=DIRECTION ( 'NONE',  ( 0.000000000000000000, -1.000000000000000000, 0.000000000000000000 ) ) ;
#2053=CARTESIAN_POINT ( 'NONE',  ( 15.58784585939999978, -100.8733984769999950, 2.070707821839999685 ) ) ;
#2059=CARTESIAN_POINT ( 'NONE',  ( 15.98190517250000120, -101.1461874320000049, 2.387865266659999985 ) ) ;
#2061=ORIENTED_EDGE ( 'NONE', *, *, #5282, .T. ) ;
#2062=CARTESIAN_POINT ( 'NONE',  ( -0.7543003842240000312, -111.0000000000000000, -16.73300722909999649 ) ) ;
#2063=CARTESIAN_POINT ( 'NONE',  ( 7.844113379649998663, -101.1184174639999895, 13.21637662110000022 ) ) ;
#2064=CARTESIAN_POINT ( 'NONE',  ( 1.375225265779999928, -94.98812079580000045, 24.46248543800000164 ) ) ;
#2066=CIRCLE ( 'NONE', #26248, 4.999999999999999112 ) ;
#2067=CARTESIAN_POINT ( 'NONE',  ( -29.70880753679850628, -92.72059904818995335, 6.901939759926293938 ) ) ;
#2069=ORIENTED_EDGE ( 'NONE', *, *, #6148, .T. ) ;
#2070=DIRECTION ( 'NONE',  ( 1.000000000000000000, 0.000000000000000000, 0.000000000000000000 ) ) ;
#2074=ORIENTED_EDGE ( 'NONE', *, *, #13986, .F. ) ;
#2077=CARTESIAN_POINT ( 'NONE',  ( -15.25169713729999899, -93.03108158919999937, 25.12655145109999921 ) ) ;
#2078=CARTESIAN_POINT ( 'NONE',  ( -19.16019836899999618, -92.50000000000000000, 22.97842938279999814 ) ) ;
#2081=AXIS2_PLACEMENT_3D ( 'NONE', #17645, #14108, #20674 ) ;
#2082=CARTESIAN_POINT ( 'NONE',  ( 0.8390948241760000093, -99.74726900420000675, -17.13497999810000039 ) ) ;
#2093=ORIENTED_EDGE ( 'NONE', *, *, #3385, .T. ) ;
#2094=CARTESIAN_POINT ( 'NONE',  ( 28.18364776602151167, -92.64884742710839305, 11.65904703969763112 ) ) ;
#2095=CARTESIAN_POINT ( 'NONE',  ( 15.29251030651879439, -101.1416252791453019, 2.772524658013501675 ) ) ;
#2099=CARTESIAN_POINT ( 'NONE',  ( -1.469243280769999993, -101.0356131030000029, -15.40539586329999899 ) ) ;
#2104=CARTESIAN_POINT ( 'NONE',  ( -6.665307709260000379, -111.0000000000000000, -13.13558364449999871 ) ) ;
#2105=ORIENTED_EDGE ( 'NONE', *, *, #8436, .T. ) ;
#2108=EDGE_LOOP ( 'NONE', ( #25166, #6629, #28009, #13082 ) ) ;
#2109=CARTESIAN_POINT ( 'NONE',  ( -0.8337756410959999975, -101.5369810359999860, -15.97866295649999913 ) ) ;
#2113=CARTESIAN_POINT ( 'NONE',  ( -20.66056017707865422, -92.75430643271349140, -22.43644101044492700 ) ) ;
#2114=DIRECTION ( 'NONE',  ( 0.000000000000000000, -1.000000000000000000, 0.000000000000000000 ) ) ;
#2120=DIRECTION ( 'NONE',  ( 0.2287893768880238932, 0.000000000000000000, -0.9734759478401044941 ) ) ;
#2121=CARTESIAN_POINT ( 'NONE',  ( 26.51311248191242242, -93.18010901228015541, 10.50323123315586926 ) ) ;
#2123=ADVANCED_FACE ( 'NONE', ( #915 ), #19653, .F. ) ;
#2128=CARTESIAN_POINT ( 'NONE',  ( -25.71305159770000159, -93.90388142500000868, -2.436348821509999762 ) ) ;
#2132=CYLINDRICAL_SURFACE ( 'NONE', #20604, 0.7999999999999994893 ) ;
#2139=CARTESIAN_POINT ( 'NONE',  ( 24.45765515529999945, -92.57423544259999915, -15.32970127379999958 ) ) ;
#2142=CARTESIAN_POINT ( 'NONE',  ( -16.17553334493379324, -99.16532134656523567, 7.643797697565219096 ) ) ;
#2145=CARTESIAN_POINT ( 'NONE',  ( -12.83089869019999973, -99.70407914540000149, -11.44895565849999919 ) ) ;
#2149=EDGE_CURVE ( 'NONE', #22535, #22268, #465, .T. ) ;
#2152=DIRECTION ( 'NONE',  ( 0.000000000000000000, 1.000000000000000000, 0.000000000000000000 ) ) ;
#2155=B_SPLINE_CURVE_WITH_KNOTS ( 'NONE', 3,
 ( #24777, #18659, #763, #20704, #9313, #20844, #18508, #7452, #18803, #906, #27402, #16309, #20396, #27256, #20550, #12076, #20987, #5250, #25222, #1051, #7595, #27695, #25069, #2640, #18217, #9749, #7152, #25366, #18369, #9463, #22596, #27555, #22741, #14275, #16019, #4954, #7293 ),
 .UNSPECIFIED., .F., .F.,
 ( 4, 2, 2, 1, 1, 1, 2, 2, 2, 2, 1, 1, 1, 2, 2, 2, 2, 1, 1, 1, 2, 2, 4 ),
 ( 0.000000000000000000, 0.1250000000000014988, 0.1875000000000017208, 0.2187500000000023592, 0.2343750000000030254, 0.2421875000000027478, 0.2460937500000026368, 0.2500000000000025535, 0.3750000000000048850, 0.4375000000000060507, 0.4687500000000068834, 0.4843750000000068834, 0.4921875000000064948, 0.4960937500000062172, 0.5000000000000058842, 0.6250000000000046629, 0.6875000000000043299, 0.7187500000000041078, 0.7343750000000041078, 0.7421875000000041078, 0.7460937500000042188, 0.7500000000000042188, 1.000000000000000000 ),
 .UNSPECIFIED. ) ;
#2160=ORIENTED_EDGE ( 'NONE', *, *, #19790, .T. ) ;
#2161=CARTESIAN_POINT ( 'NONE',  ( -12.72359307473547219, -94.60934249415720387, -21.54967800148987678 ) ) ;
#2163=CARTESIAN_POINT ( 'NONE',  ( 26.11960070690000180, -92.76550138599999684, 10.75202456979999965 ) ) ;
#2168=EDGE_CURVE ( 'NONE', #7960, #3430, #17453, .T. ) ;
#2169=CARTESIAN_POINT ( 'NONE',  ( 12.50568558790000040, -101.5216621940000152, -9.997196710569999922 ) ) ;
#2170=CARTESIAN_POINT ( 'NONE',  ( -16.48967954220000109, -93.30149055190000240, -21.58637184819999888 ) ) ;
#2174=CARTESIAN_POINT ( 'NONE',  ( 13.26576849039999928, -100.7430069139999915, -9.799237773789998940 ) ) ;
#2176=CARTESIAN_POINT ( 'NONE',  ( -1.283023294879999998, -101.3150694429999987, -16.20107482390000087 ) ) ;
#2180=ORIENTED_EDGE ( 'NONE', *, *, #17837, .T. ) ;
#2183=CARTESIAN_POINT ( 'NONE',  ( -24.33129403500096899, -92.53260370680638403, -18.39130825355575638 ) ) ;
#2185=CARTESIAN_POINT ( 'NONE',  ( 23.70295537799999863, -94.59276292389999696, -2.111841813949999924 ) ) ;
#2191=CARTESIAN_POINT ( 'NONE',  ( 22.56413522780000136, -95.98460637690000397, -4.313985318640000344 ) ) ;
#2192=ORIENTED_EDGE ( 'NONE', *, *, #27398, .F. ) ;
#2196=CARTESIAN_POINT ( 'NONE',  ( 0.000000000000000000, -101.2530993010000060, 0.000000000000000000 ) ) ;
#2198=CARTESIAN_POINT ( 'NONE',  ( -6.602758024369999923, -97.12465307349999932, -19.67811079650000039 ) ) ;
#2200=CARTESIAN_POINT ( 'NONE',  ( 0.000000000000000000, -92.50000000000000000, 0.000000000000000000 ) ) ;
#2202=CARTESIAN_POINT ( 'NONE',  ( -29.63153379720834835, -92.59735406124617896, 7.226533350539707357 ) ) ;
#2203=CARTESIAN_POINT ( 'NONE',  ( 11.16696848683634435, -96.92941680577980890, -18.97929024651338636 ) ) ;
#2205=CARTESIAN_POINT ( 'NONE',  ( 11.56003560810000153, -93.05538536839999608, -23.65426206159999722 ) ) ;
#2208=CARTESIAN_POINT ( 'NONE',  ( -13.24302487323487476, -92.80442066020155778, 27.47494743563386521 ) ) ;
#2212=CARTESIAN_POINT ( 'NONE',  ( -15.94434063720000161, -93.10431551199999944, 24.00277150759999856 ) ) ;
#2213=DIRECTION ( 'NONE',  ( -0.000000000000000000, 1.000000000000000000, 0.000000000000000000 ) ) ;
#2217=CARTESIAN_POINT ( 'NONE',  ( 0.6447269329300000518, -100.1981337080000003, -16.97091045379999841 ) ) ;
#2225=CARTESIAN_POINT ( 'NONE',  ( 28.29231644507293453, -92.71525149892931950, 11.39321545286071924 ) ) ;
#2230=CARTESIAN_POINT ( 'NONE',  ( 18.47239823780000023, -94.07620464520000780, 16.72834433539999921 ) ) ;
#2232=CARTESIAN_POINT ( 'NONE',  ( 8.831064126840001194, -94.59276292389999696, -22.09756266850000017 ) ) ;
#2235=CARTESIAN_POINT ( 'NONE',  ( -12.88998090559132237, -100.4103893717285843, -11.04208011740792372 ) ) ;
#2239=ORIENTED_EDGE ( 'NONE', *, *, #14703, .T. ) ;
#2244=CARTESIAN_POINT ( 'NONE',  ( -0.7858244733099999380, -98.73889367950000917, -18.62175195770000258 ) ) ;
#2245=CARTESIAN_POINT ( 'NONE',  ( -20.54716539860091373, -92.71525149962195655, -22.54050847398934465 ) ) ;
#2246=CIRCLE ( 'NONE', #16659, 0.5000000000000011102 ) ;
#2248=CARTESIAN_POINT ( 'NONE',  ( 11.23715774159999903, -101.0848057460000007, -10.54863848640000157 ) ) ;
#2250=CARTESIAN_POINT ( 'NONE',  ( 16.31604581177785107, -94.64681100434714267, 17.22669056164060208 ) ) ;
#2251=EDGE_CURVE ( 'NONE', #11541, #1710, #15941, .T. ) ;
#2257=CARTESIAN_POINT ( 'NONE',  ( 24.06168706167060378, -93.59825775224986444, 12.30305419896300556 ) ) ;
#2262=CARTESIAN_POINT ( 'NONE',  ( 7.648936895900000366, -101.0907558640000019, 13.53920073169999938 ) ) ;
#2263=ORIENTED_EDGE ( 'NONE', *, *, #91, .T. ) ;
#2267=CARTESIAN_POINT ( 'NONE',  ( -24.56918193900000347, -94.36515553540000667, -3.609259138410000123 ) ) ;
#2273=FACE_OUTER_BOUND ( 'NONE', #27962, .T. ) ;
#2283=CARTESIAN_POINT ( 'NONE',  ( 24.35204445910000004, -92.65715406910000240, -13.69691108600000184 ) ) ;
#2287=CARTESIAN_POINT ( 'NONE',  ( -16.63477714874928637, -98.43098968254284387, 8.842934460737525981 ) ) ;
#2288=ORIENTED_EDGE ( 'NONE', *, *, #12233, .T. ) ;
#2296=CARTESIAN_POINT ( 'NONE',  ( 26.02259374959999860, -93.00000000000000000, -15.90831903569999994 ) ) ;
#2301=CARTESIAN_POINT ( 'NONE',  ( -5.854055351700000465, -101.0685845459999967, 14.98984499340000198 ) ) ;
#2303=ORIENTED_EDGE ( 'NONE', *, *, #25496, .T. ) ;
#2305=CARTESIAN_POINT ( 'NONE',  ( -26.00297803286303377, -94.00303307101484052, -2.070463084450466784 ) ) ;
#2306=CARTESIAN_POINT ( 'NONE',  ( 20.66588605339999773, -94.54647057319999703, 13.95977755230000028 ) ) ;
#2308=ORIENTED_EDGE ( 'NONE', *, *, #28313, .F. ) ;
#2310=CARTESIAN_POINT ( 'NONE',  ( -26.59500499809594487, -93.33134965528456917, -4.495659578470679207 ) ) ;
#2314=CARTESIAN_POINT ( 'NONE',  ( 26.75649127029999619, -111.0000000000000000, -13.26822602019999842 ) ) ;
#2316=AXIS2_PLACEMENT_3D ( 'NONE', #27762, #16822, #19287 ) ;
#2317=EDGE_CURVE ( 'NONE', #11679, #11057, #9819, .T. ) ;
#2319=CARTESIAN_POINT ( 'NONE',  ( 13.92892647020000041, -99.61736775859999682, -10.33597118630000011 ) ) ;
#2322=CARTESIAN_POINT ( 'NONE',  ( -5.701030053896644745, -98.22875432232922321, -19.45415947712940863 ) ) ;
#2323=FACE_OUTER_BOUND ( 'NONE', #5466, .T. ) ;
#2324=DIRECTION ( 'NONE',  ( 0.000000000000000000, 1.000000000000000000, 0.000000000000000000 ) ) ;
#2328=DIRECTION ( 'NONE',  ( -0.000000000000000000, 1.000000000000000000, 0.000000000000000000 ) ) ;
#2329=CARTESIAN_POINT ( 'NONE',  ( 0.000000000000000000, -92.50000000000000000, 0.000000000000000000 ) ) ;
#2332=CARTESIAN_POINT ( 'NONE',  ( -14.66822218795144295, -101.0767042429054641, 4.761812676672435352 ) ) ;
#2334=PRODUCT_CONTEXT ( 'NONE', #18916, 'mechanical' ) ;
#2336=CIRCLE ( 'NONE', #7484, 15.19391340349999986 ) ;
#2341=CARTESIAN_POINT ( 'NONE',  ( 19.21071510300000185, -98.24302442670000346, -0.5565603496329999400 ) ) ;
#2348=CARTESIAN_POINT ( 'NONE',  ( -6.605171516649999575, -97.48426834619999681, -20.14546412150000165 ) ) ;
#2349=CARTESIAN_POINT ( 'NONE',  ( 7.904069757880235692, -94.04667188340653183, -24.76727834805952710 ) ) ;
#2350=CARTESIAN_POINT ( 'NONE',  ( -24.06374496360000137, -94.22763312380000400, -3.197736329870000116 ) ) ;
#2351=CARTESIAN_POINT ( 'NONE',  ( -17.98004918629999693, -98.73884893519999650, 4.909944750820000259 ) ) ;
#2352=CARTESIAN_POINT ( 'NONE',  ( -29.57839868347437218, -92.54938211478190624, 7.441512166611892631 ) ) ;
#2357=CARTESIAN_POINT ( 'NONE',  ( -12.78325572749593064, -92.58608763741581527, 27.69184823660511796 ) ) ;
#2362=PLANE ( 'NONE',  #14051 ) ;
#2363=ORIENTED_EDGE ( 'NONE', *, *, #27219, .F. ) ;
#2367=CARTESIAN_POINT ( 'NONE',  ( 0.3813996810959999761, -101.2251655520000071, -16.21856860389999966 ) ) ;
#2368=DIRECTION ( 'NONE',  ( 0.6184463001828860440, 0.000000000000000000, 0.7858270635388550085 ) ) ;
#2373=DIRECTION ( 'NONE',  ( 0.9763395129702659991, 0.000000000000000000, -0.2162432783070585007 ) ) ;
#2376=CARTESIAN_POINT ( 'NONE',  ( 28.56828035858709924, -92.92035259817281201, 10.68546831372889550 ) ) ;
#2378=CARTESIAN_POINT ( 'NONE',  ( 8.071146758930000331, -100.8816832290000036, 13.57632735329999996 ) ) ;
#2381=CARTESIAN_POINT ( 'NONE',  ( 23.28812738402805138, -92.52249206702278173, -19.69551804736990874 ) ) ;
#2382=CARTESIAN_POINT ( 'NONE',  ( 24.73953705929999813, -92.49999846069999876, 14.89634059649999998 ) ) ;
#2386=CARTESIAN_POINT ( 'NONE',  ( -7.315719113890000180, -101.0640712160000021, 14.34151901279999919 ) ) ;
#2387=ORIENTED_EDGE ( 'NONE', *, *, #2852, .F. ) ;
#2393=CARTESIAN_POINT ( 'NONE',  ( 8.257819997060000361, -98.83157882129999905, 16.36072119760000021 ) ) ;
#2394=DIRECTION ( 'NONE',  ( 1.000000000000000000, 0.000000000000000000, 0.000000000000000000 ) ) ;
#2395=CARTESIAN_POINT ( 'NONE',  ( -2.330049844439999962, -97.93128678269999909, -19.86603722859999976 ) ) ;
#2397=VERTEX_POINT ( 'NONE', #26936 ) ;
#2399=CARTESIAN_POINT ( 'NONE',  ( -18.67420757599678893, -98.28141828938548485, -7.711871447694185200 ) ) ;
#2403=DIRECTION ( 'NONE',  ( 1.000000000000000000, 0.000000000000000000, 0.000000000000000000 ) ) ;
#2409=CIRCLE ( 'NONE', #13490, 5.000000000000000888 ) ;
#2411=CARTESIAN_POINT ( 'NONE',  ( 7.962341111249999770, -101.1573270909999991, 13.90182050930000024 ) ) ;
#2418=DIRECTION ( 'NONE',  ( 0.000000000000000000, 1.000000000000000000, 0.000000000000000000 ) ) ;
#2419=DIRECTION ( 'NONE',  ( 1.000000000000000000, 0.000000000000000000, 0.000000000000000000 ) ) ;
#2420=ADVANCED_FACE ( 'NONE', ( #9284 ), #18720, .F. ) ;
#2438=CARTESIAN_POINT ( 'NONE',  ( 14.05983683630000058, -99.53431242750001218, -10.27464373080000115 ) ) ;
#2440=ORIENTED_EDGE ( 'NONE', *, *, #13450, .F. ) ;
#2443=CARTESIAN_POINT ( 'NONE',  ( -12.82129959709999945, -100.1459902240000019, -11.09448884939999935 ) ) ;
#2451=B_SPLINE_CURVE_WITH_KNOTS ( 'NONE', 5,
 ( #16029, #24934, #4963, #22751, #20558, #627 ),
 .UNSPECIFIED., .F., .F.,
 ( 6, 6 ),
 ( 0.000000000000000000, 1.000000000000000000 ),
 .UNSPECIFIED. ) ;
#2452=ADVANCED_FACE ( 'NONE', ( #2610 ), #3361, .F. ) ;
#2453=CARTESIAN_POINT ( 'NONE',  ( -0.1868532263790000092, -111.0000000000000000, -16.79896085689999907 ) ) ;
#2456=CARTESIAN_POINT ( 'NONE',  ( 12.03711594220000158, -93.00000311470000725, 27.59851862110000198 ) ) ;
#2458=VERTEX_POINT ( 'NONE', #11907 ) ;
#2461=CARTESIAN_POINT ( 'NONE',  ( 21.96855572870000017, -93.67384841979999521, 13.21298988309999878 ) ) ;
#2462=CARTESIAN_POINT ( 'NONE',  ( -14.79537251110000007, -100.9197086940000077, 5.022279785309999411 ) ) ;
#2467=CARTESIAN_POINT ( 'NONE',  ( 11.86373224459999776, -101.2530993010000060, -9.493548918760000177 ) ) ;
#2468=CARTESIAN_POINT ( 'NONE',  ( -12.50340864429999854, -94.22763312360000043, -20.80754938939999832 ) ) ;
#2470=CARTESIAN_POINT ( 'NONE',  ( -23.61875799909552143, -94.52293547164087784, -3.856443778712968395 ) ) ;
#2472=LINE ( 'NONE', #18046, #22324 ) ;
#2473=CARTESIAN_POINT ( 'NONE',  ( 14.01198241910000064, -99.55609327400000552, -10.29247172640000052 ) ) ;
#2476=CARTESIAN_POINT ( 'NONE',  ( 0.000000000000000000, -92.50000000000000000, 0.000000000000000000 ) ) ;
#2479=EDGE_LOOP ( 'NONE', ( #4183, #10396, #25072, #3925 ) ) ;
#2480=CARTESIAN_POINT ( 'NONE',  ( -7.333308059120000166, -94.59276479689999917, -22.63874320469999901 ) ) ;
#2483=CARTESIAN_POINT ( 'NONE',  ( -23.92451332507025441, -92.71619979444980686, -18.91739093709076158 ) ) ;
#2488=EDGE_CURVE ( 'NONE', #22088, #22416, #24822, .T. ) ;
#2495=CARTESIAN_POINT ( 'NONE',  ( 17.82341631479999933, -99.75094652120000660, 1.185189151289999909 ) ) ;
#2501=CARTESIAN_POINT ( 'NONE',  ( 7.472221251747646065, -93.86130746277306969, -25.29698305997012042 ) ) ;
#2513=CARTESIAN_POINT ( 'NONE',  ( -17.01429261839999896, -93.08199881499999151, 21.72620143179999985 ) ) ;
#2514=DIRECTION ( 'NONE',  ( 0.000000000000000000, -1.000000000000000000, 0.000000000000000000 ) ) ;
#2515=ORIENTED_EDGE ( 'NONE', *, *, #16076, .T. ) ;
#2516=CARTESIAN_POINT ( 'NONE',  ( -17.64295153049999954, -98.69230457299998704, 8.917116780599998904 ) ) ;
#2517=CARTESIAN_POINT ( 'NONE',  ( -12.65195851542230265, -101.1586404113024429, -9.188934965808664757 ) ) ;
#2518=CARTESIAN_POINT ( 'NONE',  ( 0.6630435622020000030, -100.4071172650000108, -16.77778116909999895 ) ) ;
#2524=CARTESIAN_POINT ( 'NONE',  ( 7.157200201290000230, -99.88067631459999518, 15.79636883619999921 ) ) ;
#2527=CARTESIAN_POINT ( 'NONE',  ( 0.000000000000000000, -90.50000000000000000, 30.50000000000000000 ) ) ;
#2530=CARTESIAN_POINT ( 'NONE',  ( 27.95526608003522639, -92.54383083955177369, 12.19645322206126359 ) ) ;
#2536=CARTESIAN_POINT ( 'NONE',  ( -7.296432207050000507, -100.9364576079999978, 14.18420974400000034 ) ) ;
#2539=CARTESIAN_POINT ( 'NONE',  ( -12.45118061580227042, -101.3846248974119248, -10.37016303958056263 ) ) ;
#2544=LINE ( 'NONE', #9072, #14632 ) ;
#2547=CARTESIAN_POINT ( 'NONE',  ( 0.4820043924829999771, -99.73367660430000115, -17.30272240089999869 ) ) ;
#2550=EDGE_LOOP ( 'NONE', ( #24878, #21852, #15857, #8556 ) ) ;
#2553=CARTESIAN_POINT ( 'NONE',  ( 9.119802927630001221, -98.28914429610000525, 16.69368728350000097 ) ) ;
#2561=EDGE_CURVE ( 'NONE', #27080, #7740, #21105, .T. ) ;
#2563=CARTESIAN_POINT ( 'NONE',  ( 8.069590842209999337, -101.0685850230000113, 13.92289867959999938 ) ) ;
#2568=TOROIDAL_SURFACE ( 'NONE', #7697, 29.91857981989999971, 10.00000000000000000 ) ;
#2576=CARTESIAN_POINT ( 'NONE',  ( -17.54973872020000059, -98.24302442859999474, -7.833773352749999752 ) ) ;
#2578=CARTESIAN_POINT ( 'NONE',  ( -30.44716603537182564, -92.66455718075737025, 1.794472358657231981 ) ) ;
#2579=VERTEX_POINT ( 'NONE', #5776 ) ;
#2586=CARTESIAN_POINT ( 'NONE',  ( -17.80822692750000158, -92.50000000000000000, -18.25149456069999943 ) ) ;
#2589=CARTESIAN_POINT ( 'NONE',  ( -16.62245297557188906, -98.45243480120420543, 8.807067550475276008 ) ) ;
#2593=CARTESIAN_POINT ( 'NONE',  ( -12.96062981900000111, -99.85455315880000171, -11.21122132580000041 ) ) ;
#2596=CARTESIAN_POINT ( 'NONE',  ( -13.32816333360000094, -99.92967571559999840, -11.12411022969999941 ) ) ;
#2597=ORIENTED_EDGE ( 'NONE', *, *, #11344, .T. ) ;
#2601=CARTESIAN_POINT ( 'NONE',  ( -2.247526421790000395, -96.97547177169998633, 20.70814103409999873 ) ) ;
#2602=CARTESIAN_POINT ( 'NONE',  ( 2.602364616200000036, -94.19923974040000303, 25.28353855870000189 ) ) ;
#2604=ORIENTED_EDGE ( 'NONE', *, *, #23443, .T. ) ;
#2605=B_SPLINE_CURVE_WITH_KNOTS ( 'NONE', 5,
 ( #27078, #11756, #12565, #18333, #23660, #13801, #23000, #3703, #7263, #18772, #13952, #27366 ),
 .UNSPECIFIED., .F., .F.,
 ( 6, 3, 3, 6 ),
 ( -25.08217527079999698, -18.82032368495484675, -10.56887946708883064, -7.186327137116709451 ),
 .UNSPECIFIED. ) ;
#2607=CARTESIAN_POINT ( 'NONE',  ( 21.40421767500000172, -94.24983954939999364, 13.68415878530000107 ) ) ;
#2610=FACE_OUTER_BOUND ( 'NONE', #14099, .T. ) ;
#2614=CARTESIAN_POINT ( 'NONE',  ( -14.04594405749999986, -93.61368346409999219, -21.04238476760000154 ) ) ;
#2616=VERTEX_POINT ( 'NONE', #25611 ) ;
#2619=B_SPLINE_CURVE_WITH_KNOTS ( 'NONE', 3,
 ( #5011, #3138, #20907, #18863, #7515, #1111, #5313, #14202, #5453, #27748, #27171, #22955 ),
 .UNSPECIFIED., .F., .F.,
 ( 4, 2, 2, 2, 2, 4 ),
 ( 0.000000000000000000, 0.2500000000000108802, 0.3750000000000217604, 0.4375000000000137113, 0.5000000000000056621, 1.000000000000000000 ),
 .UNSPECIFIED. ) ;
#2620=CARTESIAN_POINT ( 'NONE',  ( 14.05983650520000161, -99.53431386179998697, -10.27466730669999961 ) ) ;
#2628=VERTEX_POINT ( 'NONE', #9998 ) ;
#2633=CARTESIAN_POINT ( 'NONE',  ( 15.71757121830843751, -101.3846248974404460, 3.940829251724543791 ) ) ;
#2637=AXIS2_PLACEMENT_3D ( 'NONE', #379, #9223, #9376 ) ;
#2639=LINE ( 'NONE', #8865, #17284 ) ;
#2640=CARTESIAN_POINT ( 'NONE',  ( 7.077994251930249447, -93.31461711599030195, 27.00880202536949426 ) ) ;
#2644=ORIENTED_EDGE ( 'NONE', *, *, #7665, .T. ) ;
#2646=CARTESIAN_POINT ( 'NONE',  ( 7.181689689069999716, -99.92967571559999840, 15.80535034289999885 ) ) ;
#2649=CARTESIAN_POINT ( 'NONE',  ( 9.156518149657648209, -94.79128788294934793, -23.00520788063733590 ) ) ;
#2650=CARTESIAN_POINT ( 'NONE',  ( -27.33941636499999817, -92.81180222680001179, 1.030446961340000023 ) ) ;
#2651=CARTESIAN_POINT ( 'NONE',  ( -18.83007542230000197, -97.83384886670000924, 6.645594748249999739 ) ) ;
#2653=CARTESIAN_POINT ( 'NONE',  ( 11.61699134809713918, -98.12113811987541112, -16.78456760152103300 ) ) ;
#2656=CARTESIAN_POINT ( 'NONE',  ( 10.26927205930000042, -92.75885938639999040, -25.49696123720000074 ) ) ;
#2659=ORIENTED_EDGE ( 'NONE', *, *, #23375, .T. ) ;
#2660=CARTESIAN_POINT ( 'NONE',  ( 19.57843399940000140, -94.59276292389999696, 13.52682119470000011 ) ) ;
#2662=DIRECTION ( 'NONE',  ( 0.8775825618903722036, 0.000000000000000000, -0.4794255386042041156 ) ) ;
#2670=ORIENTED_EDGE ( 'NONE', *, *, #21882, .F. ) ;
#2672=CARTESIAN_POINT ( 'NONE',  ( 9.385332722619999402, -98.68450614990000247, 16.47661810339999988 ) ) ;
#2673=CARTESIAN_POINT ( 'NONE',  ( 10.23740437490000055, -99.60591711109999835, 14.03865835380000071 ) ) ;
#2674=ORIENTED_EDGE ( 'NONE', *, *, #589, .T. ) ;
#2676=CARTESIAN_POINT ( 'NONE',  ( 20.47205805249999955, -93.24058218799999054, 16.33781131059999936 ) ) ;
#2680=CARTESIAN_POINT ( 'NONE',  ( -12.56720507379640495, -101.6484611540000031, -9.903160520584330939 ) ) ;
#2684=AXIS2_PLACEMENT_3D ( 'NONE', #10869, #18783, #3330 ) ;
#2687=CARTESIAN_POINT ( 'NONE',  ( 7.936175460970000373, -99.23650994359999800, 16.10618517760000046 ) ) ;
#2689=CARTESIAN_POINT ( 'NONE',  ( -7.333307833730000169, -94.59276292389999696, -22.63874420850000035 ) ) ;
#2691=CARTESIAN_POINT ( 'NONE',  ( 11.22133265290000104, -100.9938510739999913, -10.73518741380000030 ) ) ;
#2693=CARTESIAN_POINT ( 'NONE',  ( 15.49409222530310615, -95.04050137967534795, 17.29256239693905073 ) ) ;
#2703=CARTESIAN_POINT ( 'NONE',  ( 7.984254895100000304, -100.9843696920000014, 13.33388511600000115 ) ) ;
#2709=CARTESIAN_POINT ( 'NONE',  ( 25.97241523970000188, -92.68283745200000112, 10.25715990590000004 ) ) ;
#2711=CARTESIAN_POINT ( 'NONE',  ( -13.42523386781685169, -94.35876167532840952, -21.59623076260758978 ) ) ;
#2717=CARTESIAN_POINT ( 'NONE',  ( -20.15180004589999996, -97.32097376039999403, -7.274423422870000877 ) ) ;
#2719=CARTESIAN_POINT ( 'NONE',  ( 8.546518572781618417, -92.66972459458614253, 29.27809851676327924 ) ) ;
#2722=DIRECTION ( 'NONE',  ( -0.3443190008117950063, 0.000000000000000000, 0.9388527177784421474 ) ) ;
#2726=DIRECTION ( 'NONE',  ( -0.3790931394101558771, -0.6121731929912518355, -0.6939253370752848094 ) ) ;
#2728=CARTESIAN_POINT ( 'NONE',  ( -17.53169516290746444, -96.08573336708691670, 13.07164240864208082 ) ) ;
#2729=VERTEX_POINT ( 'NONE', #11123 ) ;
#2733=CARTESIAN_POINT ( 'NONE',  ( 7.794725237649443805, -101.6024172056560815, 14.01240486772618432 ) ) ;
#2734=DIRECTION ( 'NONE',  ( -0.8091158474751273255, 0.000000000000000000, -0.5876491686070921538 ) ) ;
#2736=EDGE_LOOP ( 'NONE', ( #6226, #10424, #9912, #2192, #22297, #13876 ) ) ;
#2737=CARTESIAN_POINT ( 'NONE',  ( 26.96539441263278647, -92.54383083955173106, -14.25194291928822565 ) ) ;
#2738=VERTEX_POINT ( 'NONE', #26174 ) ;
#2741=CARTESIAN_POINT ( 'NONE',  ( -3.966380828739999753, -98.30614355410000371, 19.04978114919999754 ) ) ;
#2742=CARTESIAN_POINT ( 'NONE',  ( 11.26760366760000132, -92.51839641809998227, 27.23952649899999656 ) ) ;
#2752=FACE_OUTER_BOUND ( 'NONE', #15905, .T. ) ;
#2763=DIRECTION ( 'NONE',  ( 0.000000000000000000, -1.000000000000000000, 0.000000000000000000 ) ) ;
#2768=CIRCLE ( 'NONE', #19499, 0.8000000000000003775 ) ;
#2769=CARTESIAN_POINT ( 'NONE',  ( -10.73934281380000044, -93.50968831570000361, -23.38067028629999555 ) ) ;
#2770=CIRCLE ( 'NONE', #24148, 20.64285714289999873 ) ;
#2773=CARTESIAN_POINT ( 'NONE',  ( 15.61948084379431201, -101.6484611539999889, 3.469733395131306963 ) ) ;
#2788=CARTESIAN_POINT ( 'NONE',  ( -6.580578580030000957, -101.1889999979999999, 15.40319725099999992 ) ) ;
#2789=EDGE_CURVE ( 'NONE', #12473, #4490, #11720, .T. ) ;
#2793=AXIS2_PLACEMENT_3D ( 'NONE', #11897, #20807, #28065 ) ;
#2794=CARTESIAN_POINT ( 'NONE',  ( 7.229652833200000295, -101.2530993470000027, 13.36368574970000012 ) ) ;
#2796=CARTESIAN_POINT ( 'NONE',  ( -17.00713571869999896, -99.92967601899998442, 3.484593143450000152 ) ) ;
#2797=DIRECTION ( 'NONE',  ( 0.000000000000000000, 1.000000000000000000, 0.000000000000000000 ) ) ;
#2799=ORIENTED_EDGE ( 'NONE', *, *, #3072, .T. ) ;
#2802=CARTESIAN_POINT ( 'NONE',  ( 0.000000000000000000, -92.50000000000000000, 0.000000000000000000 ) ) ;
#2803=CARTESIAN_POINT ( 'NONE',  ( -13.13823760000467367, -92.72722989462275223, 27.52520356741175789 ) ) ;
#2804=EDGE_LOOP ( 'NONE', ( #1720, #22121, #8458, #4717 ) ) ;
#2809=CARTESIAN_POINT ( 'NONE',  ( -16.89118076489999964, -98.29694271920000403, 8.926253644079999106 ) ) ;
#2819=CARTESIAN_POINT ( 'NONE',  ( 12.43176822059999864, -98.26008456249999767, 14.57113454829999988 ) ) ;
#2820=ORIENTED_EDGE ( 'NONE', *, *, #24466, .T. ) ;
#2824=CARTESIAN_POINT ( 'NONE',  ( -7.443709283000000454, -101.0405520670000072, 14.44167797660000119 ) ) ;
#2825=FACE_OUTER_BOUND ( 'NONE', #9695, .T. ) ;
#2828=AXIS2_PLACEMENT_3D ( 'NONE', #17866, #18455, #403 ) ;
#2829=CARTESIAN_POINT ( 'NONE',  ( 7.500294343269999331, -101.1699703470000031, 13.83260060669999980 ) ) ;
#2834=DIRECTION ( 'NONE',  ( -0.8981584475625418174, 0.000000000000000000, -0.4396719266362647538 ) ) ;
#2838=CARTESIAN_POINT ( 'NONE',  ( 11.43385261259999908, -100.9763228559999959, -10.73324566510000011 ) ) ;
#2840=CARTESIAN_POINT ( 'NONE',  ( 15.77015574596263647, -94.90770262334949336, 17.27435799970811203 ) ) ;
#2844=DIRECTION ( 'NONE',  ( 0.6184463001828854889, 0.000000000000000000, 0.7858270635388554526 ) ) ;
#2852=EDGE_CURVE ( 'NONE', #21621, #5717, #12525, .T. ) ;
#2854=CARTESIAN_POINT ( 'NONE',  ( 23.70295813380000283, -94.59276292389999696, -2.111851990829999970 ) ) ;
#2856=DIRECTION ( 'NONE',  ( 0.000000000000000000, -1.000000000000000000, 0.000000000000000000 ) ) ;
#2859=CARTESIAN_POINT ( 'NONE',  ( 0.4184155361420000552, -92.92146929989999649, -30.38020812550000116 ) ) ;
#2862=CARTESIAN_POINT ( 'NONE',  ( 16.22917866779999940, -99.91102932019998661, 4.812753184709999132 ) ) ;
#2864=DIRECTION ( 'NONE',  ( 1.000000000000000000, 0.000000000000000000, 0.000000000000000000 ) ) ;
#2865=CARTESIAN_POINT ( 'NONE',  ( -17.52282427860000169, -98.26007807950000483, -7.734195792939999592 ) ) ;
#2867=CARTESIAN_POINT ( 'NONE',  ( 8.879714594546598505, -92.75430643264905939, 29.17881595893258506 ) ) ;
#2875=AXIS2_PLACEMENT_3D ( 'NONE', #14983, #8432, #7892 ) ;
#2879=CARTESIAN_POINT ( 'NONE',  ( -15.50938051129999984, -101.3150705480000084, 4.855933523060000034 ) ) ;
#2882=DIRECTION ( 'NONE',  ( 1.000000000000000000, 0.000000000000000000, 0.000000000000000000 ) ) ;
#2884=DIRECTION ( 'NONE',  ( 0.000000000000000000, 1.000000000000000000, 0.000000000000000000 ) ) ;
#2885=CARTESIAN_POINT ( 'NONE',  ( 15.89267423569999949, -101.2490009469999990, 2.460413036130000286 ) ) ;
#2891=CARTESIAN_POINT ( 'NONE',  ( -2.620111886150000124, -97.23151481229999149, 21.21167663179999963 ) ) ;
#2894=CARTESIAN_POINT ( 'NONE',  ( 5.617108918220000469, -93.05272100550000403, 26.49227707150000199 ) ) ;
#2897=EDGE_LOOP ( 'NONE', ( #1127, #12201, #26392, #17100 ) ) ;
#2900=ORIENTED_EDGE ( 'NONE', *, *, #1713, .F. ) ;
#2904=CARTESIAN_POINT ( 'NONE',  ( -8.907626117019999512, -96.37889029669999275, -20.95313078519999905 ) ) ;
#2906=LINE ( 'NONE', #12193, #6854 ) ;
#2909=CARTESIAN_POINT ( 'NONE',  ( -16.13888085079999613, -100.3684813130000038, 2.534467327679999826 ) ) ;
#2912=ADVANCED_FACE ( 'NONE', ( #5337 ), #22924, .F. ) ;
#2914=DIRECTION ( 'NONE',  ( 1.000000000000000000, 0.000000000000000000, 0.000000000000000000 ) ) ;
#2917=ORIENTED_EDGE ( 'NONE', *, *, #11507, .T. ) ;
#2921=CARTESIAN_POINT ( 'NONE',  ( 16.58398298995137665, -100.1994045927079924, 4.339543189922326683 ) ) ;
#2922=CARTESIAN_POINT ( 'NONE',  ( 19.72731200591455192, -94.57749869813547150, 14.01461210758740705 ) ) ;
#2923=VERTEX_POINT ( 'NONE', #22975 ) ;
#2931=ORIENTED_EDGE ( 'NONE', *, *, #6076, .F. ) ;
#2938=CIRCLE ( 'NONE', #21524, 0.4999999999999995559 ) ;
#2939=CARTESIAN_POINT ( 'NONE',  ( 14.62247892739999955, -92.50000000000000000, 26.76626813769999913 ) ) ;
#2952=CARTESIAN_POINT ( 'NONE',  ( -14.42556421679999978, -101.1889999979999999, -2.978755036369999942 ) ) ;
#2953=CARTESIAN_POINT ( 'NONE',  ( -12.61948338259999858, -101.5369810359999860, -9.836088610590000059 ) ) ;
#2955=VERTEX_POINT ( 'NONE', #9102 ) ;
#2956=EDGE_CURVE ( 'NONE', #4122, #24455, #3876, .T. ) ;
#2957=CARTESIAN_POINT ( 'NONE',  ( -16.12708711420000185, -99.55613392470000633, 6.748578067059999519 ) ) ;
#2959=CARTESIAN_POINT ( 'NONE',  ( 0.4290680484630000069, -99.83167681540000160, -17.32407653439999962 ) ) ;
#2962=CARTESIAN_POINT ( 'NONE',  ( 23.53302756460000111, -92.50000000000000000, -18.47479450719999861 ) ) ;
#2966=B_SPLINE_CURVE_WITH_KNOTS ( 'NONE', 3,
 ( #8331, #12416, #28446, #17524, #6153, #28589, #5872, #14888, #21331, #8481, #1389, #12984, #21894, #21471, #21748, #10231, #16962, #15023, #10788, #26412, #6442, #19146, #28033, #8073, #14752, #17382, #3698, #17234, #1799, #1525 ),
 .UNSPECIFIED., .F., .F.,
 ( 4, 1, 1, 1, 1, 2, 2, 1, 1, 1, 1, 2, 2, 2, 1, 1, 1, 1, 2, 2, 4 ),
 ( 0.000000000000000000, 0.1249999999999382994, 0.1874999999999068523, 0.2187499999998906153, 0.2343749999998821498, 0.2421874999998781253, 0.2499999999998741007, 0.3749999999998134825, 0.4374999999997830069, 0.4687499999997698508, 0.4843749999997616351, 0.4921874999997594147, 0.4999999999997573052, 0.6249999999997394307, 0.6874999999997285505, 0.7187499999997207789, 0.7343749999997143396, 0.7421874999997097877, 0.7460937499997096767, 0.7499999999997094546, 1.000000000000000000 ),
 .UNSPECIFIED. ) ;
#2969=EDGE_LOOP ( 'NONE', ( #4500, #10238 ) ) ;
#2972=CARTESIAN_POINT ( 'NONE',  ( 14.99988783689999927, -97.32097506000000919, 15.29756773239999923 ) ) ;
#2976=DIRECTION ( 'NONE',  ( 0.000000000000000000, 1.000000000000000000, 0.000000000000000000 ) ) ;
#2977=CARTESIAN_POINT ( 'NONE',  ( -8.226221597980000411, -100.1275643909999928, 14.47297520289999895 ) ) ;
#2979=CARTESIAN_POINT ( 'NONE',  ( -10.36222220525591631, -93.92272615323433627, -23.21778344804266325 ) ) ;
#2981=AXIS2_PLACEMENT_3D ( 'NONE', #18313, #6951, #26770 ) ;
#2982=CARTESIAN_POINT ( 'NONE',  ( 7.593106369170000036, -101.5369811139999996, 14.08349511319999969 ) ) ;
#2989=CARTESIAN_POINT ( 'NONE',  ( 11.85750691279999991, -101.2995922080000071, -10.62593904340000073 ) ) ;
#2991=CARTESIAN_POINT ( 'NONE',  ( 12.71397128391526721, -96.41053128091054703, 17.27455293077128573 ) ) ;
#3003=CARTESIAN_POINT ( 'NONE',  ( 6.553154880760000189, -101.1030539030000028, 13.97735961090000067 ) ) ;
#3004=CARTESIAN_POINT ( 'NONE',  ( -13.46646228700000059, -111.0000000000000000, -9.098096927170001180 ) ) ;
#3011=CYLINDRICAL_SURFACE ( 'NONE', #16532, 5.000000000000000000 ) ;
#3013=CARTESIAN_POINT ( 'NONE',  ( 0.000000000000000000, -101.2530993010000060, 0.000000000000000000 ) ) ;
#3018=DIRECTION ( 'NONE',  ( 0.000000000000000000, 1.000000000000000000, 0.000000000000000000 ) ) ;
#3021=CARTESIAN_POINT ( 'NONE',  ( -30.44841632907958129, -92.65976904079269616, 1.773215843239575928 ) ) ;
#3023=CARTESIAN_POINT ( 'NONE',  ( 0.1128683156097121110, -101.5740747342138803, -16.05694931027083783 ) ) ;
#3024=B_SPLINE_CURVE_WITH_KNOTS ( 'NONE', 3,
 ( #8503, #17110, #14905, #4285, #12719, #22205, #26298, #2250, #13007, #28609, #11093, #8353, #13157, #79, #25998, #23814, #21631, #1681, #10521, #17254, #23959, #11853, #6772, #22652, #2840, #27022, #9524, #4720, #7354, #2693, #672, #26874, #11699, #17836, #15633, #24687, #16217, #25131, #5164, #8930, #24976, #26734, #5007, #22953, #11550, #14045, #11256, #20305, #24531, #13897, #13601, #2991, #18278, #18126, #7207, #4570, #233, #2553 ),
 .UNSPECIFIED., .F., .F.,
 ( 4, 2, 1, 1, 2, 2, 2, 1, 1, 2, 2, 1, 1, 2, 2, 1, 1, 1, 1, 1, 2, 2, 2, 2, 1, 1, 1, 2, 2, 2, 2, 1, 1, 1, 1, 2, 2, 4 ),
 ( 0.000000000000000000, 0.007812500000005218048, 0.01171875000000782707, 0.01367187500000852096, 0.01464843750001047946, 0.01562500000001243797, 0.02343750000001134856, 0.02734375000001080386, 0.02929687500001182041, 0.03027343750001156020, 0.03125000000001129652, 0.04687500000001742356, 0.05468750000002103873, 0.05859375000002389755, 0.06250000000002675637, 0.09375000000004667100, 0.1093750000000555112, 0.1171875000000596329, 0.1210937500000619227, 0.1230468750000631023, 0.1240234375000626582, 0.1250000000000622002, 0.1875000000001452727, 0.2187500000001867950, 0.2343750000002075562, 0.2421875000002177147, 0.2460937500002227940, 0.2480468750002245704, 0.2500000000002263190, 0.3750000000002354783, 0.4375000000002389200, 0.4687500000002393086, 0.4843750000002381428, 0.4921875000002358669, 0.4960937500002358669, 0.4980468750002362555, 0.5000000000002366995, 1.000000000000000000 ),
 .UNSPECIFIED. ) ;
#3026=CARTESIAN_POINT ( 'NONE',  ( -12.83089869019999973, -99.70407914540000149, -11.44895565849999919 ) ) ;
#3029=CARTESIAN_POINT ( 'NONE',  ( 23.70206688740000089, -94.36515553530000489, -7.408338407089999578 ) ) ;
#3032=CARTESIAN_POINT ( 'NONE',  ( 13.94245834920000071, -96.73974214399999028, -16.03213923699999910 ) ) ;
#3039=CARTESIAN_POINT ( 'NONE',  ( 15.77847589470000145, -100.9405348700000076, 2.296806114620000283 ) ) ;
#3040=ORIENTED_EDGE ( 'NONE', *, *, #9105, .T. ) ;
#3042=AXIS2_PLACEMENT_3D ( 'NONE', #9106, #15957, #402 ) ;
#3047=CARTESIAN_POINT ( 'NONE',  ( 1.312670351570000005, -94.71480777040000021, 24.32357384970000069 ) ) ;
#3050=CARTESIAN_POINT ( 'NONE',  ( -28.44467018057688534, -93.18010901174839944, 2.040524032743244565 ) ) ;
#3052=CARTESIAN_POINT ( 'NONE',  ( -1.869165715791609950, -94.36683344921111427, 24.51523021183322726 ) ) ;
#3062=DIRECTION ( 'NONE',  ( 1.000000000000000000, 0.000000000000000000, 0.000000000000000000 ) ) ;
#3064=CARTESIAN_POINT ( 'NONE',  ( -15.23833467649999918, -101.0223712829999982, 2.799529863349999648 ) ) ;
#3070=CARTESIAN_POINT ( 'NONE',  ( -7.921025165613940544, -100.1994045928917956, 15.20254870833589145 ) ) ;
#3072=EDGE_CURVE ( 'NONE', #15581, #4465, #5696, .T. ) ;
#3077=CARTESIAN_POINT ( 'NONE',  ( 15.76345192703606024, -101.3038909014199760, 4.015656894647334774 ) ) ;
#3082=CARTESIAN_POINT ( 'NONE',  ( -29.76178938840000043, -91.50000000000000000, 6.669774538800000485 ) ) ;
#3089=CARTESIAN_POINT ( 'NONE',  ( -5.487411647150000071, -100.8733988930000010, 14.73625039430000072 ) ) ;
#3097=CARTESIAN_POINT ( 'NONE',  ( 0.000000000000000000, -92.50000000000000000, 29.91857981989999971 ) ) ;
#3099=CARTESIAN_POINT ( 'NONE',  ( 18.39061537769999788, -98.53908914310000000, 3.638009050179999981 ) ) ;
#3100=CARTESIAN_POINT ( 'NONE',  ( -20.48363899790000175, -93.24064650399999721, 16.32317473610000036 ) ) ;
#3101=DIRECTION ( 'NONE',  ( -0.9999381462442837876, 0.000000000000000000, 0.01112221585590941926 ) ) ;
#3102=EDGE_LOOP ( 'NONE', ( #16143, #17346, #14193, #8940 ) ) ;
#3107=EDGE_LOOP ( 'NONE', ( #19832, #5934, #15126, #22723, #28574 ) ) ;
#3108=CARTESIAN_POINT ( 'NONE',  ( -17.84952382330000020, -94.52419442680000827, 16.07137070119999933 ) ) ;
#3117=EDGE_CURVE ( 'NONE', #22747, #17308, #17717, .T. ) ;
#3123=CARTESIAN_POINT ( 'NONE',  ( -17.07013490150000123, -92.69457892460000892, -23.53491425640000045 ) ) ;
#3125=ADVANCED_FACE ( 'NONE', ( #2273 ), #11745, .F. ) ;
#3126=CARTESIAN_POINT ( 'NONE',  ( 7.584268293420000084, -101.6484612600000048, 14.08825297070000104 ) ) ;
#3128=CARTESIAN_POINT ( 'NONE',  ( 0.000000000000000000, -102.5000000000000000, 0.000000000000000000 ) ) ;
#3129=B_SPLINE_CURVE_WITH_KNOTS ( 'NONE', 5,
 ( #7096, #3026, #995, #9838, #16404, #27494, #9691, #11880, #22678, #27050, #4898, #7383 ),
 .UNSPECIFIED., .F., .F.,
 ( 6, 3, 3, 6 ),
 ( 0.000000000000000000, 0.4964111757615384257, 0.7833083924331027958, 1.000000000000000000 ),
 .UNSPECIFIED. ) ;
#3130=DIRECTION ( 'NONE',  ( -0.000000000000000000, 1.000000000000000000, 0.000000000000000000 ) ) ;
#3131=CARTESIAN_POINT ( 'NONE',  ( 11.52544325100000044, -97.14975610999999844, -17.91795520970000055 ) ) ;
#3132=VERTEX_POINT ( 'NONE', #17279 ) ;
#3134=CARTESIAN_POINT ( 'NONE',  ( 11.48112218699999865, -101.1411470150000014, -10.24881966589999926 ) ) ;
#3136=CARTESIAN_POINT ( 'NONE',  ( -17.71736434265992699, -92.62800705135339285, 24.82640349161211901 ) ) ;
#3138=CARTESIAN_POINT ( 'NONE',  ( 12.01314480165432563, -101.6484611540000031, -10.56820974955409298 ) ) ;
#3142=CARTESIAN_POINT ( 'NONE',  ( 6.902456655579999989, -101.3852859389999992, 14.42727485510000029 ) ) ;
#3144=CARTESIAN_POINT ( 'NONE',  ( -11.20160157070000118, -94.96737615119999987, -21.25938373800000036 ) ) ;
#3147=B_SPLINE_CURVE_WITH_KNOTS ( 'NONE', 5,
 ( #240, #6919, #6627, #9085, #15785, #4726 ),
 .UNSPECIFIED., .F., .F.,
 ( 6, 6 ),
 ( 0.000000000000000000, 1.000000000000000000 ),
 .UNSPECIFIED. ) ;
#3149=ADVANCED_FACE ( 'NONE', ( #8660 ), #2132, .T. ) ;
#3157=ADVANCED_FACE ( 'NONE', ( #19601 ), #17289, .F. ) ;
#3160=EDGE_CURVE ( 'NONE', #22409, #927, #19190, .T. ) ;
#3162=CARTESIAN_POINT ( 'NONE',  ( 0.5651181260435291787, -100.9609609850402308, -16.52593752888986245 ) ) ;
#3163=CYLINDRICAL_SURFACE ( 'NONE', #19103, 5.000000000000001776 ) ;
#3167=CARTESIAN_POINT ( 'NONE',  ( 23.92053897610000135, -93.00000000000000000, -18.92241567810000191 ) ) ;
#3172=FILL_AREA_STYLE ('',( #1003 ) ) ;
#3176=EDGE_LOOP ( 'NONE', ( #12884, #5708, #1307, #23802 ) ) ;
#3178=CARTESIAN_POINT ( 'NONE',  ( -2.575778565979999879, -97.41042627209999694, 21.30187829299999791 ) ) ;
#3179=CARTESIAN_POINT ( 'NONE',  ( 2.583222064299999676, -94.01600108440000270, 25.18845981800000189 ) ) ;
#3183=LINE ( 'NONE', #14103, #27526 ) ;
#3184=DIRECTION ( 'NONE',  ( 0.000000000000000000, 1.000000000000000000, 0.000000000000000000 ) ) ;
#3190=CIRCLE ( 'NONE', #12020, 16.00000000000000000 ) ;
#3191=CARTESIAN_POINT ( 'NONE',  ( 26.73327916010000038, -93.00000450890000536, -12.41348522350000039 ) ) ;
#3196=LINE ( 'NONE', #16441, #12518 ) ;
#3197=CARTESIAN_POINT ( 'NONE',  ( -15.84587239670000258, -101.4177331369999990, 3.264600553649999792 ) ) ;
#3200=VECTOR ( 'NONE', #1123, 1000.000000000000000 ) ;
#3203=CARTESIAN_POINT ( 'NONE',  ( -7.919901001398579332, -100.1517898586247952, 15.24641937776444323 ) ) ;
#3208=CARTESIAN_POINT ( 'NONE',  ( 16.76861568428709504, -99.99762666420065216, 4.276776115527929356 ) ) ;
#3211=AXIS2_PLACEMENT_3D ( 'NONE', #20237, #24170, #6838 ) ;
#3212=EDGE_CURVE ( 'NONE', #28629, #16297, #6669, .T. ) ;
#3217=CARTESIAN_POINT ( 'NONE',  ( -6.665307709260000379, -93.00000000000000000, -13.13558364449999871 ) ) ;
#3221=CARTESIAN_POINT ( 'NONE',  ( -5.452248121450000262, -100.9938510739999913, 14.54082342019999885 ) ) ;
#3223=EDGE_CURVE ( 'NONE', #4878, #139, #17155, .T. ) ;
#3226=EDGE_CURVE ( 'NONE', #16528, #18883, #11881, .T. ) ;
#3234=TOROIDAL_SURFACE ( 'NONE', #7434, 18.14285714289999873, 0.5000000000000000000 ) ;
#3237=CARTESIAN_POINT ( 'NONE',  ( 21.23910705489999984, -96.83679385140000306, 0.8485770364149999301 ) ) ;
#3240=CARTESIAN_POINT ( 'NONE',  ( 29.74110577495378749, -92.77521214521595994, 6.761509561029908078 ) ) ;
#3243=DIRECTION ( 'NONE',  ( 0.4794255386042040601, 0.000000000000000000, 0.8775825618903720926 ) ) ;
#3246=CARTESIAN_POINT ( 'NONE',  ( -8.124727395691921927, -99.57060688036840190, 15.34961553150924374 ) ) ;
#3250=CIRCLE ( 'NONE', #26494, 0.7500000000000006661 ) ;
#3256=DIRECTION ( 'NONE',  ( 1.000000000000000000, 0.000000000000000000, 0.000000000000000000 ) ) ;
#3259=CARTESIAN_POINT ( 'NONE',  ( 7.601090357100000361, -101.6484612010000035, 14.07919707850000002 ) ) ;
#3266=CARTESIAN_POINT ( 'NONE',  ( 7.458107840580000314, -101.1716783650000053, 13.85390195080000098 ) ) ;
#3269=DIRECTION ( 'NONE',  ( -0.000000000000000000, 1.000000000000000000, 0.000000000000000000 ) ) ;
#3270=CARTESIAN_POINT ( 'NONE',  ( 11.00987699500000083, -96.97547176729999308, -17.68222522410000153 ) ) ;
#3273=CARTESIAN_POINT ( 'NONE',  ( 11.95646652419999967, -101.4254868690000109, -10.58588781379999944 ) ) ;
#3281=CARTESIAN_POINT ( 'NONE',  ( -13.55269044519999966, -111.0000000000000000, -9.843123574170000722 ) ) ;
#3282=FACE_OUTER_BOUND ( 'NONE', #8463, .T. ) ;
#3283=EDGE_LOOP ( 'NONE', ( #4893, #18597, #24736, #8867, #10571, #12621 ) ) ;
#3284=CARTESIAN_POINT ( 'NONE',  ( 6.961737886719999935, -101.4121386959999995, 14.38077149549999945 ) ) ;
#3285=CARTESIAN_POINT ( 'NONE',  ( -8.359362780541310656, -94.05619596941960481, -23.03490016510948735 ) ) ;
#3286=CARTESIAN_POINT ( 'NONE',  ( 7.579179873580000226, -101.3235621230000021, 13.98627925510000125 ) ) ;
#3291=TOROIDAL_SURFACE ( 'NONE', #1004, 29.91857981989999971, 10.00000000000000000 ) ;
#3292=LINE ( 'NONE', #837, #26301 ) ;
#3301=CARTESIAN_POINT ( 'NONE',  ( 13.18316069947562141, -92.84927079009474937, 27.50371515764524943 ) ) ;
#3302=CARTESIAN_POINT ( 'NONE',  ( -11.73626289319999927, -94.71481161159999829, -21.34523302109999676 ) ) ;
#3305=CARTESIAN_POINT ( 'NONE',  ( -5.273680924649999824, -107.1975888269999899, -9.653408180790000515 ) ) ;
#3310=ORIENTED_EDGE ( 'NONE', *, *, #22963, .T. ) ;
#3313=PLANE ( 'NONE',  #22299 ) ;
#3319=CARTESIAN_POINT ( 'NONE',  ( -28.34275910430000067, -92.98926436760000058, 1.604598016960000040 ) ) ;
#3322=CARTESIAN_POINT ( 'NONE',  ( -29.52408826051700075, -93.00000237470420927, 5.228628232560329714 ) ) ;
#3328=AXIS2_PLACEMENT_3D ( 'NONE', #12396, #3130, #14598 ) ;
#3330=DIRECTION ( 'NONE',  ( 0.9601004944592514967, 0.000000000000000000, -0.2796552172570731520 ) ) ;
#3331=VERTEX_POINT ( 'NONE', #25991 ) ;
#3333=CARTESIAN_POINT ( 'NONE',  ( -16.25371433440000146, -100.5776968050000022, 3.032057373910000297 ) ) ;
#3341=EDGE_CURVE ( 'NONE', #7636, #8453, #2770, .T. ) ;
#3349=AXIS2_PLACEMENT_3D ( 'NONE', #18069, #15420, #4956 ) ;
#3350=EDGE_CURVE ( 'NONE', #25460, #7740, #21944, .T. ) ;
#3351=UNCERTAINTY_MEASURE_WITH_UNIT (LENGTH_MEASURE( 1.000000000000000082E-05 ), #10188, 'distance_accuracy_value', 'NONE');
#3352=CARTESIAN_POINT ( 'NONE',  ( 6.688784535489389782, -101.3038909011303161, 14.82808411082569222 ) ) ;
#3354=ORIENTED_EDGE ( 'NONE', *, *, #25773, .F. ) ;
#3358=CARTESIAN_POINT ( 'NONE',  ( -6.181676134210000839, -101.5369810359999860, 14.75803956719999910 ) ) ;
#3361=TOROIDAL_SURFACE ( 'NONE', #8514, 5.500000000000000000, 0.5000000000000000000 ) ;
#3363=PLANE ( 'NONE',  #9255 ) ;
#3370=CARTESIAN_POINT ( 'NONE',  ( 15.74335372269999844, -101.6484611540000031, 2.854262350110000401 ) ) ;
#3371=CARTESIAN_POINT ( 'NONE',  ( -20.56696564920000014, -93.13213601760000415, 16.30486652549999960 ) ) ;
#3373=ORIENTED_EDGE ( 'NONE', *, *, #1537, .T. ) ;
#3375=CARTESIAN_POINT ( 'NONE',  ( 29.72764218755513710, -92.82709422631323548, 6.820359001708948377 ) ) ;
#3378=EDGE_CURVE ( 'NONE', #27814, #4274, #28455, .T. ) ;
#3381=CARTESIAN_POINT ( 'NONE',  ( 21.04158602090314645, -97.05288880075438840, 0.8598937435395828111 ) ) ;
#3385=EDGE_CURVE ( 'NONE', #20072, #23472, #22779, .T. ) ;
#3388=ORIENTED_EDGE ( 'NONE', *, *, #13986, .T. ) ;
#3393=CARTESIAN_POINT ( 'NONE',  ( -13.30460049849999926, -101.3399913430000083, -9.124713982900001241 ) ) ;
#3398=CARTESIAN_POINT ( 'NONE',  ( 7.571226706500000070, -101.3243788949999953, 13.99005347329999793 ) ) ;
#3402=CARTESIAN_POINT ( 'NONE',  ( 12.01538071500000093, -98.51736893780000059, -15.58690078470000095 ) ) ;
#3407=DIRECTION ( 'NONE',  ( -0.04503285875970657742, 0.000000000000000000, -0.9989855062171465461 ) ) ;
#3408=AXIS2_PLACEMENT_3D ( 'NONE', #216, #512, #6753 ) ;
#3411=CARTESIAN_POINT ( 'NONE',  ( -17.99251962983047548, -92.56492639278971524, 24.62779902097171103 ) ) ;
#3414=EDGE_CURVE ( 'NONE', #19902, #726, #16380, .T. ) ;
#3426=VECTOR ( 'NONE', #24344, 1000.000000000000000 ) ;
#3430=VERTEX_POINT ( 'NONE', #7197 ) ;
#3433=ORIENTED_EDGE ( 'NONE', *, *, #20242, .F. ) ;
#3434=CARTESIAN_POINT ( 'NONE',  ( -30.40640577132692357, -92.81370807101379228, 2.387642233200668151 ) ) ;
#3436=CARTESIAN_POINT ( 'NONE',  ( 0.3872056760440000245, -99.92967571559999840, -17.35614698070000017 ) ) ;
#3439=CARTESIAN_POINT ( 'NONE',  ( 13.68012917844785292, -92.58608763744132375, 27.25993674634458230 ) ) ;
#3450=AXIS2_PLACEMENT_3D ( 'NONE', #3517, #23197, #3243 ) ;
#3452=VECTOR ( 'NONE', #13602, 1000.000000000000000 ) ;
#3456=EDGE_CURVE ( 'NONE', #27709, #2458, #10609, .T. ) ;
#3458=ORIENTED_EDGE ( 'NONE', *, *, #12233, .F. ) ;
#3459=CARTESIAN_POINT ( 'NONE',  ( -27.64435950660053010, -93.39299082529144869, 0.4115795295578285606 ) ) ;
#3465=CARTESIAN_POINT ( 'NONE',  ( 26.45655024610000083, -92.68419354089999729, -7.824660114159999402 ) ) ;
#3469=CARTESIAN_POINT ( 'NONE',  ( -14.91147105619999991, -101.0534797690000062, 4.558379831599999044 ) ) ;
#3470=CARTESIAN_POINT ( 'NONE',  ( -16.52509094760000252, -100.0517779130000093, 2.709010215110000175 ) ) ;
#3475=CIRCLE ( 'NONE', #23926, 0.7500000000000000000 ) ;
#3479=B_SPLINE_CURVE_WITH_KNOTS ( 'NONE', 5,
 ( #15078, #3884, #3746, #23987, #12749, #4021 ),
 .UNSPECIFIED., .F., .F.,
 ( 6, 6 ),
 ( 0.000000000000000000, 1.000000000000000000 ),
 .UNSPECIFIED. ) ;
#3480=EDGE_LOOP ( 'NONE', ( #26192, #10796, #25597, #19751 ) ) ;
#3481=DIRECTION ( 'NONE',  ( 1.000000000000000000, 0.000000000000000000, 0.000000000000000000 ) ) ;
#3484=ORIENTED_EDGE ( 'NONE', *, *, #9550, .T. ) ;
#3485=CIRCLE ( 'NONE', #21167, 30.50000000000000000 ) ;
#3486=AXIS2_PLACEMENT_3D ( 'NONE', #282, #4476, #4624 ) ;
#3488=CARTESIAN_POINT ( 'NONE',  ( 7.181689689069999716, -99.92967571559999840, 15.80535034289999885 ) ) ;
#3495=CARTESIAN_POINT ( 'NONE',  ( 28.15407045200000269, -92.49999926799999628, 8.194203099389998357 ) ) ;
#3496=CARTESIAN_POINT ( 'NONE',  ( -5.935178058420000013, -101.2490009469999990, 14.94671830490000097 ) ) ;
#3500=EDGE_CURVE ( 'NONE', #11909, #7960, #8656, .T. ) ;
#3503=CARTESIAN_POINT ( 'NONE',  ( -13.46646228700000059, -101.3150700380000018, -9.098096927170001180 ) ) ;
#3508=EDGE_CURVE ( 'NONE', #16242, #19815, #14388, .T. ) ;
#3509=CARTESIAN_POINT ( 'NONE',  ( -13.18672279729999985, -99.64579499010000063, -11.23091032149999968 ) ) ;
#3510=CARTESIAN_POINT ( 'NONE',  ( 15.91799941834440268, -101.5019029711150012, 2.484100747937272757 ) ) ;
#3511=CARTESIAN_POINT ( 'NONE',  ( -20.67841902900000051, -93.05545087649998948, 16.29593949070000036 ) ) ;
#3517=CARTESIAN_POINT ( 'NONE',  ( 0.000000000000000000, -108.5000000000000000, 0.000000000000000000 ) ) ;
#3521=CARTESIAN_POINT ( 'NONE',  ( -21.30003612899999865, -111.0000000000000000, -21.83021898440000186 ) ) ;
#3529=ORIENTED_EDGE ( 'NONE', *, *, #6069, .T. ) ;
#3530=CARTESIAN_POINT ( 'NONE',  ( -12.29363612039999865, -101.2530993000000024, -8.928690578759999497 ) ) ;
#3531=EDGE_CURVE ( 'NONE', #20422, #7443, #4179, .T. ) ;
#3533=ORIENTED_EDGE ( 'NONE', *, *, #25266, .T. ) ;
#3534=CARTESIAN_POINT ( 'NONE',  ( -1.228306939259999897, -101.1461863720000025, -16.11255642589999937 ) ) ;
#3535=CARTESIAN_POINT ( 'NONE',  ( 13.01745538959999848, -111.0000000000000000, -10.62006851110000127 ) ) ;
#3537=CARTESIAN_POINT ( 'NONE',  ( 7.202169754829999881, -101.2530994060000040, 13.37848089620000103 ) ) ;
#3540=CARTESIAN_POINT ( 'NONE',  ( 12.85307023921196468, -101.4085864806519481, -9.837083722716631229 ) ) ;
#3542=CARTESIAN_POINT ( 'NONE',  ( 11.15108638419999920, -100.9197081840000010, -10.94438793620000183 ) ) ;
#3543=VERTEX_POINT ( 'NONE', #4520 ) ;
#3545=CARTESIAN_POINT ( 'NONE',  ( 12.04737265750000041, -101.5369810359999860, -10.52904611309999972 ) ) ;
#3547=CARTESIAN_POINT ( 'NONE',  ( -17.98395509190000041, -94.09782194550001577, 17.16060177909999851 ) ) ;
#3548=CARTESIAN_POINT ( 'NONE',  ( -18.59081129359999807, -92.50000000000000000, 24.17915911369999904 ) ) ;
#3550=DIRECTION ( 'NONE',  ( 0.000000000000000000, 1.000000000000000000, 0.000000000000000000 ) ) ;
#3556=CARTESIAN_POINT ( 'NONE',  ( 6.812757346439999750, -99.85455315880000171, 15.72436791289999825 ) ) ;
#3557=CARTESIAN_POINT ( 'NONE',  ( 15.61171978429999996, -101.6311724339999927, 3.565474465639999924 ) ) ;
#3558=CARTESIAN_POINT ( 'NONE',  ( 7.723274522320000557, -101.5232170330000088, 14.02298824230000029 ) ) ;
#3559=CARTESIAN_POINT ( 'NONE',  ( -11.60187077849999859, -94.77767847329999995, -21.32567029700000205 ) ) ;
#3562=CARTESIAN_POINT ( 'NONE',  ( -7.941640844080000150, -99.73367660430000115, 15.38008034509999966 ) ) ;
#3563=CARTESIAN_POINT ( 'NONE',  ( 8.577089147620000631, -94.15497152599999708, -23.87126057090000231 ) ) ;
#3564=EDGE_CURVE ( 'NONE', #5746, #20422, #22628, .T. ) ;
#3565=CARTESIAN_POINT ( 'NONE',  ( 0.000000000000000000, -101.6484611540000031, 0.000000000000000000 ) ) ;
#3568=CARTESIAN_POINT ( 'NONE',  ( -5.487411647150000071, -100.8733988930000010, 14.73625039430000072 ) ) ;
#3569=ORIENTED_EDGE ( 'NONE', *, *, #18939, .F. ) ;
#3571=ORIENTED_EDGE ( 'NONE', *, *, #1592, .T. ) ;
#3573=CARTESIAN_POINT ( 'NONE',  ( 0.1687264450993073983, -101.5409490181601058, -16.08202886997192493 ) ) ;
#3575=CARTESIAN_POINT ( 'NONE',  ( 14.01961443358530701, -92.52249206702738604, 27.08691047983507261 ) ) ;
#3578=DIRECTION ( 'NONE',  ( 0.3799696139668871098, 0.000000000000000000, -0.9249989688977251490 ) ) ;
#3582=EDGE_CURVE ( 'NONE', #2628, #14989, #25053, .T. ) ;
#3584=FACE_OUTER_BOUND ( 'NONE', #21830, .T. ) ;
#3586=CARTESIAN_POINT ( 'NONE',  ( -29.71161915649999941, -93.00000902169999506, 6.352307318500000299 ) ) ;
#3588=EDGE_CURVE ( 'NONE', #17507, #22416, #2451, .T. ) ;
#3599=AXIS2_PLACEMENT_3D ( 'NONE', #17758, #26643, #22423 ) ;
#3602=CARTESIAN_POINT ( 'NONE',  ( -15.55828293370000104, -101.5369810359999860, 3.733608462370000325 ) ) ;
#3607=DIRECTION ( 'NONE',  ( 1.000000000000000000, 0.000000000000000000, 0.000000000000000000 ) ) ;
#3610=CARTESIAN_POINT ( 'NONE',  ( -12.61948338259999858, -111.0000000000000000, -9.836088610590000059 ) ) ;
#3613=ADVANCED_FACE ( 'NONE', ( #14148 ), #3363, .F. ) ;
#3614=DIRECTION ( 'NONE',  ( 0.000000000000000000, 1.000000000000000000, 0.000000000000000000 ) ) ;
#3622=CARTESIAN_POINT ( 'NONE',  ( 6.822492494782297356, -100.4103893717170450, 15.54132353519026566 ) ) ;
#3628=CARTESIAN_POINT ( 'NONE',  ( 27.23434004499999972, -92.57423549739999658, 9.563854126349999873 ) ) ;
#3630=CARTESIAN_POINT ( 'NONE',  ( -5.549654215229999465, -100.9728541479999961, 14.57947289470000030 ) ) ;
#3631=ORIENTED_EDGE ( 'NONE', *, *, #3508, .T. ) ;
#3632=DIRECTION ( 'NONE',  ( 0.000000000000000000, 1.000000000000000000, 0.000000000000000000 ) ) ;
#3633=CARTESIAN_POINT ( 'NONE',  ( -27.21207320324499079, -93.20709273738651746, -3.793618906176141170 ) ) ;
#3636=CARTESIAN_POINT ( 'NONE',  ( 16.77426419571010996, -99.76647888980478740, 4.307225748008878696 ) ) ;
#3639=CARTESIAN_POINT ( 'NONE',  ( -22.27192559399999894, -94.59276292389999696, -8.381615205879999309 ) ) ;
#3640=CARTESIAN_POINT ( 'NONE',  ( 16.75373607410000076, -99.64579499020000242, 4.397195963869999780 ) ) ;
#3641=CARTESIAN_POINT ( 'NONE',  ( -20.16249632440000283, -93.14733754460000625, 18.54048584069999706 ) ) ;
#3642=CARTESIAN_POINT ( 'NONE',  ( 24.33711400909999867, -92.62399497440000573, -16.98201569060000082 ) ) ;
#3647=AXIS2_PLACEMENT_3D ( 'NONE', #16446, #2763, #2914 ) ;
#3649=CARTESIAN_POINT ( 'NONE',  ( 0.000000000000000000, -102.8486084350000027, 0.000000000000000000 ) ) ;
#3661=ORIENTED_EDGE ( 'NONE', *, *, #20576, .F. ) ;
#3662=CARTESIAN_POINT ( 'NONE',  ( -12.97902083080000146, -100.9728541479999961, -8.654750722490000214 ) ) ;
#3663=AXIS2_PLACEMENT_3D ( 'NONE', #7845, #19060, #5654 ) ;
#3664=CARTESIAN_POINT ( 'NONE',  ( -15.07981158940000022, -92.68449574909999455, -23.80217061829999992 ) ) ;
#3665=CARTESIAN_POINT ( 'NONE',  ( -7.959924907470000477, -99.99711545080000974, 15.21642579620000113 ) ) ;
#3667=CARTESIAN_POINT ( 'NONE',  ( -1.561394334049999832, -94.07620464540001137, 24.87225459399999750 ) ) ;
#3671=CARTESIAN_POINT ( 'NONE',  ( 12.96791850173126193, -101.3038909013318118, -9.820641867354686028 ) ) ;
#3672=CARTESIAN_POINT ( 'NONE',  ( -25.57103825560000132, -93.13207089489999646, -5.913928942570000125 ) ) ;
#3674=ORIENTED_EDGE ( 'NONE', *, *, #10874, .T. ) ;
#3682=CARTESIAN_POINT ( 'NONE',  ( -0.1749952543550000184, -101.1716782170000073, -15.73287486140000091 ) ) ;
#3684=DIRECTION ( 'NONE',  ( 0.000000000000000000, 1.000000000000000000, 0.000000000000000000 ) ) ;
#3687=EDGE_LOOP ( 'NONE', ( #16165, #441, #27094, #27383 ) ) ;
#3691=CIRCLE ( 'NONE', #23690, 5.499999999999998224 ) ;
#3692=CARTESIAN_POINT ( 'NONE',  ( 6.678130984960001015, -101.3090757639999993, 14.82851652149999921 ) ) ;
#3693=CARTESIAN_POINT ( 'NONE',  ( -14.75037098800590130, -92.63657771148726283, -24.06201644404302797 ) ) ;
#3695=CARTESIAN_POINT ( 'NONE',  ( -5.344456951210212914, -96.89152197296419899, 20.58333059934093612 ) ) ;
#3698=CARTESIAN_POINT ( 'NONE',  ( 4.391227679578132204, -92.82668962669040980, -30.18223191820092310 ) ) ;
#3701=CARTESIAN_POINT ( 'NONE',  ( 8.738006338790000882, -94.16701134370001114, -22.89272684270000013 ) ) ;
#3703=CARTESIAN_POINT ( 'NONE',  ( -20.48493760250000051, -92.56290624670000966, -20.07155161329999871 ) ) ;
#3704=CARTESIAN_POINT ( 'NONE',  ( 3.778423607708916165, -92.49999918154601630, 28.62985903013981215 ) ) ;
#3712=CARTESIAN_POINT ( 'NONE',  ( -0.8216454186400000692, -101.4254868690000109, -15.94813504319999709 ) ) ;
#3714=CARTESIAN_POINT ( 'NONE',  ( 7.457144889719999448, -111.0000000000000000, 15.05426816870000017 ) ) ;
#3721=LINE ( 'NONE', #19168, #3956 ) ;
#3723=EDGE_CURVE ( 'NONE', #8492, #10101, #21815, .T. ) ;
#3732=CARTESIAN_POINT ( 'NONE',  ( -0.7041684613104601809, -101.1586404113103583, -15.62090672338606190 ) ) ;
#3736=CARTESIAN_POINT ( 'NONE',  ( -19.45768768673364590, -96.57210918401234778, -9.555941133991472825 ) ) ;
#3737=ORIENTED_EDGE ( 'NONE', *, *, #17415, .T. ) ;
#3743=AXIS2_PLACEMENT_3D ( 'NONE', #4029, #6514, #4472 ) ;
#3746=CARTESIAN_POINT ( 'NONE',  ( 11.19714103559999963, -101.2141467319999890, -10.34781371220000068 ) ) ;
#3748=CARTESIAN_POINT ( 'NONE',  ( 19.17604567300720575, -99.07183862241784311, -0.09086224700556182199 ) ) ;
#3749=CARTESIAN_POINT ( 'NONE',  ( -12.56407913139999977, -101.6484611540000031, -9.907171035319999319 ) ) ;
#3761=CARTESIAN_POINT ( 'NONE',  ( 11.70237128448379416, -101.1416252791438950, -10.22752515391487371 ) ) ;
#3771=CARTESIAN_POINT ( 'NONE',  ( -7.593125501599999438, -94.98812477769999418, -22.45811160230000070 ) ) ;
#3774=VERTEX_POINT ( 'NONE', #6419 ) ;
#3778=ORIENTED_EDGE ( 'NONE', *, *, #4617, .F. ) ;
#3779=CARTESIAN_POINT ( 'NONE',  ( -16.86871002079999826, -97.64874574800001028, -10.69232097959999983 ) ) ;
#3780=CARTESIAN_POINT ( 'NONE',  ( 12.72815622549999937, -100.9364576079999978, -9.613728106940000018 ) ) ;
#3781=CARTESIAN_POINT ( 'NONE',  ( -19.16019836899999618, -92.50000000000000000, 22.97842938279999814 ) ) ;
#3782=CARTESIAN_POINT ( 'NONE',  ( 24.67022271940000167, -93.21603264559999502, -11.26210241870000139 ) ) ;
#3784=B_SPLINE_CURVE_WITH_KNOTS ( 'NONE', 5,
 ( #20373, #5784, #21374, #19186, #1433, #7840 ),
 .UNSPECIFIED., .F., .F.,
 ( 6, 6 ),
 ( 0.000000000000000000, 1.000000000000000000 ),
 .UNSPECIFIED. ) ;
#3785=TOROIDAL_SURFACE ( 'NONE', #4728, 21.14285714289999873, 0.5000000000000000000 ) ;
#3789=TOROIDAL_SURFACE ( 'NONE', #27550, 10.00000000000000000, 1.000000000000000000 ) ;
#3795=CARTESIAN_POINT ( 'NONE',  ( 20.78253645173401409, -97.24405583786555951, 1.124206967171268001 ) ) ;
#3800=EDGE_LOOP ( 'NONE', ( #12796, #28418, #1778, #10380 ) ) ;
#3801=DIRECTION ( 'NONE',  ( 0.000000000000000000, -1.000000000000000000, 0.000000000000000000 ) ) ;
#3805=CARTESIAN_POINT ( 'NONE',  ( -12.54665039110000002, -101.1411470150000014, -8.912689559260000394 ) ) ;
#3806=EDGE_CURVE ( 'NONE', #21689, #11679, #7438, .T. ) ;
#3807=CARTESIAN_POINT ( 'NONE',  ( -16.07857726140000310, -92.61154353310000431, -23.75764880570000059 ) ) ;
#3815=CARTESIAN_POINT ( 'NONE',  ( 6.888451955769999913, -99.53431386179998697, 15.99365555089999802 ) ) ;
#3816=ORIENTED_EDGE ( 'NONE', *, *, #2561, .F. ) ;
#3820=DIRECTION ( 'NONE',  ( 0.000000000000000000, 1.000000000000000000, 0.000000000000000000 ) ) ;
#3821=CARTESIAN_POINT ( 'NONE',  ( 25.81289538086879531, -93.01584921695616970, -5.657399889028498663 ) ) ;
#3824=CARTESIAN_POINT ( 'NONE',  ( 0.05326513945900000074, -101.1417990620000040, -15.75792088070000041 ) ) ;
#3826=CARTESIAN_POINT ( 'NONE',  ( 15.07154978059999983, -101.2141467319999890, 2.302521054160000080 ) ) ;
#3830=VERTEX_POINT ( 'NONE', #27420 ) ;
#3831=CARTESIAN_POINT ( 'NONE',  ( 6.101612763509999482, -100.4731125450000064, 15.00927834069999989 ) ) ;
#3832=CARTESIAN_POINT ( 'NONE',  ( 14.89941269380000044, -101.1700440390000040, 3.486984464110000292 ) ) ;
#3833=CARTESIAN_POINT ( 'NONE',  ( -2.903039748510000351, -94.98812477769999418, 23.52859306979999943 ) ) ;
#3838=CARTESIAN_POINT ( 'NONE',  ( 1.951203915629999841, -92.83702889919999279, -29.73265166020000194 ) ) ;
#3839=CARTESIAN_POINT ( 'NONE',  ( 7.025840212360933812, -101.6484611540000174, 14.37514525054935532 ) ) ;
#3840=CARTESIAN_POINT ( 'NONE',  ( -5.969238273050000210, -101.2530993000000024, 13.97222956270000083 ) ) ;
#3842=AXIS2_PLACEMENT_3D ( 'NONE', #10703, #2152, #4030 ) ;
#3843=DIRECTION ( 'NONE',  ( 0.000000000000000000, 1.000000000000000000, 0.000000000000000000 ) ) ;
#3845=CARTESIAN_POINT ( 'NONE',  ( -12.89684236643334536, -100.4010812938312114, -11.04552942129398474 ) ) ;
#3847=EDGE_CURVE ( 'NONE', #21458, #17507, #28791, .T. ) ;
#3851=CARTESIAN_POINT ( 'NONE',  ( -1.062521193220000049, -101.1516803200000112, -15.28978926900000168 ) ) ;
#3852=DIRECTION ( 'NONE',  ( 0.000000000000000000, 1.000000000000000000, 0.000000000000000000 ) ) ;
#3869=CARTESIAN_POINT ( 'NONE',  ( -29.42137572429999892, -92.83702889919999279, 4.713854256609999460 ) ) ;
#3874=ORIENTED_EDGE ( 'NONE', *, *, #25383, .T. ) ;
#3876=B_SPLINE_CURVE_WITH_KNOTS ( 'NONE', 3,
 ( #13923, #22825, #7091, #698, #20328, #11427, #11283, #9551, #24859, #263, #18452, #27336, #7379, #3021, #2578, #11876, #27047, #401, #843, #18598, #9686, #27490, #3434, #28559, #21865, #23113, #4083, #10759, #17352, #8449 ),
 .UNSPECIFIED., .F., .F.,
 ( 4, 1, 1, 1, 1, 2, 2, 1, 1, 1, 1, 2, 2, 2, 1, 1, 1, 1, 2, 2, 4 ),
 ( 0.000000000000000000, 0.1250000000000514866, 0.1875000000000766054, 0.2187500000000884848, 0.2343750000000944245, 0.2421875000000983380, 0.2500000000001022515, 0.3750000000001702527, 0.4375000000002042810, 0.4687500000002198797, 0.4843750000002277067, 0.4921875000002299827, 0.5000000000002322587, 0.6250000000002787770, 0.6875000000003004264, 0.7187500000003108624, 0.7343750000003180789, 0.7421875000003219647, 0.7460937500003220757, 0.7500000000003222977, 1.000000000000000000 ),
 .UNSPECIFIED. ) ;
#3877=ORIENTED_EDGE ( 'NONE', *, *, #7823, .F. ) ;
#3881=ADVANCED_FACE ( 'NONE', ( #28114 ), #6603, .F. ) ;
#3882=CARTESIAN_POINT ( 'NONE',  ( -15.10594828610000029, -101.1292389759999963, 3.502950928120000196 ) ) ;
#3884=CARTESIAN_POINT ( 'NONE',  ( 11.30123137200000016, -101.2530993039999885, -10.15784976960000030 ) ) ;
#3887=CARTESIAN_POINT ( 'NONE',  ( -12.42321381640000055, -101.0405520670000072, -10.47065562140000061 ) ) ;
#3888=CARTESIAN_POINT ( 'NONE',  ( 16.58537890990000108, -94.98812477769999418, 16.93952572510000110 ) ) ;
#3891=CIRCLE ( 'NONE', #17855, 0.4999999999999986677 ) ;
#3897=B_SPLINE_CURVE_WITH_KNOTS ( 'NONE', 5,
 ( #24150, #22407, #8828, #24291, #13498, #11150, #26787, #17745, #26337 ),
 .UNSPECIFIED., .F., .F.,
 ( 6, 3, 6 ),
 ( 0.000000000000000000, 0.5000000000000000000, 1.000000000000000000 ),
 .UNSPECIFIED. ) ;
#3899=CARTESIAN_POINT ( 'NONE',  ( 6.920191221405996629, -100.2392017795743158, 15.64847181329894887 ) ) ;
#3903=ORIENTED_EDGE ( 'NONE', *, *, #8336, .T. ) ;
#3904=CARTESIAN_POINT ( 'NONE',  ( 29.18096563980000013, -92.50000947299999154, 6.925280479609999595 ) ) ;
#3908=CARTESIAN_POINT ( 'NONE',  ( -4.660534226913422451, -96.57210917874438394, -21.17066465899685213 ) ) ;
#3914=CARTESIAN_POINT ( 'NONE',  ( -21.91154649879999994, -92.53610956480000027, -19.81987556260000005 ) ) ;
#3918=CARTESIAN_POINT ( 'NONE',  ( 12.86423915559999998, -101.1412505549999992, -9.792936688159999292 ) ) ;
#3920=CARTESIAN_POINT ( 'NONE',  ( 23.32816514950000197, -93.91547326110000427, -8.285286069360001449 ) ) ;
#3921=VERTEX_POINT ( 'NONE', #14971 ) ;
#3923=CARTESIAN_POINT ( 'NONE',  ( 29.77631732523176566, -92.68577957616035690, 6.604815473007913162 ) ) ;
#3925=ORIENTED_EDGE ( 'NONE', *, *, #17240, .F. ) ;
#3928=CARTESIAN_POINT ( 'NONE',  ( 6.139035473192171466, -92.73901256242973545, 28.87717835461170424 ) ) ;
#3935=ORIENTED_EDGE ( 'NONE', *, *, #1821, .T. ) ;
#3937=VERTEX_POINT ( 'NONE', #17038 ) ;
#3940=EDGE_LOOP ( 'NONE', ( #3816, #24067, #10685, #2239 ) ) ;
#3941=CARTESIAN_POINT ( 'NONE',  ( -13.19565947609999945, -101.4334236450000049, -9.166987053370000638 ) ) ;
#3943=CARTESIAN_POINT ( 'NONE',  ( -14.07810103419999948, -92.69822489080000594, -24.05355070809999773 ) ) ;
#3944=CARTESIAN_POINT ( 'NONE',  ( -7.946020008919999711, -100.0482783049999966, 15.24923535169999944 ) ) ;
#3946=DIRECTION ( 'NONE',  ( 0.000000000000000000, -1.000000000000000000, 0.000000000000000000 ) ) ;
#3949=CARTESIAN_POINT ( 'NONE',  ( 6.114061450890000415, -101.1889999979999999, -13.40104985119999981 ) ) ;
#3951=CARTESIAN_POINT ( 'NONE',  ( 12.62420072685640271, -101.5740747342616856, -9.923100141449944900 ) ) ;
#3954=CARTESIAN_POINT ( 'NONE',  ( 9.015422398089999234, -94.52293512109999085, -22.16844759350000160 ) ) ;
#3956=VECTOR ( 'NONE', #9738, 1000.000000000000000 ) ;
#3957=CARTESIAN_POINT ( 'NONE',  ( -23.77081188420000046, -91.50000000000000000, -19.11016751280000037 ) ) ;
#3958=B_SPLINE_CURVE_WITH_KNOTS ( 'NONE', 3,
 ( #14342, #23378, #23238, #10086, #25563, #21058, #1117, #12285, #11862, #21194, #9671, #9532, #5171, #7929, #14055, #27475, #25709 ),
 .UNSPECIFIED., .F., .F.,
 ( 4, 2, 2, 1, 1, 1, 1, 1, 2, 2, 4 ),
 ( 0.000000000000000000, 0.2500000000000325295, 0.3750000000000475175, 0.4375000000000550116, 0.4687500000000596745, 0.4843750000000613398, 0.4921875000000622280, 0.4960937500000626721, 0.4980468750000630607, 0.5000000000000635048, 1.000000000000000000 ),
 .UNSPECIFIED. ) ;
#3961=CARTESIAN_POINT ( 'NONE',  ( -20.54704754939906763, -92.97190650805515588, 17.33505249212057819 ) ) ;
#3962=ORIENTED_EDGE ( 'NONE', *, *, #6296, .T. ) ;
#3964=B_SPLINE_CURVE_WITH_KNOTS ( 'NONE', 3,
 ( #2672, #15611, #24512, #4548 ),
 .UNSPECIFIED., .F., .F.,
 ( 4, 4 ),
 ( -19.56549066489999689, -15.82800262790000012 ),
 .UNSPECIFIED. ) ;
#3972=CARTESIAN_POINT ( 'NONE',  ( 6.274723105890000596, -100.5027207520000019, 14.99162967899999899 ) ) ;
#3973=CARTESIAN_POINT ( 'NONE',  ( 15.52324312520000049, -101.3138676899999950, 3.505211958319999876 ) ) ;
#3974=CARTESIAN_POINT ( 'NONE',  ( -5.720570170225761863, -97.24405583566215228, 20.01131529210075755 ) ) ;
#3979=ORIENTED_EDGE ( 'NONE', *, *, #14699, .T. ) ;
#3980=CARTESIAN_POINT ( 'NONE',  ( 6.576566045489999901, -93.21603264559999502, -26.30976280700000203 ) ) ;
#3982=CARTESIAN_POINT ( 'NONE',  ( -6.522510977999999682, -101.1411470200000053, 13.93862250449999785 ) ) ;
#3987=CARTESIAN_POINT ( 'NONE',  ( 23.63615965700000032, -94.63960343439998724, -2.179844538739999837 ) ) ;
#3989=CARTESIAN_POINT ( 'NONE',  ( -1.200716280800000035, -101.4309749570000037, -16.11926675319999802 ) ) ;
#3992=CARTESIAN_POINT ( 'NONE',  ( 14.40601943769999949, -92.50000000000000000, 26.88338899689999906 ) ) ;
#3993=CARTESIAN_POINT ( 'NONE',  ( -6.708539788989999586, -101.2358105800000061, 13.65871639999999942 ) ) ;
#3995=CARTESIAN_POINT ( 'NONE',  ( 13.77368720893815635, -100.0863963177836666, -10.35768808805547181 ) ) ;
#3999=DIRECTION ( 'NONE',  ( 0.8172561201429209277, 0.000000000000000000, 0.5762746169049438594 ) ) ;
#4000=ORIENTED_EDGE ( 'NONE', *, *, #16564, .F. ) ;
#4008=CARTESIAN_POINT ( 'NONE',  ( -25.22186920720000103, -94.24983875570001146, -3.042057529720000097 ) ) ;
#4013=CARTESIAN_POINT ( 'NONE',  ( -22.29269500190000386, -94.98812477769999418, -8.065858985560000249 ) ) ;
#4014=CARTESIAN_POINT ( 'NONE',  ( -13.31136841900000078, -101.0685845459999967, -9.042836269629999535 ) ) ;
#4021=CARTESIAN_POINT ( 'NONE',  ( 11.15108825559999950, -100.9197081840000010, -10.94438638200000113 ) ) ;
#4022=B_SPLINE_SURFACE_WITH_KNOTS ( 'NONE', 5, 5, ( 
 ( #6856, #15576, #15421, #8585, #24332, #15718, #2053, #4663, #13388 ),
 ( #22449, #24479, #22292, #2495, #1905, #15267, #11349, #20253, #320 ),
 ( #4372, #22005, #10894, #10747, #19659, #4218, #2341, #13244, #11194 ),
 ( #20106, #4512, #17342, #28549, #8868, #15125, #24034, #17488, #22152 ),
 ( #26372, #6400, #2191, #24187, #13093, #8714, #11031, #6560, #17781 ),
 ( #28681, #17634, #26520, #26669, #6710, #7297, #14139, #909, #9751 ) ),
 .UNSPECIFIED., .F., .F., .F.,
 ( 6, 6 ),
 ( 6, 3, 6 ),
 ( 10.27982891500000129, 28.98450582939999975 ),
 ( 0.000000000000000000, 0.2500000000000000000, 0.5000000000000000000 ),
 .UNSPECIFIED. ) ;
#4025=CARTESIAN_POINT ( 'NONE',  ( -12.44597910190000079, -100.6809449770000100, -10.73533039990000049 ) ) ;
#4027=CARTESIAN_POINT ( 'NONE',  ( -7.129748092820078931, -101.5409490182324532, 14.41619968365793625 ) ) ;
#4029=CARTESIAN_POINT ( 'NONE',  ( 6.623136366559999821, -93.00000000000000000, -29.58057261400000115 ) ) ;
#4030=DIRECTION ( 'NONE',  ( 1.000000000000000000, 0.000000000000000000, 0.000000000000000000 ) ) ;
#4034=CARTESIAN_POINT ( 'NONE',  ( -5.582122996319999864, -100.8816831189999874, 14.77497816989999890 ) ) ;
#4037=VERTEX_POINT ( 'NONE', #21985 ) ;
#4039=CARTESIAN_POINT ( 'NONE',  ( -19.99038385860702505, -95.81012667687654982, 9.711302805237647107 ) ) ;
#4045=CARTESIAN_POINT ( 'NONE',  ( 0.000000000000000000, -102.5000000000000000, 0.000000000000000000 ) ) ;
#4052=CARTESIAN_POINT ( 'NONE',  ( 12.84172902559999940, -100.7776802639999971, -9.219477447620000987 ) ) ;
#4055=AXIS2_PLACEMENT_3D ( 'NONE', #26440, #21921, #26878 ) ;
#4056=CARTESIAN_POINT ( 'NONE',  ( 29.83256477045206623, -92.59735406127096269, 6.345759108124658709 ) ) ;
#4059=DIRECTION ( 'NONE',  ( 1.000000000000000000, 0.000000000000000000, 0.000000000000000000 ) ) ;
#4064=CARTESIAN_POINT ( 'NONE',  ( -0.7914099002037787711, -92.53260370683119618, -30.48976482468907534 ) ) ;
#4068=CARTESIAN_POINT ( 'NONE',  ( -11.29408752129999982, -94.76700071680001258, -21.12307072750000358 ) ) ;
#4074=AXIS2_PLACEMENT_3D ( 'NONE', #17331, #24027, #6251 ) ;
#4078=CARTESIAN_POINT ( 'NONE',  ( -12.81629053550000030, -101.0555477039999914, -8.711806805760000216 ) ) ;
#4082=CARTESIAN_POINT ( 'NONE',  ( 1.741343278310000020, -92.68419354089999729, 27.53437997139999993 ) ) ;
#4083=CARTESIAN_POINT ( 'NONE',  ( -30.40264043347529466, -92.82668962668607548, 2.435048001739037904 ) ) ;
#4092=CARTESIAN_POINT ( 'NONE',  ( 9.370945274540000369, -94.71481430550001335, -22.48432346729999765 ) ) ;
#4096=CARTESIAN_POINT ( 'NONE',  ( -14.80857177290000060, -92.53271748610001168, 24.80080696000000273 ) ) ;
#4097=CARTESIAN_POINT ( 'NONE',  ( -20.54120388167250510, -92.96187023300437602, 17.39114321432820987 ) ) ;
#4101=CARTESIAN_POINT ( 'NONE',  ( 0.5427213986669999768, -100.0482783049999966, -17.18673518379999621 ) ) ;
#4103=CARTESIAN_POINT ( 'NONE',  ( 15.50047883180000063, -101.1716782080000030, 2.701940809000000332 ) ) ;
#4106=VERTEX_POINT ( 'NONE', #11173 ) ;
#4108=CARTESIAN_POINT ( 'NONE',  ( 6.185491179879999635, -101.0875971110000080, 14.11315596670000083 ) ) ;
#4109=CARTESIAN_POINT ( 'NONE',  ( 14.81927149150000034, -101.2530993010000060, 3.356308434120000239 ) ) ;
#4110=CARTESIAN_POINT ( 'NONE',  ( -4.986610887291577754, -96.57210917192522004, 21.09623979869162724 ) ) ;
#4116=CARTESIAN_POINT ( 'NONE',  ( 4.420730772149999765, -92.67327634539999792, -27.51018170170000232 ) ) ;
#4117=CARTESIAN_POINT ( 'NONE',  ( 6.741848109771249931, -101.4304678898295293, 14.69584814897645586 ) ) ;
#4118=DIRECTION ( 'NONE',  ( 1.000000000000000000, 0.000000000000000000, 0.000000000000000000 ) ) ;
#4120=DIRECTION ( 'NONE',  ( 0.4794255386042040601, 0.000000000000000000, 0.8775825618903722036 ) ) ;
#4121=CARTESIAN_POINT ( 'NONE',  ( -13.05879515434285132, -100.1994045928751120, -11.10531386412310262 ) ) ;
#4122=VERTEX_POINT ( 'NONE', #13966 ) ;
#4125=CARTESIAN_POINT ( 'NONE',  ( -0.9221465140669999894, -101.1499348409999897, -15.72402173499999911 ) ) ;
#4132=CARTESIAN_POINT ( 'NONE',  ( -15.39276618189999901, -101.4254873440000040, 4.250919977269999706 ) ) ;
#4133=DIRECTION ( 'NONE',  ( 0.000000000000000000, 1.000000000000000000, 0.000000000000000000 ) ) ;
#4136=AXIS2_PLACEMENT_3D ( 'NONE', #3949, #1503, #6414 ) ;
#4140=CARTESIAN_POINT ( 'NONE',  ( 24.65020093668425005, -93.55106866415557931, -11.39260662483369124 ) ) ;
#4141=CARTESIAN_POINT ( 'NONE',  ( 19.98296175649999995, -94.98812477599999227, 14.17692170039999944 ) ) ;
#4148=CARTESIAN_POINT ( 'NONE',  ( -24.98485751299999791, -93.92589062430000979, -2.982315457539999937 ) ) ;
#4153=EDGE_LOOP ( 'NONE', ( #19680, #18918, #5533, #22054 ) ) ;
#4165=CARTESIAN_POINT ( 'NONE',  ( -13.15133833870000046, -100.9197081840000010, -8.436152112259998503 ) ) ;
#4168=CARTESIAN_POINT ( 'NONE',  ( -12.01303215110000089, -101.1284992150000051, -9.644678736739999536 ) ) ;
#4170=CARTESIAN_POINT ( 'NONE',  ( 25.49913305207284253, -93.00000166546709579, 13.79230533256381186 ) ) ;
#4171=CARTESIAN_POINT ( 'NONE',  ( -7.293834223439488618, -101.4241070620022640, 14.43537265006951742 ) ) ;
#4173=EDGE_CURVE ( 'NONE', #6867, #9479, #13896, .T. ) ;
#4176=CARTESIAN_POINT ( 'NONE',  ( -1.207226396496814180, -101.4218099523420449, -16.12573525851230372 ) ) ;
#4179=B_SPLINE_CURVE_WITH_KNOTS ( 'NONE', 5,
 ( #10758, #4382, #19670, #2063, #28689, #28558 ),
 .UNSPECIFIED., .F., .F.,
 ( 6, 6 ),
 ( 0.000000000000000000, 1.000000000000000000 ),
 .UNSPECIFIED. ) ;
#4183=ORIENTED_EDGE ( 'NONE', *, *, #20242, .T. ) ;
#4184=CARTESIAN_POINT ( 'NONE',  ( -18.95261912118637682, -97.48771974254098893, 6.567162275491772228 ) ) ;
#4186=CARTESIAN_POINT ( 'NONE',  ( 25.89192503760000008, -92.65715432180000732, 10.49931292039999953 ) ) ;
#4188=ORIENTED_EDGE ( 'NONE', *, *, #14258, .T. ) ;
#4191=CARTESIAN_POINT ( 'NONE',  ( -22.87716665625361045, -94.65677004888377155, -7.699218993550634771 ) ) ;
#4195=CARTESIAN_POINT ( 'NONE',  ( -21.87838817989999995, -92.50732182800000203, -19.74814203740000096 ) ) ;
#4200=CARTESIAN_POINT ( 'NONE',  ( 13.83027782289999941, -99.92384627689999377, -9.732040768319999202 ) ) ;
#4202=CARTESIAN_POINT ( 'NONE',  ( -5.405932493604948874, -98.40858131475137327, -19.29511042873029680 ) ) ;
#4207=ORIENTED_EDGE ( 'NONE', *, *, #17771, .T. ) ;
#4210=FACE_OUTER_BOUND ( 'NONE', #24404, .T. ) ;
#4218=CARTESIAN_POINT ( 'NONE',  ( 19.28934113089999869, -98.24904978849998827, -0.4858748118589999443 ) ) ;
#4219=B_SPLINE_CURVE_WITH_KNOTS ( 'NONE', 3,
 ( #26883, #24695, #24983, #4731, #13609, #22517, #1770, #13401, #13107, #6124, #14997, #26095, #19960, #2067, #4232, #10614, #22162, #22019, #8730, #20116, #2202, #6272, #8451, #15278, #19673, #2352, #10905, #24200, #19813, #26529, #19530, #11044, #28692 ),
 .UNSPECIFIED., .F., .F.,
 ( 4, 2, 1, 1, 2, 2, 1, 1, 1, 2, 2, 2, 1, 1, 2, 2, 1, 1, 2, 2, 4 ),
 ( 0.000000000000000000, 0.06249999999994848565, 0.09374999999993488542, 0.1093749999999379940, 0.1171874999999479444, 0.1249999999999578948, 0.1874999999999998335, 0.2187500000000123235, 0.2343750000000191513, 0.2421875000000219269, 0.2500000000000247025, 0.3750000000000558997, 0.4375000000000673905, 0.4687500000000705547, 0.4843750000000699441, 0.5000000000000693889, 0.6250000000000489608, 0.6875000000000387468, 0.7187500000000344169, 0.7500000000000300870, 1.000000000000000000 ),
 .UNSPECIFIED. ) ;
#4225=CARTESIAN_POINT ( 'NONE',  ( -13.10651977150000036, -92.87496808400000248, -23.83817077610000368 ) ) ;
#4228=CARTESIAN_POINT ( 'NONE',  ( -8.882254428079999542, -95.94151723290001144, -20.27227240450000068 ) ) ;
#4230=CARTESIAN_POINT ( 'NONE',  ( 1.631276547419999945, -94.59276292389999696, 23.74086995720000104 ) ) ;
#4231=CARTESIAN_POINT ( 'NONE',  ( -20.27480750739999849, -94.70871900059999859, 12.26045949169999894 ) ) ;
#4232=CARTESIAN_POINT ( 'NONE',  ( -29.70690187338877308, -92.71619979444709259, 6.910137393209939027 ) ) ;
#4234=CARTESIAN_POINT ( 'NONE',  ( 12.00265656396589975, -100.1470170749897619, -13.12398194341028024 ) ) ;
#4237=EDGE_CURVE ( 'NONE', #1488, #1054, #3479, .T. ) ;
#4245=CARTESIAN_POINT ( 'NONE',  ( -18.00579138470000018, -93.94806047000001570, 18.35448323720000019 ) ) ;
#4246=FACE_OUTER_BOUND ( 'NONE', #4153, .T. ) ;
#4247=ORIENTED_EDGE ( 'NONE', *, *, #11163, .T. ) ;
#4250=CARTESIAN_POINT ( 'NONE',  ( 0.7792231278100000269, -100.9137139110000021, -15.61347424839999931 ) ) ;
#4252=CARTESIAN_POINT ( 'NONE',  ( 14.98792925300000078, -101.2530993039999885, 2.502342737139999773 ) ) ;
#4255=ORIENTED_EDGE ( 'NONE', *, *, #4752, .T. ) ;
#4261=CARTESIAN_POINT ( 'NONE',  ( -15.50938051129999984, -111.0000000000000000, 4.855933523060000034 ) ) ;
#4264=CARTESIAN_POINT ( 'NONE',  ( 8.831064156680000110, -94.59276292120000562, -22.09756269280000041 ) ) ;
#4266=LINE ( 'NONE', #10794, #7920 ) ;
#4267=CARTESIAN_POINT ( 'NONE',  ( -6.805335268389999470, -101.3256027139999986, 14.37758720309999916 ) ) ;
#4270=CARTESIAN_POINT ( 'NONE',  ( -13.29096466015767852, -99.96200787834916923, -11.12774058592850679 ) ) ;
#4272=DIRECTION ( 'NONE',  ( 1.000000000000000000, 0.000000000000000000, 0.000000000000000000 ) ) ;
#4274=VERTEX_POINT ( 'NONE', #10696 ) ;
#4276=CARTESIAN_POINT ( 'NONE',  ( -1.125884257989999915, -101.0535396030000044, -15.55188116729999770 ) ) ;
#4279=CARTESIAN_POINT ( 'NONE',  ( -21.30003612899999865, -93.00000000000000000, -21.83021898440000186 ) ) ;
#4281=EDGE_CURVE ( 'NONE', #15723, #7597, #19107, .T. ) ;
#4282=CARTESIAN_POINT ( 'NONE',  ( -14.67001285520000131, -101.1516882750000121, 4.438127419890000702 ) ) ;
#4283=CIRCLE ( 'NONE', #20585, 0.7500000000000006661 ) ;
#4285=CARTESIAN_POINT ( 'NONE',  ( 16.36049596713812093, -94.62565524723831345, 17.22219307773070440 ) ) ;
#4291=CARTESIAN_POINT ( 'NONE',  ( 24.64984454473747277, -93.08996811592339782, -15.39677593028482505 ) ) ;
#4292=CARTESIAN_POINT ( 'NONE',  ( 27.15071147507873306, -93.11247489698153856, 9.921984135710960828 ) ) ;
#4293=VERTEX_POINT ( 'NONE', #1438 ) ;
#4298=EDGE_CURVE ( 'NONE', #19516, #9243, #8290, .T. ) ;
#4300=CARTESIAN_POINT ( 'NONE',  ( -25.76715338260000010, -94.09272382160000348, -2.407609377890000069 ) ) ;
#4304=CARTESIAN_POINT ( 'NONE',  ( 16.25788162539999959, -100.4650220110000021, 4.370703170420000561 ) ) ;
#4305=ORIENTED_EDGE ( 'NONE', *, *, #11011, .F. ) ;
#4307=DIRECTION ( 'NONE',  ( 0.000000000000000000, 1.000000000000000000, 0.000000000000000000 ) ) ;
#4308=ORIENTED_EDGE ( 'NONE', *, *, #11306, .F. ) ;
#4310=ADVANCED_FACE ( 'NONE', ( #20339 ), #16825, .T. ) ;
#4317=EDGE_CURVE ( 'NONE', #4037, #24255, #15946, .T. ) ;
#4319=B_SPLINE_CURVE_WITH_KNOTS ( 'NONE', 3,
 ( #16301, #13975, #3208, #18652, #25358, #25211, #22880, #20837, #18359, #2921, #20538, #16153, #9304, #27393, #27546, #11784, #23165, #895, #7590, #16010, #5093, #610, #13683, #11628, #16455, #11480, #20386, #24915, #5244, #9600, #5388, #6998, #9882, #9453, #15861, #460, #14270, #14128, #18797, #27247, #12069, #13827, #22732, #23026, #3077, #1045, #2633, #20980, #24771, #22590, #4807, #20695, #18207, #755, #27105, #7144, #4946, #2773, #25059 ),
 .UNSPECIFIED., .F., .F.,
 ( 4, 2, 1, 1, 2, 2, 2, 2, 1, 1, 2, 2, 2, 2, 2, 2, 2, 1, 1, 2, 2, 2, 1, 1, 2, 2, 2, 1, 2, 2, 2, 2, 2, 4 ),
 ( 0.000000000000000000, 0.06249999999986541321, 0.09374999999980372645, 0.1093749999997741945, 0.1171874999997657707, 0.1249999999997573330, 0.1874999999997541689, 0.2187499999997595257, 0.2343749999997633837, 0.2421874999997600253, 0.2460937499997583322, 0.2499999999997566391, 0.3124999999997333799, 0.3437499999997205569, 0.3749999999997077338, 0.4374999999996713185, 0.4687499999996531108, 0.4843749999996440070, 0.4921874999996383448, 0.4960937499996446731, 0.4999999999996509459, 0.5624999999997148947, 0.5937499999997458699, 0.6093749999997675193, 0.6171874999997792877, 0.6249999999997910560, 0.6874999999998409050, 0.7187499999998658851, 0.7343749999998772093, 0.7499999999998882005, 0.8124999999999155120, 0.8437499999999296119, 0.8749999999999436007, 1.000000000000000000 ),
 .UNSPECIFIED. ) ;
#4322=CARTESIAN_POINT ( 'NONE',  ( -11.72126804459999860, -100.9137139110000021, -10.34406313869999927 ) ) ;
#4324=CARTESIAN_POINT ( 'NONE',  ( -13.14566783280000095, -99.53431386179998697, -11.42099844400000030 ) ) ;
#4334=EDGE_CURVE ( 'NONE', #19799, #927, #26754, .T. ) ;
#4335=CARTESIAN_POINT ( 'NONE',  ( -5.873421706809999421, -101.3150700380000018, 15.15334630729999965 ) ) ;
#4336=CARTESIAN_POINT ( 'NONE',  ( 12.78426795600000077, -92.51541980399998977, 27.21084123129999810 ) ) ;
#4338=CARTESIAN_POINT ( 'NONE',  ( -19.27031001210522732, -97.04315770582992684, 7.370512498575622296 ) ) ;
#4339=ORIENTED_EDGE ( 'NONE', *, *, #6688, .T. ) ;
#4340=CARTESIAN_POINT ( 'NONE',  ( 21.04495798600000001, -93.87552356599999825, 13.16258487500000030 ) ) ;
#4348=CARTESIAN_POINT ( 'NONE',  ( -20.51010360339999750, -92.96321827540000982, -20.71562969230000206 ) ) ;
#4352=B_SPLINE_CURVE_WITH_KNOTS ( 'NONE', 4,
 ( #8581, #10891, #26514, #11028, #11191 ),
 .UNSPECIFIED., .F., .F.,
 ( 5, 5 ),
 ( 0.000000000000000000, 1.000000000000000000 ),
 .UNSPECIFIED. ) ;
#4353=CARTESIAN_POINT ( 'NONE',  ( 12.08982211680000063, -101.2010924020000004, -9.314613846919998608 ) ) ;
#4355=CARTESIAN_POINT ( 'NONE',  ( -11.69653532996436063, -94.52419745024094766, -20.97822779232529200 ) ) ;
#4356=CIRCLE ( 'NONE', #22042, 1.000000000000000444 ) ;
#4358=CARTESIAN_POINT ( 'NONE',  ( 29.80903961887878850, -92.62938374245408113, 6.455398338214653364 ) ) ;
#4361=DIRECTION ( 'NONE',  ( 0.000000000000000000, 1.000000000000000000, 0.000000000000000000 ) ) ;
#4362=DIRECTION ( 'NONE',  ( 0.000000000000000000, 1.000000000000000000, 0.000000000000000000 ) ) ;
#4363=CARTESIAN_POINT ( 'NONE',  ( -23.99741465927868234, -92.66191076881281674, -18.82493379776595432 ) ) ;
#4365=CARTESIAN_POINT ( 'NONE',  ( -1.177688289451497061, -92.49999999999998579, -30.47756502919148147 ) ) ;
#4366=AXIS2_PLACEMENT_3D ( 'NONE', #13336, #2884, #11441 ) ;
#4368=DIRECTION ( 'NONE',  ( 0.000000000000000000, 1.000000000000000000, 0.000000000000000000 ) ) ;
#4372=CARTESIAN_POINT ( 'NONE',  ( 19.76462585710000042, -98.69238697660000526, -0.3789175872999999695 ) ) ;
#4373=ORIENTED_EDGE ( 'NONE', *, *, #26793, .T. ) ;
#4376=CARTESIAN_POINT ( 'NONE',  ( 14.62247892739999955, -91.50000000000000000, 26.76626813769999913 ) ) ;
#4379=CARTESIAN_POINT ( 'NONE',  ( 16.58537726420000169, -94.98812477769999418, 16.93952758609999876 ) ) ;
#4381=CARTESIAN_POINT ( 'NONE',  ( -8.862540297109999798, -96.28763787000001173, -20.93955327700000169 ) ) ;
#4382=CARTESIAN_POINT ( 'NONE',  ( 7.462391103660000802, -101.2375126459999848, 13.25959037569999843 ) ) ;
#4385=CIRCLE ( 'NONE', #4366, 30.50000000000000000 ) ;
#4389=CARTESIAN_POINT ( 'NONE',  ( 10.13270341610000180, -93.01085527740001169, -25.43967382270000144 ) ) ;
#4390=CARTESIAN_POINT ( 'NONE',  ( 0.000000000000000000, -107.1975888269999899, 0.000000000000000000 ) ) ;
#4392=CARTESIAN_POINT ( 'NONE',  ( 28.66244647610000129, -93.00000000000000000, 10.42660836539999991 ) ) ;
#4396=CARTESIAN_POINT ( 'NONE',  ( -17.76804213369999985, -93.83763213849999829, 19.50200951540000105 ) ) ;
#4401=CARTESIAN_POINT ( 'NONE',  ( 0.6960536556740000158, -100.3517545579999961, -16.73679824259999904 ) ) ;
#4403=CARTESIAN_POINT ( 'NONE',  ( 15.66918838289999982, -101.3256027080000052, 2.740257563980000199 ) ) ;
#4409=CARTESIAN_POINT ( 'NONE',  ( 28.21920633877042661, -92.66972459461230471, 11.57265855722420511 ) ) ;
#4412=CARTESIAN_POINT ( 'NONE',  ( -3.055530930329999784, -94.70873613630000420, 23.49572349450000175 ) ) ;
#4414=CARTESIAN_POINT ( 'NONE',  ( 8.920172905260001173, -94.54719310899999130, -22.12533866800000126 ) ) ;
#4419=CARTESIAN_POINT ( 'NONE',  ( 27.05591625959999647, -101.1889999979999999, 12.64646362319999895 ) ) ;
#4423=CARTESIAN_POINT ( 'NONE',  ( 9.165534020729998232, -98.33329995120000433, 16.60371393490000003 ) ) ;
#4425=CARTESIAN_POINT ( 'NONE',  ( -7.384731337359999870, -94.63960162979999780, -22.55849179059999798 ) ) ;
#4426=CARTESIAN_POINT ( 'NONE',  ( 14.16648691321227815, -92.50630337894781974, 27.01069259898191532 ) ) ;
#4428=CARTESIAN_POINT ( 'NONE',  ( 11.66470437849999975, -101.1042759770000004, -10.63853114260000154 ) ) ;
#4431=CARTESIAN_POINT ( 'NONE',  ( 23.92053897610000135, -93.00000000000000000, -18.92241567810000191 ) ) ;
#4436=CARTESIAN_POINT ( 'NONE',  ( 22.57356305922917628, -93.98969193917014309, 13.12592337714520241 ) ) ;
#4439=B_SPLINE_CURVE_WITH_KNOTS ( 'NONE', 5,
 ( #5037, #5190, #27049, #7095, #15958, #4600 ),
 .UNSPECIFIED., .F., .F.,
 ( 6, 6 ),
 ( 0.000000000000000000, 1.000000000000000000 ),
 .UNSPECIFIED. ) ;
#4440=CARTESIAN_POINT ( 'NONE',  ( 7.750008477179999744, -101.2850603089999879, 13.91843549959999926 ) ) ;
#4449=EDGE_LOOP ( 'NONE', ( #11293, #17968, #10763, #8184, #9815, #6982 ) ) ;
#4450=DIRECTION ( 'NONE',  ( -0.9839596076661280000, 0.000000000000000000, -0.1783913968820232399 ) ) ;
#4453=ORIENTED_EDGE ( 'NONE', *, *, #6926, .T. ) ;
#4460=CARTESIAN_POINT ( 'NONE',  ( 24.46247886789999981, -92.83702889919999279, -17.01249244230000102 ) ) ;
#4463=CARTESIAN_POINT ( 'NONE',  ( 14.07913102130000027, -97.93128678259999731, -14.20797793960000099 ) ) ;
#4465=VERTEX_POINT ( 'NONE', #12629 ) ;
#4466=DIRECTION ( 'NONE',  ( 1.000000000000000000, 0.000000000000000000, 0.000000000000000000 ) ) ;
#4468=CARTESIAN_POINT ( 'NONE',  ( -13.20967871329999888, -99.69348480060000384, -11.20452871620000046 ) ) ;
#4472=DIRECTION ( 'NONE',  ( 0.6285074900730011072, 0.000000000000000000, -0.7778035323409996371 ) ) ;
#4474=EDGE_CURVE ( 'NONE', #2458, #7636, #23656, .T. ) ;
#4476=DIRECTION ( 'NONE',  ( 1.555923129751019993E-15, 1.000000000000000000, 1.096297985141100053E-15 ) ) ;
#4477=CARTESIAN_POINT ( 'NONE',  ( -5.750263158049999213, -100.9405345029999950, 14.87178882549999948 ) ) ;
#4479=CARTESIAN_POINT ( 'NONE',  ( -19.68295015794943126, -96.39141346198870508, 8.586065742081073537 ) ) ;
#4482=CARTESIAN_POINT ( 'NONE',  ( 21.21659859809999915, -93.92589142420000314, 13.52749749360000031 ) ) ;
#4485=CARTESIAN_POINT ( 'NONE',  ( 16.46460381570141962, -94.70873790529931568, 17.03825317169986064 ) ) ;
#4489=CARTESIAN_POINT ( 'NONE',  ( -6.665307709260000379, -92.50000000000000000, -13.13558364449999871 ) ) ;
#4490=VERTEX_POINT ( 'NONE', #23076 ) ;
#4491=CARTESIAN_POINT ( 'NONE',  ( -5.909020910341554078, -101.4218099524584602, 15.05258134268767378 ) ) ;
#4496=CARTESIAN_POINT ( 'NONE',  ( -1.977702949901789520, -100.7438493865795692, -16.89156302428552436 ) ) ;
#4500=ORIENTED_EDGE ( 'NONE', *, *, #16529, .T. ) ;
#4502=FACE_OUTER_BOUND ( 'NONE', #22257, .T. ) ;
#4503=CARTESIAN_POINT ( 'NONE',  ( -24.05612431029909715, -92.62938374242331463, -18.74977050185806604 ) ) ;
#4510=ORIENTED_EDGE ( 'NONE', *, *, #28496, .F. ) ;
#4512=CARTESIAN_POINT ( 'NONE',  ( 21.31239851289999976, -97.32097375579999721, -2.189509325750000013 ) ) ;
#4517=CARTESIAN_POINT ( 'NONE',  ( 13.46942446439999941, -96.16288795909999010, 17.21854863529999946 ) ) ;
#4518=CARTESIAN_POINT ( 'NONE',  ( -5.273680924649999824, -107.5000000000000000, -9.653408180790000515 ) ) ;
#4519=AXIS2_PLACEMENT_3D ( 'NONE', #14714, #10456, #14979 ) ;
#4520=CARTESIAN_POINT ( 'NONE',  ( 1.631276547419999945, -94.59276292389999696, 23.74086995720000104 ) ) ;
#4522=CARTESIAN_POINT ( 'NONE',  ( -18.01262108789999772, -98.65106254609999326, 4.840278925599998949 ) ) ;
#4529=VERTEX_POINT ( 'NONE', #10438 ) ;
#4531=CARTESIAN_POINT ( 'NONE',  ( -13.55845395530000097, -93.00000046469999404, 27.19007896420000137 ) ) ;
#4533=ORIENTED_EDGE ( 'NONE', *, *, #6978, .T. ) ;
#4538=CARTESIAN_POINT ( 'NONE',  ( -12.92437881006504874, -101.4628082233713258, -9.386789896503060504 ) ) ;
#4539=CARTESIAN_POINT ( 'NONE',  ( 0.8834120860809999698, -100.8023006570000035, -15.75170354469999978 ) ) ;
#4540=CARTESIAN_POINT ( 'NONE',  ( 14.28941763439999946, -101.1889999979999999, -3.575252188409999921 ) ) ;
#4542=ADVANCED_FACE ( 'NONE', ( #27447 ), #27598, .T. ) ;
#4547=CARTESIAN_POINT ( 'NONE',  ( 28.07360232333943628, -92.59033770620598602, 11.92235161152704670 ) ) ;
#4548=CARTESIAN_POINT ( 'NONE',  ( 7.181689689069999716, -99.92967571559999840, 15.80535034289999885 ) ) ;
#4549=CARTESIAN_POINT ( 'NONE',  ( 17.23458459540000121, -95.71128709549999769, 14.57456978229999933 ) ) ;
#4560=ORIENTED_EDGE ( 'NONE', *, *, #3456, .F. ) ;
#4564=CARTESIAN_POINT ( 'NONE',  ( -7.550577645110000624, -94.89196973819998959, -22.44319288410000368 ) ) ;
#4565=CARTESIAN_POINT ( 'NONE',  ( -20.38647250310078718, -92.66455718077615700, -22.68571774292804122 ) ) ;
#4568=CARTESIAN_POINT ( 'NONE',  ( 11.83146313070000133, -101.1461874320000049, -11.00634697169999932 ) ) ;
#4570=CARTESIAN_POINT ( 'NONE',  ( 11.46395552116856464, -97.04146848922184176, 17.18158243287650677 ) ) ;
#4571=EDGE_CURVE ( 'NONE', #24255, #9243, #28130, .T. ) ;
#4577=CARTESIAN_POINT ( 'NONE',  ( 9.718892398710000435, -93.00000000000000000, 28.91008700340000104 ) ) ;
#4579=CARTESIAN_POINT ( 'NONE',  ( 28.17677534670164263, -93.02765837720463082, 8.900282725603984701 ) ) ;
#4581=EDGE_CURVE ( 'NONE', #21750, #11312, #6936, .T. ) ;
#4585=CARTESIAN_POINT ( 'NONE',  ( 8.037687215760000115, -101.3302889870000030, 13.99636585439999870 ) ) ;
#4590=CARTESIAN_POINT ( 'NONE',  ( -23.61874792040000060, -94.52293239719999463, -3.856435390649999739 ) ) ;
#4592=CARTESIAN_POINT ( 'NONE',  ( 15.97524996809999998, -100.1512121650000040, 4.654508469899999668 ) ) ;
#4598=CARTESIAN_POINT ( 'NONE',  ( 7.937989663683267416, -92.55017404142785153, 29.44891095136318881 ) ) ;
#4600=CARTESIAN_POINT ( 'NONE',  ( -8.209463884390000743, -99.53431386179998697, 15.35748973489999969 ) ) ;
#4601=AXIS2_PLACEMENT_3D ( 'NONE', #5149, #20750, #4709 ) ;
#4609=CARTESIAN_POINT ( 'NONE',  ( 13.80438629439999865, -99.83167544280000527, -10.46687976449999979 ) ) ;
#4611=DIRECTION ( 'NONE',  ( 0.000000000000000000, 1.000000000000000000, 0.000000000000000000 ) ) ;
#4613=CARTESIAN_POINT ( 'NONE',  ( -12.32361334809999853, -100.1340845430000002, -11.17997075410000107 ) ) ;
#4615=CARTESIAN_POINT ( 'NONE',  ( 14.32275000858649250, -96.09421897364175891, 17.10293378353320648 ) ) ;
#4617=EDGE_CURVE ( 'NONE', #19075, #17884, #19038, .T. ) ;
#4619=CARTESIAN_POINT ( 'NONE',  ( 26.64225616468215563, -92.66972459460608036, -14.84722933505276465 ) ) ;
#4622=CIRCLE ( 'NONE', #25601, 6.000000000000000000 ) ;
#4624=DIRECTION ( 'NONE',  ( 0.1279666792900072403, 8.881784197000502906E-16, -0.9917784676990565318 ) ) ;
#4627=CARTESIAN_POINT ( 'NONE',  ( 12.77963394200000025, -92.50000200689999019, 27.13243699659999919 ) ) ;
#4631=CARTESIAN_POINT ( 'NONE',  ( 26.23214993620000257, -92.98926460689999374, 10.85177180670000041 ) ) ;
#4636=CARTESIAN_POINT ( 'NONE',  ( 11.92432098210000113, -101.1411470200000053, -9.728253486470000766 ) ) ;
#4638=ORIENTED_EDGE ( 'NONE', *, *, #19763, .T. ) ;
#4640=CARTESIAN_POINT ( 'NONE',  ( -6.285925807789999986, -101.6484611540000031, 14.71350185169999847 ) ) ;
#4650=CARTESIAN_POINT ( 'NONE',  ( -7.550578184249999047, -94.89197151660000884, -22.44319203070000057 ) ) ;
#4663=CARTESIAN_POINT ( 'NONE',  ( 15.54119315139999991, -100.8869813350000015, 1.981730678670000190 ) ) ;
#4669=CARTESIAN_POINT ( 'NONE',  ( 5.711762562947686028, -93.38554229049410083, -27.07704979681747659 ) ) ;
#4682=CARTESIAN_POINT ( 'NONE',  ( -17.33149606389999775, -93.33737544240000261, 19.25501164609999805 ) ) ;
#4684=ORIENTED_EDGE ( 'NONE', *, *, #6517, .F. ) ;
#4686=CARTESIAN_POINT ( 'NONE',  ( -14.94261203119999948, -100.8733967390000004, 4.897670397449999768 ) ) ;
#4688=CARTESIAN_POINT ( 'NONE',  ( 0.3417563417390000469, -101.0151300849999814, -15.63443945619999731 ) ) ;
#4690=B_SPLINE_CURVE_WITH_KNOTS ( 'NONE', 3,
 ( #14715, #18059, #17623, #15115, #8576, #26812, #13379, #26961, #6548, #161, #6701, #21993, #17480, #19937, #2483, #26363, #313, #4363, #4503, #9014, #15710, #13528, #22144, #28540, #11340, #20246, #2183, #17920, #15412, #22439, #24620, #1897, #9152 ),
 .UNSPECIFIED., .F., .F.,
 ( 4, 2, 1, 1, 2, 2, 1, 1, 1, 2, 2, 2, 1, 1, 2, 2, 1, 1, 2, 2, 4 ),
 ( 0.000000000000000000, 0.06250000000002969847, 0.09375000000005637157, 0.1093750000000590639, 0.1171875000000546785, 0.1250000000000502931, 0.1875000000001130762, 0.2187500000001388889, 0.2343750000001501854, 0.2421875000001594003, 0.2500000000001686429, 0.3750000000001466050, 0.4375000000001378897, 0.4687500000001335043, 0.4843750000001280087, 0.5000000000001224576, 0.6250000000000865974, 0.6875000000000731637, 0.7187500000000640599, 0.7500000000000549560, 1.000000000000000000 ),
 .UNSPECIFIED. ) ;
#4693=CARTESIAN_POINT ( 'NONE',  ( 7.040046461240000220, -99.69348480060000384, 15.82639634539999918 ) ) ;
#4697=CARTESIAN_POINT ( 'NONE',  ( 13.12517053680000068, -91.50000000000000000, 27.53143473160000099 ) ) ;
#4699=CARTESIAN_POINT ( 'NONE',  ( 12.46091330099999972, -98.29703159100000676, 14.48139617630000053 ) ) ;
#4702=CARTESIAN_POINT ( 'NONE',  ( 26.57391653120000186, -92.50000460620000808, 13.43926559110000163 ) ) ;
#4705=CARTESIAN_POINT ( 'NONE',  ( 10.56566109427459033, -96.61062616328538866, -18.41854727118479218 ) ) ;
#4706=CARTESIAN_POINT ( 'NONE',  ( -6.976086355399999661, -101.3852859389999992, 14.39181666049999997 ) ) ;
#4707=ORIENTED_EDGE ( 'NONE', *, *, #16495, .F. ) ;
#4709=DIRECTION ( 'NONE',  ( 1.000000000000000000, 0.000000000000000000, 0.000000000000000000 ) ) ;
#4713=CARTESIAN_POINT ( 'NONE',  ( 7.501173096960000564, -99.48532946420000656, 15.95771025049999992 ) ) ;
#4717=ORIENTED_EDGE ( 'NONE', *, *, #19026, .F. ) ;
#4718=CARTESIAN_POINT ( 'NONE',  ( 11.43994069400000058, -100.8816835080000089, -10.88980376029999952 ) ) ;
#4720=CARTESIAN_POINT ( 'NONE',  ( 15.52051803399669261, -95.02776861797826768, 17.29095834261395126 ) ) ;
#4721=CIRCLE ( 'NONE', #21026, 18.64285714289999873 ) ;
#4723=B_SPLINE_CURVE_WITH_KNOTS ( 'NONE', 5,
 ( #21148, #1330, #16616, #10174, #5268, #16330 ),
 .UNSPECIFIED., .F., .F.,
 ( 6, 6 ),
 ( 0.000000000000000000, 1.000000000000000000 ),
 .UNSPECIFIED. ) ;
#4726=CARTESIAN_POINT ( 'NONE',  ( 15.50925563669999896, -100.9197081840000010, 1.894558565230000102 ) ) ;
#4727=CARTESIAN_POINT ( 'NONE',  ( 22.18949969423676905, -94.10917102494428832, 13.31178859376489321 ) ) ;
#4728=AXIS2_PLACEMENT_3D ( 'NONE', #27616, #19130, #25418 ) ;
#4729=EDGE_LOOP ( 'NONE', ( #25908, #1629, #10470, #27204 ) ) ;
#4731=CARTESIAN_POINT ( 'NONE',  ( -29.75530570606409597, -92.89593097428694080, 6.698644383117053458 ) ) ;
#4733=CARTESIAN_POINT ( 'NONE',  ( 7.976137737220000190, -101.5137793180000045, 13.98721220989999914 ) ) ;
#4734=ORIENTED_EDGE ( 'NONE', *, *, #27565, .F. ) ;
#4741=EDGE_CURVE ( 'NONE', #17152, #18837, #7869, .T. ) ;
#4743=ORIENTED_EDGE ( 'NONE', *, *, #3582, .T. ) ;
#4747=CARTESIAN_POINT ( 'NONE',  ( -15.35950681959999997, -99.56347590750000620, -8.501124659940000328 ) ) ;
#4748=ORIENTED_EDGE ( 'NONE', *, *, #2168, .F. ) ;
#4752=EDGE_CURVE ( 'NONE', #25977, #9315, #21527, .T. ) ;
#4753=DIRECTION ( 'NONE',  ( -0.3390050494208429743, 0.7071067811866730279, -0.6205445805637129775 ) ) ;
#4761=CARTESIAN_POINT ( 'NONE',  ( -15.64456437664894750, -99.93376895843553598, 6.429786443641783755 ) ) ;
#4762=B_SPLINE_SURFACE_WITH_KNOTS ( 'NONE', 5, 5, ( 
 ( #22586, #9302, #18203, #24911, #22876, #16007 ),
 ( #15707, #9597, #310, #4943, #25056, #13824 ),
 ( #9012, #20243, #2769, #24616, #27390, #20535 ),
 ( #11179, #15858, #13972, #5240, #7436, #606 ),
 ( #16298, #25208, #20094, #9449, #6994, #18356 ),
 ( #158, #4650, #16150, #13526, #22437, #2480 ) ),
 .UNSPECIFIED., .F., .F., .F.,
 ( 6, 6 ),
 ( 6, 6 ),
 ( 14.35373998510000071, 23.44689954260000064 ),
 ( 0.000000000000000000, 0.5000000000000000000 ),
 .UNSPECIFIED. ) ;
#4766=CARTESIAN_POINT ( 'NONE',  ( -13.02860857159999952, -99.94751438429999268, -11.16201040320000004 ) ) ;
#4768=CARTESIAN_POINT ( 'NONE',  ( -13.24425460951195888, -99.76647888979881884, -11.15875677615296091 ) ) ;
#4772=CARTESIAN_POINT ( 'NONE',  ( 26.47131973888236800, -92.75430643216988358, -15.14997898769894036 ) ) ;
#4775=DIRECTION ( 'NONE',  ( 1.000000000000000000, 0.000000000000000000, 0.000000000000000000 ) ) ;
#4776=CARTESIAN_POINT ( 'NONE',  ( -4.062581167790000336, -98.51736893940000073, 19.25659066309999901 ) ) ;
#4777=CARTESIAN_POINT ( 'NONE',  ( 8.007555411949999424, -93.15603699990001019, 27.33235638589999894 ) ) ;
#4782=CARTESIAN_POINT ( 'NONE',  ( 20.62093289109999716, -94.45168212990000711, 13.94874876430000121 ) ) ;
#4789=CARTESIAN_POINT ( 'NONE',  ( 12.19134911989999814, -101.1716782170000073, -9.946103829120000128 ) ) ;
#4791=AXIS2_PLACEMENT_3D ( 'NONE', #7460, #23043, #11943 ) ;
#4792=CARTESIAN_POINT ( 'NONE',  ( -24.07228054242398230, -94.80026864433543210, -4.144187258122226325 ) ) ;
#4793=ORIENTED_EDGE ( 'NONE', *, *, #17906, .T. ) ;
#4795=CARTESIAN_POINT ( 'NONE',  ( 13.80769401629999926, -99.88067631459999518, -10.49277699589999813 ) ) ;
#4798=DIRECTION ( 'NONE',  ( 1.000000000000000000, 0.000000000000000000, 0.000000000000000000 ) ) ;
#4799=FACE_OUTER_BOUND ( 'NONE', #13249, .T. ) ;
#4807=CARTESIAN_POINT ( 'NONE',  ( 15.67135797424042742, -101.4728631013787208, 3.842886462708210438 ) ) ;
#4823=EDGE_LOOP ( 'NONE', ( #12314, #26010, #19397, #24221 ) ) ;
#4824=DIRECTION ( 'NONE',  ( 1.000000000000000000, 0.000000000000000000, 0.000000000000000000 ) ) ;
#4826=AXIS2_PLACEMENT_3D ( 'NONE', #7779, #10073, #23636 ) ;
#4827=CARTESIAN_POINT ( 'NONE',  ( 8.153295725933123350, -94.16483583575367788, -24.44841081015503192 ) ) ;
#4833=CARTESIAN_POINT ( 'NONE',  ( 9.017793344559999369, -92.49999846069999876, -27.43401283590000261 ) ) ;
#4835=CARTESIAN_POINT ( 'NONE',  ( -12.77311630576821244, -92.58347372263071406, 27.69652610236371970 ) ) ;
#4841=CARTESIAN_POINT ( 'NONE',  ( -17.59164495649999793, -96.97509177549999038, 11.15485559729999920 ) ) ;
#4851=ADVANCED_FACE ( 'NONE', ( #12596 ), #5909, .T. ) ;
#4852=DIRECTION ( 'NONE',  ( -0.3928703629870110570, 0.000000000000000000, 0.9195938657290262386 ) ) ;
#4854=CARTESIAN_POINT ( 'NONE',  ( 17.20775814350000132, -95.72998475950001307, 14.36350897220000000 ) ) ;
#4856=AXIS2_PLACEMENT_3D ( 'NONE', #23600, #18827, #21417 ) ;
#4858=CARTESIAN_POINT ( 'NONE',  ( 24.66732901470000172, -92.51556042380001088, 14.76695160569999921 ) ) ;
#4864=CARTESIAN_POINT ( 'NONE',  ( 7.181688671299999882, -99.92967573500000356, 15.80534928199999989 ) ) ;
#4876=CARTESIAN_POINT ( 'NONE',  ( -17.80822692750000158, -111.0000000000000000, -18.25149456069999943 ) ) ;
#4878=VERTEX_POINT ( 'NONE', #9349 ) ;
#4880=AXIS2_PLACEMENT_3D ( 'NONE', #2453, #22404, #4775 ) ;
#4881=CARTESIAN_POINT ( 'NONE',  ( 7.787105047099999844, -101.3792338629999961, 13.97258517809999923 ) ) ;
#4889=CARTESIAN_POINT ( 'NONE',  ( 16.52049151459999976, -99.72202992580000114, 4.688718860289999846 ) ) ;
#4892=CARTESIAN_POINT ( 'NONE',  ( -21.99303270440000446, -95.76596938280000870, -5.803739253210000726 ) ) ;
#4893=ORIENTED_EDGE ( 'NONE', *, *, #20203, .F. ) ;
#4897=AXIS2_PLACEMENT_3D ( 'NONE', #16314, #13989, #9316 ) ;
#4898=CARTESIAN_POINT ( 'NONE',  ( -11.89545460579999947, -101.2530993010000060, -9.453770335970000716 ) ) ;
#4902=CARTESIAN_POINT ( 'NONE',  ( -16.50266362683683141, -98.65920929149453400, 8.461970372646858252 ) ) ;
#4903=EDGE_LOOP ( 'NONE', ( #11305, #7178, #27175, #28486 ) ) ;
#4906=CARTESIAN_POINT ( 'NONE',  ( 7.635702898730000854, -101.6454117330000031, 14.06304778130000166 ) ) ;
#4911=EDGE_CURVE ( 'NONE', #23865, #21973, #28712, .T. ) ;
#4912=CARTESIAN_POINT ( 'NONE',  ( 26.89630156707283959, -92.56492639279250056, -14.38221850968363746 ) ) ;
#4915=EDGE_CURVE ( 'NONE', #8492, #24436, #5537, .T. ) ;
#4916=CIRCLE ( 'NONE', #18889, 30.50000000000000000 ) ;
#4918=DIRECTION ( 'NONE',  ( 0.000000000000000000, -1.000000000000000000, 0.000000000000000000 ) ) ;
#4919=CARTESIAN_POINT ( 'NONE',  ( 7.995248799109998750, -92.98123155529999906, 27.31123713640000261 ) ) ;
#4921=ORIENTED_EDGE ( 'NONE', *, *, #5667, .T. ) ;
#4925=ORIENTED_EDGE ( 'NONE', *, *, #2251, .F. ) ;
#4927=ORIENTED_EDGE ( 'NONE', *, *, #16564, .T. ) ;
#4929=CARTESIAN_POINT ( 'NONE',  ( 12.36959650760000073, -101.3256027139999986, -10.00103415339999913 ) ) ;
#4930=CARTESIAN_POINT ( 'NONE',  ( -14.67423319995313413, -93.10940799664778922, -23.67382460028223434 ) ) ;
#4933=CARTESIAN_POINT ( 'NONE',  ( -17.03413894869999723, -99.61736770250000461, 3.268853260370000235 ) ) ;
#4936=VERTEX_POINT ( 'NONE', #11522 ) ;
#4941=EDGE_LOOP ( 'NONE', ( #5657, #20805, #20571, #19479 ) ) ;
#4942=EDGE_CURVE ( 'NONE', #21621, #22807, #8773, .T. ) ;
#4943=CARTESIAN_POINT ( 'NONE',  ( -11.89700623620000108, -93.14241133300001252, -23.62892427899999959 ) ) ;
#4944=CARTESIAN_POINT ( 'NONE',  ( 23.56050310359999855, -94.79581646409999962, -2.314011072670000058 ) ) ;
#4946=CARTESIAN_POINT ( 'NONE',  ( 15.61464033245285599, -101.6297509123138525, 3.556724360410273178 ) ) ;
#4954=CARTESIAN_POINT ( 'NONE',  ( 11.66718683064264361, -93.00000367782563160, 27.62038300901093280 ) ) ;
#4955=ORIENTED_EDGE ( 'NONE', *, *, #17035, .F. ) ;
#4956=DIRECTION ( 'NONE',  ( 1.000000000000000000, 0.000000000000000000, 0.000000000000000000 ) ) ;
#4958=ORIENTED_EDGE ( 'NONE', *, *, #14386, .T. ) ;
#4959=CARTESIAN_POINT ( 'NONE',  ( 9.279094190537668041, -98.48918237499029260, 16.48187022330440499 ) ) ;
#4963=CARTESIAN_POINT ( 'NONE',  ( -27.33230668875999925, -92.65509297689254709, -4.521833498730020828 ) ) ;
#4964=CARTESIAN_POINT ( 'NONE',  ( -20.20541094980000096, -94.98812148390000232, 12.40015412250000004 ) ) ;
#4965=CARTESIAN_POINT ( 'NONE',  ( -18.84946647679999998, -97.93129755900000077, 6.692285885629999598 ) ) ;
#4966=CARTESIAN_POINT ( 'NONE',  ( -15.50938051129999984, -101.1889999979999999, 4.855933523060000034 ) ) ;
#4969=CARTESIAN_POINT ( 'NONE',  ( 13.12743937220000134, -94.59276479679999738, -19.84843662619999805 ) ) ;
#4973=DIRECTION ( 'NONE',  ( 1.000000000000000000, 0.000000000000000000, 0.000000000000000000 ) ) ;
#4975=DIRECTION ( 'NONE',  ( -0.8775825618903722036, 0.000000000000000000, 0.4794255386042041156 ) ) ;
#4978=CARTESIAN_POINT ( 'NONE',  ( -2.934900197419999746, -94.89197151660000884, 23.49669041109999768 ) ) ;
#4983=ADVANCED_FACE ( 'NONE', ( #6620 ), #6913, .T. ) ;
#4986=DIRECTION ( 'NONE',  ( 0.000000000000000000, -1.000000000000000000, 0.000000000000000000 ) ) ;
#4989=ORIENTED_EDGE ( 'NONE', *, *, #25889, .F. ) ;
#4991=CARTESIAN_POINT ( 'NONE',  ( 16.46460381569999853, -94.70873790529999781, 17.03825317170000275 ) ) ;
#4992=B_SPLINE_SURFACE_WITH_KNOTS ( 'NONE', 5, 5, ( 
 ( #25684, #5709, #3534, #10201, #8176, #14728, #19116, #28006, #10475 ),
 ( #28268, #5845, #12528, #8303, #19252, #17205, #6122, #18340, #26676 ),
 ( #27230, #27373, #8874, #10902, #13104, #19956, #24341, #7415, #6718 ),
 ( #27, #2348, #24197, #17496, #5224, #2198, #8594, #6409, #7268 ),
 ( #2904, #4381, #15429, #19668, #16133, #28688, #11761, #4228, #19810 ),
 ( #11201, #26381, #11041, #25196, #22015, #17788, #6567, #15585, #13957 ) ),
 .UNSPECIFIED., .F., .F., .F.,
 ( 6, 6 ),
 ( 6, 3, 6 ),
 ( 10.27996124010000045, 28.19205293310000116 ),
 ( 0.000000000000000000, 0.2500000000000000000, 0.5000000000000000000 ),
 .UNSPECIFIED. ) ;
#4994=CARTESIAN_POINT ( 'NONE',  ( -6.943253548370000416, -101.2902355740000075, 14.33557670620000124 ) ) ;
#4995=CARTESIAN_POINT ( 'NONE',  ( 6.019085164319999848, -92.50000467790000869, 29.30686339500000059 ) ) ;
#5000=CARTESIAN_POINT ( 'NONE',  ( 8.207855523239999229, -98.78769286879999356, 16.44907893679999944 ) ) ;
#5007=CARTESIAN_POINT ( 'NONE',  ( 14.54939535876293988, -95.49908309382901450, 17.32799205191540892 ) ) ;
#5011=CARTESIAN_POINT ( 'NONE',  ( 12.04737265770000043, -101.6484611540000031, -10.52904611289999970 ) ) ;
#5015=CARTESIAN_POINT ( 'NONE',  ( -15.71875659940000247, -100.6826114469999993, 2.591326689040000186 ) ) ;
#5018=CARTESIAN_POINT ( 'NONE',  ( 6.744238910220000882, -101.2530993010000060, 13.61507422070000040 ) ) ;
#5028=CARTESIAN_POINT ( 'NONE',  ( -14.64295283881845933, -93.98969193940334321, -21.62035027063686599 ) ) ;
#5029=CARTESIAN_POINT ( 'NONE',  ( 16.52775595720000013, -99.70407914540000149, 4.748034318380000229 ) ) ;
#5032=DIRECTION ( 'NONE',  ( 1.000000000000000000, 0.000000000000000000, 0.000000000000000000 ) ) ;
#5034=CARTESIAN_POINT ( 'NONE',  ( 8.538276090549652864, -92.66777315148682703, 29.28050361645156840 ) ) ;
#5037=CARTESIAN_POINT ( 'NONE',  ( -3.215510237749999778, -94.59276292389999696, 23.57860181210000405 ) ) ;
#5049=CARTESIAN_POINT ( 'NONE',  ( -12.57997069900000042, -101.2141467319999890, -8.613800160570001196 ) ) ;
#5051=ORIENTED_EDGE ( 'NONE', *, *, #217, .F. ) ;
#5052=CARTESIAN_POINT ( 'NONE',  ( 27.24068616960000000, -92.50000000000000000, -13.71841889620000110 ) ) ;
#5056=CARTESIAN_POINT ( 'NONE',  ( 1.342713516450000144, -94.57749834670001121, 24.16140173950000047 ) ) ;
#5057=CARTESIAN_POINT ( 'NONE',  ( 4.182785939470000436, -93.31177568259998623, 25.48038252359999944 ) ) ;
#5059=CIRCLE ( 'NONE', #19027, 5.500000000000001776 ) ;
#5060=CARTESIAN_POINT ( 'NONE',  ( -1.527823559601194425, -96.61062616600978004, 21.17880622167292159 ) ) ;
#5065=ORIENTED_EDGE ( 'NONE', *, *, #11624, .T. ) ;
#5076=CARTESIAN_POINT ( 'NONE',  ( 0.3059185938709999553, -93.00000000000000000, 14.72672055670000013 ) ) ;
#5083=FACE_OUTER_BOUND ( 'NONE', #21093, .T. ) ;
#5087=CIRCLE ( 'NONE', #8779, 15.19391340349999986 ) ;
#5093=CARTESIAN_POINT ( 'NONE',  ( 16.34170762565740631, -100.4872618028340838, 4.353002873095284997 ) ) ;
#5095=ORIENTED_EDGE ( 'NONE', *, *, #25673, .T. ) ;
#5097=CYLINDRICAL_SURFACE ( 'NONE', #5662, 18.64285714290000584 ) ;
#5108=CARTESIAN_POINT ( 'NONE',  ( 9.220169834277720966, -98.40144667389034794, 16.53004056780445907 ) ) ;
#5117=CARTESIAN_POINT ( 'NONE',  ( 23.42164048755097383, -94.71481465625956275, -6.692245640674809870 ) ) ;
#5122=EDGE_CURVE ( 'NONE', #27080, #2923, #26013, .T. ) ;
#5129=FACE_OUTER_BOUND ( 'NONE', #22546, .T. ) ;
#5132=CARTESIAN_POINT ( 'NONE',  ( -17.93586394770000325, -95.70815265259999194, 13.56389423130000083 ) ) ;
#5138=B_SPLINE_CURVE_WITH_KNOTS ( 'NONE', 3,
 ( #27641, #7683, #25444, #10806, #6168, #28459, #23667, #17539, #17106, #12848 ),
 .UNSPECIFIED., .F., .F.,
 ( 4, 2, 2, 2, 4 ),
 ( 0.000000000000000000, 0.2500000000000000000, 0.5000000000000000000, 0.7500000000000000000, 1.000000000000000000 ),
 .UNSPECIFIED. ) ;
#5139=ORIENTED_EDGE ( 'NONE', *, *, #13819, .T. ) ;
#5142=CARTESIAN_POINT ( 'NONE',  ( 14.78241224890000183, -96.95622554120001269, 14.77248467170000090 ) ) ;
#5145=CARTESIAN_POINT ( 'NONE',  ( 16.42966481050000027, -94.59276479679999738, 17.21499971510000293 ) ) ;
#5149=CARTESIAN_POINT ( 'NONE',  ( 0.000000000000000000, -111.0000000000000000, 0.000000000000000000 ) ) ;
#5152=CARTESIAN_POINT ( 'NONE',  ( -6.781378104809999030, -101.6484611540000031, 14.49182221120000058 ) ) ;
#5159=CARTESIAN_POINT ( 'NONE',  ( 12.02679296059999814, -98.69238697830000717, -15.68885798269999832 ) ) ;
#5164=CARTESIAN_POINT ( 'NONE',  ( 14.64236194031395044, -95.45364739782090169, 17.32643780036390879 ) ) ;
#5171=CARTESIAN_POINT ( 'NONE',  ( 13.87499543336579144, -97.43022994613481558, -15.19070948534773180 ) ) ;
#5177=FACE_OUTER_BOUND ( 'NONE', #27792, .T. ) ;
#5185=CARTESIAN_POINT ( 'NONE',  ( -17.80939098829999878, -98.43722211970001013, -8.214143917099999470 ) ) ;
#5189=CARTESIAN_POINT ( 'NONE',  ( 0.6125012097518164333, -100.6644468680149060, -16.75904295264657762 ) ) ;
#5190=CARTESIAN_POINT ( 'NONE',  ( -4.643931556212963052, -95.55433702412769037, 22.13027306510061720 ) ) ;
#5198=CARTESIAN_POINT ( 'NONE',  ( 23.77207126295173367, -92.72059904818672749, -19.10860135063087384 ) ) ;
#5209=CIRCLE ( 'NONE', #12617, 16.00000000000000000 ) ;
#5212=CIRCLE ( 'NONE', #7562, 9.999999999999996447 ) ;
#5213=CARTESIAN_POINT ( 'NONE',  ( 10.51051219959999905, -93.03281165500000327, 27.57047580710000290 ) ) ;
#5215=ADVANCED_FACE ( 'NONE', ( #17364 ), #28451, .T. ) ;
#5217=ORIENTED_EDGE ( 'NONE', *, *, #27565, .T. ) ;
#5220=DIRECTION ( 'NONE',  ( 1.000000000000000000, 0.000000000000000000, 0.000000000000000000 ) ) ;
#5224=CARTESIAN_POINT ( 'NONE',  ( -6.547105968080000338, -97.18075703250001141, -19.87372873440000376 ) ) ;
#5225=CARTESIAN_POINT ( 'NONE',  ( -12.22512452690000018, -101.6484611540000031, -9.528710841509999696 ) ) ;
#5230=CARTESIAN_POINT ( 'NONE',  ( -15.72691182720000214, -100.6651030490000096, 2.680982550860000035 ) ) ;
#5237=CARTESIAN_POINT ( 'NONE',  ( 24.18486883099999929, -92.81180222670001001, -12.79052883029999954 ) ) ;
#5240=CARTESIAN_POINT ( 'NONE',  ( -9.548240116189999682, -93.74526857300000415, -23.19355367660000056 ) ) ;
#5244=CARTESIAN_POINT ( 'NONE',  ( 16.03248225524879444, -100.8945630371651276, 4.256357661172395446 ) ) ;
#5247=B_SPLINE_SURFACE_WITH_KNOTS ( 'NONE', 5, 5, ( 
 ( #7603, #23313, #18809, #19080, #27701, #5257, #3089, #11940, #27964 ),
 ( #8002, #7865, #3496, #16467, #23586, #5398, #3630, #3221, #769 ),
 ( #18942, #23040, #9614, #1192, #7739, #25501, #18515, #12354, #20994 ),
 ( #5532, #20712, #14552, #27408, #21264, #7457, #16316, #20853, #913 ),
 ( #9754, #3358, #18667, #14282, #23178, #12225, #23457, #21133, #12082 ),
 ( #10028, #1056, #27825, #16746, #25643, #5672, #1318, #10160, #28373 ) ),
 .UNSPECIFIED., .F., .F., .F.,
 ( 6, 6 ),
 ( 6, 3, 6 ),
 ( 4.816191416739999731, 6.255250589900000158 ),
 ( 0.000000000000000000, 0.2500000000000000000, 0.5000000000000000000 ),
 .UNSPECIFIED. ) ;
#5250=CARTESIAN_POINT ( 'NONE',  ( 6.173817828315791623, -93.45278262996737340, 26.74719681978107744 ) ) ;
#5254=B_SPLINE_CURVE_WITH_KNOTS ( 'NONE', 5,
 ( #25082, #11947, #9476, #7306, #7745, #5117, #21141, #918, #25648 ),
 .UNSPECIFIED., .F., .F.,
 ( 6, 3, 6 ),
 ( 0.000000000000000000, 0.5000000000000000000, 1.000000000000000000 ),
 .UNSPECIFIED. ) ;
#5257=CARTESIAN_POINT ( 'NONE',  ( -5.582121642149999730, -100.8816835080000089, 14.77497840909999915 ) ) ;
#5261=DIRECTION ( 'NONE',  ( -0.000000000000000000, 1.000000000000000000, 0.000000000000000000 ) ) ;
#5263=CARTESIAN_POINT ( 'NONE',  ( -13.36030084967533682, -101.4218099524540264, -9.110383877951878873 ) ) ;
#5268=CARTESIAN_POINT ( 'NONE',  ( 12.53707620288065350, -93.63284908669999140, -21.72543824449705596 ) ) ;
#5269=CARTESIAN_POINT ( 'NONE',  ( -20.02788083190000279, -92.50000000000000000, 20.80461572599999798 ) ) ;
#5271=ORIENTED_EDGE ( 'NONE', *, *, #22051, .T. ) ;
#5274=CARTESIAN_POINT ( 'NONE',  ( -12.23011636260000046, -101.1292389600000092, -9.532601661500001100 ) ) ;
#5276=ORIENTED_EDGE ( 'NONE', *, *, #6404, .F. ) ;
#5277=CARTESIAN_POINT ( 'NONE',  ( -18.25187102170000131, -97.32059399370000108, 11.22053352470000043 ) ) ;
#5282=EDGE_CURVE ( 'NONE', #25457, #1700, #25762, .T. ) ;
#5285=EDGE_CURVE ( 'NONE', #2397, #22989, #3250, .T. ) ;
#5288=VERTEX_POINT ( 'NONE', #25246 ) ;
#5296=CARTESIAN_POINT ( 'NONE',  ( -13.41619584950000110, -101.2306315440000049, -9.103915625870000028 ) ) ;
#5301=CARTESIAN_POINT ( 'NONE',  ( 7.555516771499999784, -101.3253988449999952, 13.99788120350000042 ) ) ;
#5305=CARTESIAN_POINT ( 'NONE',  ( 11.56404080679999957, -97.23151480800000002, -17.97423634720000152 ) ) ;
#5308=CARTESIAN_POINT ( 'NONE',  ( 11.91199879370000048, -101.3256027080000052, -10.54214213689999902 ) ) ;
#5310=CARTESIAN_POINT ( 'NONE',  ( -18.38790699489164737, -92.50638022835023833, 24.33425043882840200 ) ) ;
#5311=AXIS2_PLACEMENT_3D ( 'NONE', #11779, #26956, #752 ) ;
#5313=CARTESIAN_POINT ( 'NONE',  ( 11.91128644723943708, -101.5839620086842814, -10.75510067162974970 ) ) ;
#5321=CARTESIAN_POINT ( 'NONE',  ( 6.946147887829999590, -101.6311724339999927, 14.42877099100000216 ) ) ;
#5323=VECTOR ( 'NONE', #2324, 1000.000000000000000 ) ;
#5329=CARTESIAN_POINT ( 'NONE',  ( -20.15695820925639126, -93.11247489648164333, -20.71965102693426530 ) ) ;
#5334=DIRECTION ( 'NONE',  ( 0.000000000000000000, 1.000000000000000000, 0.000000000000000000 ) ) ;
#5337=FACE_OUTER_BOUND ( 'NONE', #15838, .T. ) ;
#5338=CARTESIAN_POINT ( 'NONE',  ( 0.5980344247127714619, -100.4211561361990732, -16.95372977634908906 ) ) ;
#5358=CARTESIAN_POINT ( 'NONE',  ( 0.000000000000000000, -92.50000000000000000, 0.000000000000000000 ) ) ;
#5359=CARTESIAN_POINT ( 'NONE',  ( 4.140575906510000515, -93.29998627720000570, 25.57099462040000049 ) ) ;
#5360=ORIENTED_EDGE ( 'NONE', *, *, #18023, .T. ) ;
#5361=CARTESIAN_POINT ( 'NONE',  ( -11.17102488801581650, -94.77696260184704613, -20.89251602398021035 ) ) ;
#5362=CARTESIAN_POINT ( 'NONE',  ( -29.24808533433442648, -93.02765837721192099, 4.206566995128039999 ) ) ;
#5367=DIRECTION ( 'NONE',  ( 1.000000000000000000, 0.000000000000000000, 0.000000000000000000 ) ) ;
#5376=CARTESIAN_POINT ( 'NONE',  ( -15.39899069939999876, -101.1262888790000005, 3.404061698440000061 ) ) ;
#5382=CARTESIAN_POINT ( 'NONE',  ( -7.900916432368809694, -99.99762666408553002, 15.39651926382340363 ) ) ;
#5388=CARTESIAN_POINT ( 'NONE',  ( 16.00294200327352101, -100.9364580239705873, 4.239096016115913024 ) ) ;
#5397=EDGE_LOOP ( 'NONE', ( #15207, #3040, #4793, #16185, #21265, #1792, #20713, #21293, #23823, #24151, #2363, #4560, #7405, #7400, #7676, #6927, #13790, #20899, #446, #20060, #124, #14419 ) ) ;
#5398=CARTESIAN_POINT ( 'NONE',  ( -5.644564482089999835, -100.9763228559999959, 14.63128291989999852 ) ) ;
#5399=ORIENTED_EDGE ( 'NONE', *, *, #17076, .F. ) ;
#5402=ADVANCED_FACE ( 'NONE', ( #5129 ), #21246, .T. ) ;
#5406=CARTESIAN_POINT ( 'NONE',  ( 13.12517053680000068, -93.00000000000000000, 27.53143473160000099 ) ) ;
#5409=ORIENTED_EDGE ( 'NONE', *, *, #21080, .F. ) ;
#5410=CARTESIAN_POINT ( 'NONE',  ( 12.43265749360000072, -93.67869433820000324, -21.69433720420000000 ) ) ;
#5412=CARTESIAN_POINT ( 'NONE',  ( -0.1723943457659999900, -101.6484611540000031, -15.49904126680000083 ) ) ;
#5414=CIRCLE ( 'NONE', #23545, 20.64285714289999873 ) ;
#5415=CARTESIAN_POINT ( 'NONE',  ( 29.72661487340210229, -92.83160374581348151, 6.824835530513863269 ) ) ;
#5416=CARTESIAN_POINT ( 'NONE',  ( -15.55828293390000105, -101.6484611540000031, 3.733608462140000306 ) ) ;
#5429=CARTESIAN_POINT ( 'NONE',  ( 19.83536304030000252, -94.71481430550001335, 14.13922876900000070 ) ) ;
#5432=FACE_OUTER_BOUND ( 'NONE', #13858, .T. ) ;
#5433=CARTESIAN_POINT ( 'NONE',  ( -17.11893731760000037, -92.49999999210000112, -23.95273848429999930 ) ) ;
#5434=CARTESIAN_POINT ( 'NONE',  ( -7.720628919050000150, -100.8088109309999965, 14.63797111400000084 ) ) ;
#5435=DIRECTION ( 'NONE',  ( 1.000000000000000000, 0.000000000000000000, 0.000000000000000000 ) ) ;
#5436=DIRECTION ( 'NONE',  ( 1.000000000000000000, 0.000000000000000000, 0.000000000000000000 ) ) ;
#5437=CARTESIAN_POINT ( 'NONE',  ( 7.594361522519999852, -101.6484612250000055, 14.08281941390000114 ) ) ;
#5439=EDGE_CURVE ( 'NONE', #7753, #13918, #15128, .T. ) ;
#5443=CARTESIAN_POINT ( 'NONE',  ( 11.11271058390000022, -96.95622423819999369, -17.69897580199999965 ) ) ;
#5453=CARTESIAN_POINT ( 'NONE',  ( 11.89727022614212615, -101.5620304352158314, -10.79529442988603272 ) ) ;
#5455=CARTESIAN_POINT ( 'NONE',  ( 13.84987421219491921, -98.08323781429143651, 15.06242402452379636 ) ) ;
#5458=CARTESIAN_POINT ( 'NONE',  ( 6.731493086280000426, -101.1411470200000053, 13.83935196010000013 ) ) ;
#5463=CARTESIAN_POINT ( 'NONE',  ( 24.31651070795704683, -94.36683344927989481, -3.632850094172810795 ) ) ;
#5466=EDGE_LOOP ( 'NONE', ( #17632, #23870, #8907, #2180 ) ) ;
#5467=CARTESIAN_POINT ( 'NONE',  ( -5.969238273050000210, -101.2530993000000024, 13.97222956270000083 ) ) ;
#5471=EDGE_LOOP ( 'NONE', ( #15527, #2597, #24869, #16148 ) ) ;
#5473=CARTESIAN_POINT ( 'NONE',  ( 0.6068588990009703421, -100.7538407677319583, -16.68821395358974158 ) ) ;
#5474=CARTESIAN_POINT ( 'NONE',  ( 6.744238910220000882, -101.2530993010000060, 13.61507422070000040 ) ) ;
#5475=CARTESIAN_POINT ( 'NONE',  ( 3.166345171159999694, -111.0000000000000000, -25.30265318609999881 ) ) ;
#5476=CARTESIAN_POINT ( 'NONE',  ( -12.56240048859999803, -94.54647010769998872, -21.54391703350000142 ) ) ;
#5483=CARTESIAN_POINT ( 'NONE',  ( 12.82422680459999853, -94.98812477769999418, -19.93894967960000386 ) ) ;
#5484=B_SPLINE_SURFACE_WITH_KNOTS ( 'NONE', 5, 5, ( 
 ( #14087, #5865, #9413, #19275, #3039, #10223, #23645, #13939, #21462 ),
 ( #22841, #20803, #2885, #27877, #11742, #18998, #20658, #9567, #857 ),
 ( #18466, #12408, #19135, #9701, #5729, #14615, #23517, #21320, #28024 ),
 ( #8322, #22179, #6288, #15154, #24064, #21602, #8469, #5998, #3826 ),
 ( #1658, #28707, #26266, #4403, #4103, #12973, #11062, #17225, #4252 ),
 ( #24362, #17664, #8747, #10923, #24218, #21886, #21739, #10777, #1789 ) ),
 .UNSPECIFIED., .F., .F., .F.,
 ( 6, 6 ),
 ( 6, 3, 6 ),
 ( 4.816191416749999732, 6.255250589900000158 ),
 ( 0.000000000000000000, 0.2500000000000000000, 0.5000000000000000000 ),
 .UNSPECIFIED. ) ;
#5493=CARTESIAN_POINT ( 'NONE',  ( -28.52512532269999923, -92.54030566109999256, 3.253864596379999696 ) ) ;
#5511=CARTESIAN_POINT ( 'NONE',  ( -16.13804302950000036, -100.4011261050000030, 2.780960711030000088 ) ) ;
#5524=ORIENTED_EDGE ( 'NONE', *, *, #18963, .T. ) ;
#5525=CIRCLE ( 'NONE', #3647, 20.64285714289999873 ) ;
#5532=CARTESIAN_POINT ( 'NONE',  ( -6.058780266770000367, -101.6095085860000040, 14.84092105570000086 ) ) ;
#5533=ORIENTED_EDGE ( 'NONE', *, *, #19654, .F. ) ;
#5537=CIRCLE ( 'NONE', #21361, 0.4999999999999983902 ) ;
#5544=ORIENTED_EDGE ( 'NONE', *, *, #19790, .F. ) ;
#5550=CARTESIAN_POINT ( 'NONE',  ( -20.41940881060000024, -94.07621218059999535, 14.28684394100000077 ) ) ;
#5554=CARTESIAN_POINT ( 'NONE',  ( 29.70837229499504772, -92.96960399592401814, 6.903811671076394596 ) ) ;
#5558=CARTESIAN_POINT ( 'NONE',  ( -7.879410208250000380, -99.92967571559999840, 15.46934584979999983 ) ) ;
#5562=DIRECTION ( 'NONE',  ( 0.000000000000000000, 0.000000000000000000, 1.000000000000000000 ) ) ;
#5572=CARTESIAN_POINT ( 'NONE',  ( -13.14571786560000000, -100.8733988930000010, -8.628954981190000595 ) ) ;
#5575=CARTESIAN_POINT ( 'NONE',  ( -7.722863872719999634, -100.5717442099999914, 14.38966742470000071 ) ) ;
#5578=CARTESIAN_POINT ( 'NONE',  ( 7.320076657800000497, -101.1409265030000029, 13.53711875870000192 ) ) ;
#5579=ORIENTED_EDGE ( 'NONE', *, *, #17076, .T. ) ;
#5581=CARTESIAN_POINT ( 'NONE',  ( -27.06659278359999732, -93.14733690340000294, -4.203927835110000011 ) ) ;
#5582=DIRECTION ( 'NONE',  ( 0.000000000000000000, -1.000000000000000000, 0.000000000000000000 ) ) ;
#5585=CARTESIAN_POINT ( 'NONE',  ( 11.67565778989999892, -101.1292389600000092, -10.20417835260000139 ) ) ;
#5586=CARTESIAN_POINT ( 'NONE',  ( -17.54428591559999973, -94.59275927410000406, 16.07756161280000029 ) ) ;
#5590=FACE_OUTER_BOUND ( 'NONE', #25541, .T. ) ;
#5591=B_SPLINE_CURVE_WITH_KNOTS ( 'NONE', 5,
 ( #24838, #18430, #679, #9379, #16081, #12137, #5015, #974, #9814, #11704, #16527, #825 ),
 .UNSPECIFIED., .F., .F.,
 ( 6, 3, 3, 6 ),
 ( -7.896981424030000696, -6.690827956829999756, -5.319894352600000431, -3.365447998909999683 ),
 .UNSPECIFIED. ) ;
#5594=CARTESIAN_POINT ( 'NONE',  ( 13.67893538235999529, -98.17437103743534976, 15.05775980708956219 ) ) ;
#5600=CARTESIAN_POINT ( 'NONE',  ( -11.73664997740000082, -94.54719592029999831, -20.76900810619999760 ) ) ;
#5602=CARTESIAN_POINT ( 'NONE',  ( 6.019093083229999586, -92.50000000000000000, 29.30685818879999971 ) ) ;
#5603=ADVANCED_FACE ( 'NONE', ( #7820 ), #5761, .T. ) ;
#5606=CARTESIAN_POINT ( 'NONE',  ( -19.96485215072167563, -93.12686943432630926, -20.78016349561067599 ) ) ;
#5607=VECTOR ( 'NONE', #2976, 1000.000000000000000 ) ;
#5609=CARTESIAN_POINT ( 'NONE',  ( -5.774731795730000172, -101.2530993039999885, 14.05532693159999980 ) ) ;
#5611=ORIENTED_EDGE ( 'NONE', *, *, #12604, .T. ) ;
#5613=CARTESIAN_POINT ( 'NONE',  ( 0.5718234277215632488, -100.9364580247160177, -16.54500244008519161 ) ) ;
#5615=CARTESIAN_POINT ( 'NONE',  ( 13.45309085318943687, -92.66191076889870715, 27.37276729370756101 ) ) ;
#5618=CARTESIAN_POINT ( 'NONE',  ( 23.87439762153048761, -92.83865970264375278, -18.98059930716613408 ) ) ;
#5623=AXIS2_PLACEMENT_3D ( 'NONE', #11433, #557, #9402 ) ;
#5627=AXIS2_PLACEMENT_3D ( 'NONE', #24435, #17447, #17149 ) ;
#5628=VERTEX_POINT ( 'NONE', #17410 ) ;
#5634=DIRECTION ( 'NONE',  ( -0.4299718839438681495, 0.000000000000000000, 0.9028422780407223680 ) ) ;
#5640=CIRCLE ( 'NONE', #9355, 0.4999999999999993894 ) ;
#5643=CIRCLE ( 'NONE', #1455, 16.00000000000000000 ) ;
#5648=CARTESIAN_POINT ( 'NONE',  ( -14.79093856799999962, -101.1411468629999888, 4.252364208789999545 ) ) ;
#5649=CARTESIAN_POINT ( 'NONE',  ( -16.73274653779999710, -100.1461833709999922, 3.179024074209999995 ) ) ;
#5652=B_SPLINE_SURFACE_WITH_KNOTS ( 'NONE', 5, 5, ( 
 ( #12388, #19387, #10334, #28265, #28001, #8038 ),
 ( #5842, #23621, #23905, #25950, #19522, #19250 ),
 ( #26090, #6119, #17058, #14859, #28408, #6266 ),
 ( #23762, #15131, #7011, #4517, #13394, #6861 ),
 ( #19949, #19806, #20111, #22298, #22455, #1910 ),
 ( #4379, #10754, #24192, #13546, #179, #13703 ) ),
 .UNSPECIFIED., .F., .F., .F.,
 ( 6, 6 ),
 ( 6, 6 ),
 ( 0.000000000000000000, 11.23209334890000122 ),
 ( 0.000000000000000000, 0.5000000000000000000 ),
 .UNSPECIFIED. ) ;
#5653=ORIENTED_EDGE ( 'NONE', *, *, #3160, .T. ) ;
#5654=DIRECTION ( 'NONE',  ( 1.000000000000000000, 0.000000000000000000, 0.000000000000000000 ) ) ;
#5657=ORIENTED_EDGE ( 'NONE', *, *, #6406, .T. ) ;
#5659=CARTESIAN_POINT ( 'NONE',  ( 14.05983645159999895, -99.53431386179998697, -10.27466725399999881 ) ) ;
#5662=AXIS2_PLACEMENT_3D ( 'NONE', #24920, #20543, #9457 ) ;
#5663=EDGE_CURVE ( 'NONE', #1700, #21528, #24960, .T. ) ;
#5664=B_SPLINE_CURVE_WITH_KNOTS ( 'NONE', 5,
 ( #11651, #14000, #11807, #14151, #630, #26980 ),
 .UNSPECIFIED., .F., .F.,
 ( 6, 6 ),
 ( 0.000000000000000000, 1.000000000000000000 ),
 .UNSPECIFIED. ) ;
#5665=CARTESIAN_POINT ( 'NONE',  ( 6.819379226960565532, -100.4166221066960816, 15.53723975361173082 ) ) ;
#5667=EDGE_CURVE ( 'NONE', #4274, #11243, #18912, .T. ) ;
#5669=CARTESIAN_POINT ( 'NONE',  ( -18.29991037700670731, -98.29443223157012710, 5.167542575955573092 ) ) ;
#5671=CARTESIAN_POINT ( 'NONE',  ( 29.52540666350000365, -92.92146929989999649, 7.168157270950000104 ) ) ;
#5672=CARTESIAN_POINT ( 'NONE',  ( -6.091977122730000360, -101.1292389600000092, 14.25952507679999925 ) ) ;
#5673=ORIENTED_EDGE ( 'NONE', *, *, #5439, .F. ) ;
#5676=DIRECTION ( 'NONE',  ( 1.000000000000000000, 0.000000000000000000, 0.000000000000000000 ) ) ;
#5678=DIRECTION ( 'NONE',  ( 0.000000000000000000, 1.000000000000000000, 0.000000000000000000 ) ) ;
#5682=CARTESIAN_POINT ( 'NONE',  ( -16.86248238029999769, -97.53592492889998766, -10.88383597820000048 ) ) ;
#5683=CARTESIAN_POINT ( 'NONE',  ( 19.83108000150000194, -97.73638926309999420, 2.238875083469999971 ) ) ;
#5684=CARTESIAN_POINT ( 'NONE',  ( -20.44007416299999846, -93.36538189280000211, 16.34753294749999952 ) ) ;
#5685=CARTESIAN_POINT ( 'NONE',  ( 15.94061401059999916, -100.1275643909999928, 4.799433088389999824 ) ) ;
#5691=CARTESIAN_POINT ( 'NONE',  ( 20.58461438809549193, -97.38870237790757756, 1.320766927699984938 ) ) ;
#5693=DIRECTION ( 'NONE',  ( 1.000000000000000000, 0.000000000000000000, 0.000000000000000000 ) ) ;
#5696=CIRCLE ( 'NONE', #21976, 18.64285714289999873 ) ;
#5699=ADVANCED_FACE ( 'NONE', ( #22657 ), #27026, .T. ) ;
#5703=CARTESIAN_POINT ( 'NONE',  ( 19.72731272460000085, -94.57749834670001121, 14.01461188380000067 ) ) ;
#5705=CARTESIAN_POINT ( 'NONE',  ( -12.86848417080000040, -101.1499348409999897, -9.082804019830000186 ) ) ;
#5706=PRODUCT_DEFINITION_SHAPE ( 'NONE', 'NONE',  #1029 ) ;
#5708=ORIENTED_EDGE ( 'NONE', *, *, #8688, .F. ) ;
#5709=CARTESIAN_POINT ( 'NONE',  ( -1.247128410550000011, -101.2306304600000004, -16.16540378150000024 ) ) ;
#5711=CARTESIAN_POINT ( 'NONE',  ( 7.547750227499999909, -101.3256028069999957, 14.00193654699999968 ) ) ;
#5712=ORIENTED_EDGE ( 'NONE', *, *, #12805, .T. ) ;
#5717=VERTEX_POINT ( 'NONE', #4577 ) ;
#5720=CARTESIAN_POINT ( 'NONE',  ( 11.30123137200000016, -101.2530993039999885, -10.15784976960000030 ) ) ;
#5723=CARTESIAN_POINT ( 'NONE',  ( -18.26810282299999955, -94.98812129370000434, 16.32728610020000204 ) ) ;
#5726=CARTESIAN_POINT ( 'NONE',  ( 14.28941763439999946, -101.1889999979999999, -3.575252188409999921 ) ) ;
#5729=CARTESIAN_POINT ( 'NONE',  ( 15.59036279620000087, -101.1042759770000004, 2.486817442600000039 ) ) ;
#5732=ORIENTED_EDGE ( 'NONE', *, *, #18953, .F. ) ;
#5735=CARTESIAN_POINT ( 'NONE',  ( 6.228305304889999228, -100.7707614970000094, 14.58014589510000114 ) ) ;
#5738=CARTESIAN_POINT ( 'NONE',  ( 7.653117467020000397, -101.1929016639999901, 13.21760603179999904 ) ) ;
#5739=CARTESIAN_POINT ( 'NONE',  ( -11.77049225210000039, -94.59276583640000524, -20.68202189790000034 ) ) ;
#5742=B_SPLINE_CURVE_WITH_KNOTS ( 'NONE', 3,
 ( #950, #3259, #12112, #12523 ),
 .UNSPECIFIED., .F., .F.,
 ( 4, 4 ),
 ( -0.1274251584810000004, 0.000000000000000000 ),
 .UNSPECIFIED. ) ;
#5743=CARTESIAN_POINT ( 'NONE',  ( 26.16322034310070421, -93.20709273739696243, -8.388943539576686703 ) ) ;
#5745=CARTESIAN_POINT ( 'NONE',  ( 7.694095999870000036, -93.61368346389998862, -24.10127357489999866 ) ) ;
#5746=VERTEX_POINT ( 'NONE', #18864 ) ;
#5747=CARTESIAN_POINT ( 'NONE',  ( -16.99294773969999994, -99.88067626670000720, 3.462731254189999941 ) ) ;
#5751=CARTESIAN_POINT ( 'NONE',  ( 0.4754459893910686907, -101.1884902310534358, -16.35008640957526183 ) ) ;
#5753=CARTESIAN_POINT ( 'NONE',  ( 6.390838521760000113, -101.2010924020000004, 13.85940160760000062 ) ) ;
#5755=CARTESIAN_POINT ( 'NONE',  ( 13.32851355232033441, -92.72722989462353382, 27.43357149820718632 ) ) ;
#5759=CARTESIAN_POINT ( 'NONE',  ( 18.39097424218846299, -93.63284908709232468, 17.05711033620115558 ) ) ;
#5761=CYLINDRICAL_SURFACE ( 'NONE', #19797, 0.7500000000000004441 ) ;
#5770=DIRECTION ( 'NONE',  ( 0.7175736280288005364, 0.000000000000000000, -0.6964826547428046855 ) ) ;
#5776=CARTESIAN_POINT ( 'NONE',  ( 9.718892398710000435, -111.0000000000000000, 28.91008700340000104 ) ) ;
#5778=ORIENTED_EDGE ( 'NONE', *, *, #5282, .F. ) ;
#5784=CARTESIAN_POINT ( 'NONE',  ( -22.24124310690000073, -94.63960343439998724, -8.291373264160000645 ) ) ;
#5785=CARTESIAN_POINT ( 'NONE',  ( -15.54748971619999942, -100.8069964150000004, 2.643158339580000238 ) ) ;
#5790=CARTESIAN_POINT ( 'NONE',  ( 20.41153474230850051, -98.08323605630401687, -1.437002437402584043 ) ) ;
#5791=CARTESIAN_POINT ( 'NONE',  ( 15.63748056140000209, -101.1889999979999999, 3.386620984279999913 ) ) ;
#5792=EDGE_CURVE ( 'NONE', #1710, #17884, #25603, .T. ) ;
#5794=CARTESIAN_POINT ( 'NONE',  ( -7.109209100094830980, -101.5526869446641456, 14.41623343727262352 ) ) ;
#5801=B_SPLINE_CURVE_WITH_KNOTS ( 'NONE', 3,
 ( #5052, #7251, #9122, #16118, #26781, #2737, #11593, #13942, #9416, #4912, #13791, #126, #18024, #13646, #22246, #15674, #4619, #20351, #20501, #4772, #18324, #572, #25019, #24579, #22555, #24877, #27213, #15826, #20208, #2296 ),
 .UNSPECIFIED., .F., .F.,
 ( 4, 1, 1, 1, 1, 2, 2, 1, 1, 1, 1, 2, 2, 2, 1, 1, 1, 1, 2, 2, 4 ),
 ( 0.000000000000000000, 0.1250000000000730249, 0.1875000000001089129, 0.2187500000001260103, 0.2343750000001336986, 0.2421875000001385003, 0.2500000000001432743, 0.3750000000001741385, 0.4375000000001877942, 0.4687500000001946221, 0.4843750000001973421, 0.4921875000001995071, 0.5000000000002016165, 0.6250000000002247091, 0.6875000000002352563, 0.7187500000002405853, 0.7343750000002452483, 0.7421875000002475797, 0.7460937500002480238, 0.7500000000002483569, 1.000000000000000000 ),
 .UNSPECIFIED. ) ;
#5803=CARTESIAN_POINT ( 'NONE',  ( 6.977121519902694580, -100.1585711159146257, 15.69426428360687709 ) ) ;
#5804=CARTESIAN_POINT ( 'NONE',  ( 11.56318970670437452, -101.1604341566338121, -10.10588458626208208 ) ) ;
#5807=CARTESIAN_POINT ( 'NONE',  ( -18.06240238254229880, -98.56362441878414415, 4.716205741958754416 ) ) ;
#5810=CARTESIAN_POINT ( 'NONE',  ( 27.42310009790000080, -92.79907194240000479, 9.733922945540001592 ) ) ;
#5820=ORIENTED_EDGE ( 'NONE', *, *, #23270, .F. ) ;
#5821=EDGE_CURVE ( 'NONE', #7330, #19526, #5414, .T. ) ;
#5822=CARTESIAN_POINT ( 'NONE',  ( -15.14477094210000097, -98.93445099689999722, -10.94682493010000002 ) ) ;
#5823=CARTESIAN_POINT ( 'NONE',  ( 15.82848316267510747, -101.5902664364219135, 2.618622591423955370 ) ) ;
#5824=CARTESIAN_POINT ( 'NONE',  ( -20.21807458789999856, -92.87437404489999437, 18.51498583080000060 ) ) ;
#5825=CARTESIAN_POINT ( 'NONE',  ( 24.80162329460000237, -92.90721294759998727, -13.73419815169999936 ) ) ;
#5827=CARTESIAN_POINT ( 'NONE',  ( 29.76318999973515034, -92.71619979446128923, 6.663522998223462501 ) ) ;
#5829=VERTEX_POINT ( 'NONE', #11224 ) ;
#5834=CARTESIAN_POINT ( 'NONE',  ( 21.25651707432598414, -96.89152197653719156, 0.6302383136284459564 ) ) ;
#5842=CARTESIAN_POINT ( 'NONE',  ( 10.74632799350000134, -97.93548434830000815, 16.80947664850000223 ) ) ;
#5843=CARTESIAN_POINT ( 'NONE',  ( -15.10670588340000009, -93.09001853929999015, -23.64475874150000223 ) ) ;
#5844=CARTESIAN_POINT ( 'NONE',  ( -8.064919287289999517, -99.61736775859999682, 15.35592295719999889 ) ) ;
#5845=CARTESIAN_POINT ( 'NONE',  ( -2.773446675360000224, -99.97119183019999866, -17.69078287840000030 ) ) ;
#5848=CARTESIAN_POINT ( 'NONE',  ( 7.361150943080000175, -101.1292390549999993, 13.64770487110000019 ) ) ;
#5851=CARTESIAN_POINT ( 'NONE',  ( 13.27227242060828871, -100.9616911410478934, -9.861731524377153946 ) ) ;
#5852=CARTESIAN_POINT ( 'NONE',  ( -25.52527845280000207, -93.36531860699999186, -5.788118625400000106 ) ) ;
#5855=VERTEX_POINT ( 'NONE', #24657 ) ;
#5859=CARTESIAN_POINT ( 'NONE',  ( -18.51202076211952630, -92.49999999999998579, 24.23973938018714946 ) ) ;
#5860=ORIENTED_EDGE ( 'NONE', *, *, #12172, .T. ) ;
#5863=CARTESIAN_POINT ( 'NONE',  ( 0.02056460011280000083, -101.1180794200000008, -15.51940904669999988 ) ) ;
#5865=CARTESIAN_POINT ( 'NONE',  ( 16.03761573839999954, -101.2306315440000049, 2.381275335019999773 ) ) ;
#5869=CARTESIAN_POINT ( 'NONE',  ( 6.682224820120000075, -100.4071172650000108, 15.40394232580000100 ) ) ;
#5870=CARTESIAN_POINT ( 'NONE',  ( 15.12572900610000026, -101.1180794200000008, 3.473442398169999557 ) ) ;
#5872=CARTESIAN_POINT ( 'NONE',  ( 5.648478490313273426, -92.54687141712493315, -29.97239971131430636 ) ) ;
#5874=CARTESIAN_POINT ( 'NONE',  ( -6.520248143609999936, -97.93128678229999196, 18.90965181079999979 ) ) ;
#5876=CARTESIAN_POINT ( 'NONE',  ( 7.615531154710000195, -93.65023553240000354, -24.05380218500000211 ) ) ;
#5880=CARTESIAN_POINT ( 'NONE',  ( -6.950015043800000569, -101.6311724339999927, 14.42690866679999928 ) ) ;
#5886=ADVANCED_FACE ( 'NONE', ( #26847 ), #22623, .T. ) ;
#5887=CARTESIAN_POINT ( 'NONE',  ( -1.271820802479999957, -100.9405348700000076, -15.89396400309999891 ) ) ;
#5905=CARTESIAN_POINT ( 'NONE',  ( 9.015422770486624771, -94.52293547164840959, -22.16844695295810297 ) ) ;
#5909=CYLINDRICAL_SURFACE ( 'NONE', #17635, 10.99999999999999822 ) ;
#5917=DIRECTION ( 'NONE',  ( 0.000000000000000000, 1.000000000000000000, 0.000000000000000000 ) ) ;
#5921=CARTESIAN_POINT ( 'NONE',  ( -11.84587943579999880, -100.7776802639999971, -10.46823333549999901 ) ) ;
#5924=VERTEX_POINT ( 'NONE', #14167 ) ;
#5928=ORIENTED_EDGE ( 'NONE', *, *, #20134, .F. ) ;
#5931=CARTESIAN_POINT ( 'NONE',  ( 6.827177860526931319, -100.4010812938127231, 15.54740832690005625 ) ) ;
#5934=ORIENTED_EDGE ( 'NONE', *, *, #21545, .F. ) ;
#5936=CARTESIAN_POINT ( 'NONE',  ( -18.87175863199883707, -97.59429761047931606, 6.378058639867395740 ) ) ;
#5938=CARTESIAN_POINT ( 'NONE',  ( 28.52646387189999899, -92.76004106530000115, 8.498496893989999634 ) ) ;
#5943=CARTESIAN_POINT ( 'NONE',  ( 14.05983645159999895, -99.53431386179998697, -10.27466725399999881 ) ) ;
#5947=CARTESIAN_POINT ( 'NONE',  ( -15.25169713729999899, -93.03108158919999937, 25.12655145109999921 ) ) ;
#5949=FACE_OUTER_BOUND ( 'NONE', #2897, .T. ) ;
#5950=CARTESIAN_POINT ( 'NONE',  ( 13.02419203620000054, -101.1191090859999946, -9.808337647929999292 ) ) ;
#5953=CARTESIAN_POINT ( 'NONE',  ( 24.74320438849999704, -92.87863185420000889, -15.37964689979999910 ) ) ;
#5967=ORIENTED_EDGE ( 'NONE', *, *, #13761, .T. ) ;
#5971=DIRECTION ( 'NONE',  ( -0.000000000000000000, 1.000000000000000000, 0.000000000000000000 ) ) ;
#5973=ORIENTED_EDGE ( 'NONE', *, *, #9868, .F. ) ;
#5974=CARTESIAN_POINT ( 'NONE',  ( -12.62850920960000067, -101.1292389529999980, -8.999250585949999603 ) ) ;
#5975=EDGE_CURVE ( 'NONE', #15187, #3937, #9493, .T. ) ;
#5978=CARTESIAN_POINT ( 'NONE',  ( -8.306762876789999694, -99.70407914540000149, 15.05683357740000083 ) ) ;
#5979=ORIENTED_EDGE ( 'NONE', *, *, #20948, .F. ) ;
#5983=FACE_OUTER_BOUND ( 'NONE', #17671, .T. ) ;
#5985=CARTESIAN_POINT ( 'NONE',  ( 13.32384360391719902, -100.8945630383305172, -9.880903774112189453 ) ) ;
#5986=CARTESIAN_POINT ( 'NONE',  ( -23.86455928470000032, -93.85307999919999133, -7.129255525669999649 ) ) ;
#5998=CARTESIAN_POINT ( 'NONE',  ( 15.14287553800000019, -101.1516803200000112, 2.366416619579999825 ) ) ;
#6004=CARTESIAN_POINT ( 'NONE',  ( 6.850256061619999670, -100.3063911739999980, 15.61955539839999929 ) ) ;
#6005=CARTESIAN_POINT ( 'NONE',  ( 15.54628162380000056, -101.3256027139999986, 3.366869961439999948 ) ) ;
#6006=EDGE_CURVE ( 'NONE', #19985, #11556, #10889, .T. ) ;
#6012=CARTESIAN_POINT ( 'NONE',  ( 8.990098085549998785, -94.64125147560000073, -23.28616752739999995 ) ) ;
#6015=CARTESIAN_POINT ( 'NONE',  ( -6.477090623329999630, -101.1848541609999899, 13.84155909140000063 ) ) ;
#6018=CARTESIAN_POINT ( 'NONE',  ( -5.298192075760000286, -100.9197081840000010, 14.69882727599999939 ) ) ;
#6021=CARTESIAN_POINT ( 'NONE',  ( -1.034434536250000036, -101.3350617309999961, -15.98868234950000300 ) ) ;
#6023=CARTESIAN_POINT ( 'NONE',  ( -17.12548553040000243, -99.53431416519998720, 3.156821174210000081 ) ) ;
#6027=CARTESIAN_POINT ( 'NONE',  ( -15.42268960139999834, -101.6484611540000031, 4.259183661159999801 ) ) ;
#6029=DIRECTION ( 'NONE',  ( 1.000000000000000000, 0.000000000000000000, 0.000000000000000000 ) ) ;
#6038=CARTESIAN_POINT ( 'NONE',  ( -28.92127267589999917, -92.49999926799999628, 4.832872623250000110 ) ) ;
#6044=ORIENTED_EDGE ( 'NONE', *, *, #16592, .F. ) ;
#6053=AXIS2_PLACEMENT_3D ( 'NONE', #621, #18941, #27824 ) ;
#6055=CARTESIAN_POINT ( 'NONE',  ( -14.77445022520000073, -101.2530993010000060, 3.545507728200000042 ) ) ;
#6061=CARTESIAN_POINT ( 'NONE',  ( -12.47865851810000137, -101.3852859389999992, -10.00366179029999891 ) ) ;
#6065=PLANE ( 'NONE',  #5627 ) ;
#6069=EDGE_CURVE ( 'NONE', #11541, #21210, #13345, .T. ) ;
#6071=CARTESIAN_POINT ( 'NONE',  ( 6.663898719022744110, -101.1742791179282648, 14.95015922851185586 ) ) ;
#6076=EDGE_CURVE ( 'NONE', #8673, #25599, #22394, .T. ) ;
#6081=CARTESIAN_POINT ( 'NONE',  ( 29.24515378159999912, -92.51542729400000553, 6.970541694669999622 ) ) ;
#6088=CARTESIAN_POINT ( 'NONE',  ( -22.03785038180000200, -92.91851489729999969, -20.07776381180000058 ) ) ;
#6091=CARTESIAN_POINT ( 'NONE',  ( -16.93606078800000247, -97.83383802270000729, -10.57851684799999958 ) ) ;
#6092=CARTESIAN_POINT ( 'NONE',  ( 13.68838860480000186, -100.0496341300000154, -9.933239034620001462 ) ) ;
#6095=CARTESIAN_POINT ( 'NONE',  ( 24.85836157880000030, -93.07693985719998864, -13.75204276130000025 ) ) ;
#6096=ORIENTED_EDGE ( 'NONE', *, *, #21080, .T. ) ;
#6101=AXIS2_PLACEMENT_3D ( 'NONE', #1314, #1593, #15232 ) ;
#6104=DIRECTION ( 'NONE',  ( 1.000000000000000000, 0.000000000000000000, 0.000000000000000000 ) ) ;
#6118=CIRCLE ( 'NONE', #104, 30.50000000000000000 ) ;
#6119=CARTESIAN_POINT ( 'NONE',  ( 12.10964400579999811, -97.08998106820000373, 17.02756156720000291 ) ) ;
#6120=CARTESIAN_POINT ( 'NONE',  ( -13.12430390699999982, -92.94830164210000589, -23.71756087949999880 ) ) ;
#6121=CARTESIAN_POINT ( 'NONE',  ( -8.158623819759998952, -99.55609327400000552, 15.35276792370000010 ) ) ;
#6122=CARTESIAN_POINT ( 'NONE',  ( -2.925413340589999578, -99.61199057899999332, -17.15801633579999930 ) ) ;
#6124=CARTESIAN_POINT ( 'NONE',  ( -29.73766983855969315, -92.80442066020916059, 6.776535763705393123 ) ) ;
#6135=CARTESIAN_POINT ( 'NONE',  ( -17.74112986619999788, -94.52292883270000345, 16.06143330240000111 ) ) ;
#6136=CARTESIAN_POINT ( 'NONE',  ( 27.23269985219999967, -92.50000000000000000, -12.38957130830000075 ) ) ;
#6143=ADVANCED_FACE ( 'NONE', ( #28252 ), #14307, .T. ) ;
#6146=TOROIDAL_SURFACE ( 'NONE', #22454, 15.50000000000000000, 0.5000000000000000000 ) ;
#6148=EDGE_CURVE ( 'NONE', #22871, #25977, #168, .T. ) ;
#6149=CARTESIAN_POINT ( 'NONE',  ( 6.634569963610000620, -99.72202992580000114, 15.83960876509999949 ) ) ;
#6150=CARTESIAN_POINT ( 'NONE',  ( 14.82033914870000046, -101.2010924020000004, 3.644636806539999885 ) ) ;
#6151=CARTESIAN_POINT ( 'NONE',  ( -3.451442281954444802, -95.36087493701890594, 22.97937161173546272 ) ) ;
#6153=CARTESIAN_POINT ( 'NONE',  ( 5.719937426361796362, -92.53708507728568122, -29.95886813200712595 ) ) ;
#6156=CARTESIAN_POINT ( 'NONE',  ( 1.896867888589999884, -92.62399497440000573, -29.61563552290000345 ) ) ;
#6162=CIRCLE ( 'NONE', #24328, 5.000000000000000888 ) ;
#6166=CARTESIAN_POINT ( 'NONE',  ( 0.7331063123750001242, -99.53431386179998697, -17.39857302659999760 ) ) ;
#6168=CARTESIAN_POINT ( 'NONE',  ( 10.30088935743342127, -93.33134965530122429, -24.92783432923098630 ) ) ;
#6171=CARTESIAN_POINT ( 'NONE',  ( 12.94734957360000038, -94.70873790539999959, -19.84316983170000270 ) ) ;
#6172=CARTESIAN_POINT ( 'NONE',  ( 15.18880477729999967, -100.8685038539999965, 4.097255861100000729 ) ) ;
#6179=CARTESIAN_POINT ( 'NONE',  ( -11.32307664120000013, -93.00000000000000000, 9.421136869679999748 ) ) ;
#6180=DIRECTION ( 'NONE',  ( -0.4740167705367956952, 0.000000000000000000, -0.8805158154456209640 ) ) ;
#6194=DIRECTION ( 'NONE',  ( 0.000000000000000000, 1.000000000000000000, 0.000000000000000000 ) ) ;
#6199=DIRECTION ( 'NONE',  ( 0.000000000000000000, -1.000000000000000000, 0.000000000000000000 ) ) ;
#6200=ORIENTED_EDGE ( 'NONE', *, *, #7382, .T. ) ;
#6207=EDGE_CURVE ( 'NONE', #26488, #16504, #4690, .T. ) ;
#6208=CARTESIAN_POINT ( 'NONE',  ( -15.55828293380000105, -101.6484611540000031, 3.733608462300000319 ) ) ;
#6209=CARTESIAN_POINT ( 'NONE',  ( -14.95416558133042173, -99.82487968003415801, -8.244819971624391286 ) ) ;
#6213=CARTESIAN_POINT ( 'NONE',  ( -12.01041538379999984, -101.0151300849999814, -10.01510942600000043 ) ) ;
#6214=EDGE_CURVE ( 'NONE', #17152, #23549, #23128, .T. ) ;
#6216=CARTESIAN_POINT ( 'NONE',  ( -7.191796251969473808, -101.5026031440308287, 14.41852686845345133 ) ) ;
#6224=CARTESIAN_POINT ( 'NONE',  ( 6.678222761480453684, -101.2637735885552104, 14.86716957882814683 ) ) ;
#6226=ORIENTED_EDGE ( 'NONE', *, *, #21230, .T. ) ;
#6227=CARTESIAN_POINT ( 'NONE',  ( -19.26257329162280385, -97.05447415508082543, 7.349808109310738580 ) ) ;
#6231=CYLINDRICAL_SURFACE ( 'NONE', #23730, 0.7499999999999997780 ) ;
#6238=CARTESIAN_POINT ( 'NONE',  ( -20.48397077079999917, -92.79907188619999658, -20.66839783129999830 ) ) ;
#6242=CARTESIAN_POINT ( 'NONE',  ( -13.32814101110000138, -99.92967428129999519, -11.12411402770000102 ) ) ;
#6244=CARTESIAN_POINT ( 'NONE',  ( 13.67037274660000001, -100.1981337080000003, -10.07712178240000078 ) ) ;
#6247=CARTESIAN_POINT ( 'NONE',  ( 29.76435817172988152, -92.71346081468161060, 6.658302562895561216 ) ) ;
#6249=ORIENTED_EDGE ( 'NONE', *, *, #27637, .F. ) ;
#6251=DIRECTION ( 'NONE',  ( 0.4794255386042036715, 0.000000000000000000, 0.8775825618903724257 ) ) ;
#6253=DIRECTION ( 'NONE',  ( -0.004337301922959033856, 0.000000000000000000, -0.9999905938617769108 ) ) ;
#6254=CARTESIAN_POINT ( 'NONE',  ( -0.5088921683643864435, -92.58347372262090857, -30.49575523020497769 ) ) ;
#6257=ORIENTED_EDGE ( 'NONE', *, *, #27562, .T. ) ;
#6258=B_SPLINE_CURVE_WITH_KNOTS ( 'NONE', 3,
 ( #23962, #15485, #6773, #1972, #3995, #21774, #12856, #10668, #10816, #8643, #17548, #26439, #19393, #24049, #23632, #12814, #28565, #21871, #1774, #6417, #28420, #21586, #23501, #26100, #12957, #10764, #19533, #25829, #5985, #12532, #10480, #28275, #17503, #21307, #5851, #15000, #19120, #19258, #8308, #8600, #8454, #17357, #14733, #28010, #21724, #3671, #26388, #1505, #3540, #14864, #12395, #23914, #10617, #16937, #1358, #3951, #1644, #12675, #17209, #10207 ),
 .UNSPECIFIED., .F., .F.,
 ( 4, 2, 1, 1, 2, 2, 2, 2, 1, 1, 2, 2, 2, 2, 2, 2, 2, 1, 1, 2, 2, 2, 2, 1, 2, 2, 2, 1, 2, 2, 2, 2, 2, 4 ),
 ( 0.000000000000000000, 0.06249999999994744482, 0.09374999999992050803, 0.1093749999999064221, 0.1171874999998935712, 0.1249999999998807343, 0.1874999999997902789, 0.2187499999997453703, 0.2343749999997233602, 0.2421874999997184474, 0.2460937499997155331, 0.2499999999997126465, 0.3124999999998161471, 0.3437499999998687716, 0.3749999999999213407, 0.4375000000000253131, 0.4687500000000772715, 0.4843750000001035283, 0.4921875000001249001, 0.4960937500001271760, 0.5000000000001294520, 0.5625000000001711964, 0.5937500000001925127, 0.6093750000002039480, 0.6171875000002032818, 0.6250000000002027267, 0.6875000000001446621, 0.7187500000001210143, 0.7343750000001157963, 0.7500000000001104672, 0.8125000000000816014, 0.8437500000000671685, 0.8750000000000528466, 1.000000000000000000 ),
 .UNSPECIFIED. ) ;
#6262=EDGE_LOOP ( 'NONE', ( #18955, #25239, #15732, #4925 ) ) ;
#6264=LINE ( 'NONE', #4376, #21405 ) ;
#6266=CARTESIAN_POINT ( 'NONE',  ( 11.93184982500000046, -96.79176330629999825, 17.27990385200000034 ) ) ;
#6272=CARTESIAN_POINT ( 'NONE',  ( -29.62499822415610851, -92.59055325464531450, 7.253245202836821726 ) ) ;
#6278=CARTESIAN_POINT ( 'NONE',  ( -16.65233384409999928, -100.4382163219999882, 3.162646594119999932 ) ) ;
#6282=CARTESIAN_POINT ( 'NONE',  ( -17.71931456970000340, -93.56364925920000530, 19.41824640629999621 ) ) ;
#6283=DIRECTION ( 'NONE',  ( -0.6321469351840500739, 0.000000000000000000, -0.7748485350940611527 ) ) ;
#6285=DIRECTION ( 'NONE',  ( 1.000000000000000000, 0.000000000000000000, 0.000000000000000000 ) ) ;
#6286=CARTESIAN_POINT ( 'NONE',  ( 0.6147020776099999528, -100.8685038539999965, -15.71971493089999861 ) ) ;
#6288=CARTESIAN_POINT ( 'NONE',  ( 15.76529576789999965, -101.3957169669999985, 2.649641455589999861 ) ) ;
#6292=CARTESIAN_POINT ( 'NONE',  ( 6.278326372410000467, -101.0403179300000005, 14.13892092110000043 ) ) ;
#6293=CARTESIAN_POINT ( 'NONE',  ( 15.15499494600000041, -101.1292389600000092, 3.282128709870000272 ) ) ;
#6296=EDGE_CURVE ( 'NONE', #23549, #4293, #28708, .T. ) ;
#6299=CARTESIAN_POINT ( 'NONE',  ( -5.860729663480000795, -96.53848370209999530, 20.54377699719999839 ) ) ;
#6301=CARTESIAN_POINT ( 'NONE',  ( 4.670288045889999573, -92.76550115769998683, -27.85728039249999810 ) ) ;
#6302=ADVANCED_FACE ( 'NONE', ( #4210 ), #20096, .F. ) ;
#6305=DIRECTION ( 'NONE',  ( 0.000000000000000000, 1.000000000000000000, 0.000000000000000000 ) ) ;
#6312=CARTESIAN_POINT ( 'NONE',  ( 23.58655530659999755, -94.70873790539999959, -2.249368515490000053 ) ) ;
#6313=EDGE_CURVE ( 'NONE', #25599, #1700, #4319, .T. ) ;
#6315=CARTESIAN_POINT ( 'NONE',  ( -1.228311966399999955, -101.1461874320000049, -16.11255545180000226 ) ) ;
#6318=CARTESIAN_POINT ( 'NONE',  ( -20.37063303559435212, -92.65976904082468479, -22.69994848242665242 ) ) ;
#6321=CARTESIAN_POINT ( 'NONE',  ( -6.851093861369999871, -101.2010924020000004, 13.63775431790000070 ) ) ;
#6323=B_SPLINE_CURVE_WITH_KNOTS ( 'NONE', 5,
 ( #15457, #12983, #6441, #24665, #20140, #24814, #11381, #10787, #10931, #21893, #15307, #17815, #350, #24224, #27004 ),
 .UNSPECIFIED., .F., .F.,
 ( 6, 3, 3, 3, 6 ),
 ( -72.86859331460000533, -71.60123715040001002, -63.48927009810000044, -56.91038232380000039, -54.97253517989999949 ),
 .UNSPECIFIED. ) ;
#6326=CARTESIAN_POINT ( 'NONE',  ( 24.62113160253329269, -93.59825775071381315, -11.14135564786052335 ) ) ;
#6334=CARTESIAN_POINT ( 'NONE',  ( -25.28414760490000290, -93.59856727289999867, -2.205049167689999923 ) ) ;
#6350=CARTESIAN_POINT ( 'NONE',  ( -13.31136913029999924, -101.0685849509999912, -9.042834681369999572 ) ) ;
#6351=B_SPLINE_SURFACE_WITH_KNOTS ( 'NONE', 5, 5, ( 
 ( #9365, #13887, #20296, #22789, #2829, #11690, #20601, #661, #16208 ),
 ( #25120, #14036, #16362, #3398, #14187, #25272, #25408, #9653, #25540 ),
 ( #7644, #27861, #27453, #8045, #7909, #16792, #25827, #7773, #16511 ),
 ( #27604, #25686, #7499, #5301, #11980, #12265, #5578, #14595, #22941 ),
 ( #5437, #2982, #23083, #5711, #21174, #5848, #14322, #23498, #14462 ),
 ( #3126, #27737, #10204, #20894, #3266, #12120, #1095, #10067, #3537 ) ),
 .UNSPECIFIED., .F., .F., .F.,
 ( 6, 6 ),
 ( 6, 3, 6 ),
 ( 0.000000000000000000, 0.1274251584810000004 ),
 ( 0.000000000000000000, 0.2500000000000000000, 0.5000000000000000000 ),
 .UNSPECIFIED. ) ;
#6354=CARTESIAN_POINT ( 'NONE',  ( -12.21857400070000033, -100.8455998110000138, -10.39687837159999972 ) ) ;
#6356=CARTESIAN_POINT ( 'NONE',  ( -7.823320741682010748, -100.6644468684844327, 14.83362164074870648 ) ) ;
#6363=CARTESIAN_POINT ( 'NONE',  ( 12.80450062669999944, -92.92146214120000991, 27.55316299560000104 ) ) ;
#6366=CARTESIAN_POINT ( 'NONE',  ( -17.50873242076130509, -93.40025063778267622, -21.36494869218120840 ) ) ;
#6368=CARTESIAN_POINT ( 'NONE',  ( 24.26105873420000236, -93.48569624599998917, 12.29345215780000089 ) ) ;
#6370=ORIENTED_EDGE ( 'NONE', *, *, #21230, .F. ) ;
#6376=ORIENTED_EDGE ( 'NONE', *, *, #23951, .T. ) ;
#6378=CARTESIAN_POINT ( 'NONE',  ( -21.84411882930000104, -92.49537389370000540, -19.67291967990000146 ) ) ;
#6379=AXIS2_PLACEMENT_3D ( 'NONE', #3649, #23480, #26074 ) ;
#6380=CARTESIAN_POINT ( 'NONE',  ( -18.01708526109999653, -94.13770192399999814, 18.41653692539999909 ) ) ;
#6383=CARTESIAN_POINT ( 'NONE',  ( 13.07785959079999927, -101.1976625110000043, -9.812318318510000026 ) ) ;
#6392=CARTESIAN_POINT ( 'NONE',  ( 0.2284267155709999997, -92.50000000000000000, -29.91770779450000362 ) ) ;
#6395=AXIS2_PLACEMENT_3D ( 'NONE', #9992, #19321, #5634 ) ;
#6400=CARTESIAN_POINT ( 'NONE',  ( 22.60964169310000216, -96.07623048240000685, -4.342433871829999070 ) ) ;
#6401=ORIENTED_EDGE ( 'NONE', *, *, #2956, .F. ) ;
#6404=EDGE_CURVE ( 'NONE', #8764, #27709, #1533, .T. ) ;
#6405=CARTESIAN_POINT ( 'NONE',  ( 15.77847589470000145, -100.9405348700000076, 2.296806114620000283 ) ) ;
#6406=EDGE_CURVE ( 'NONE', #17438, #18837, #20711, .T. ) ;
#6408=CARTESIAN_POINT ( 'NONE',  ( -7.984177743680001882, -99.69348480060000384, 15.37172668299999856 ) ) ;
#6409=CARTESIAN_POINT ( 'NONE',  ( -6.697057311400000046, -97.13885494210001070, -19.48988624889999954 ) ) ;
#6411=DIRECTION ( 'NONE',  ( 0.000000000000000000, 1.000000000000000000, 0.000000000000000000 ) ) ;
#6412=CARTESIAN_POINT ( 'NONE',  ( -20.43934827010000177, -94.59274571439999590, 12.18706707989999849 ) ) ;
#6414=DIRECTION ( 'NONE',  ( 0.9999792992113794021, 0.000000000000000000, 0.006434372441712415611 ) ) ;
#6417=CARTESIAN_POINT ( 'NONE',  ( 13.61208627270031535, -100.4507315469313653, -10.08440332799037265 ) ) ;
#6419=CARTESIAN_POINT ( 'NONE',  ( 12.04737265770000043, -111.0000000000000000, -10.52904611289999970 ) ) ;
#6420=CARTESIAN_POINT ( 'NONE',  ( -17.00715350810000004, -99.92967601899998442, 3.484608414699999823 ) ) ;
#6421=VERTEX_POINT ( 'NONE', #18582 ) ;
#6424=CARTESIAN_POINT ( 'NONE',  ( -13.18661255610000183, -92.50000050529999385, 26.85581263849999800 ) ) ;
#6429=CARTESIAN_POINT ( 'NONE',  ( 0.4405410860649999760, -101.0405520670000072, -16.24120667380000071 ) ) ;
#6436=CARTESIAN_POINT ( 'NONE',  ( -15.94967535902879696, -92.55895609343200192, -24.01911116337151597 ) ) ;
#6441=CARTESIAN_POINT ( 'NONE',  ( -13.41727642240000051, -92.50059758980000879, 26.58634259119999754 ) ) ;
#6442=CARTESIAN_POINT ( 'NONE',  ( 4.581687752772167777, -92.77481473406787416, -30.15399321906782859 ) ) ;
#6443=CARTESIAN_POINT ( 'NONE',  ( -3.134349734139999732, -94.63960162979999780, 23.52861365520000092 ) ) ;
#6445=CARTESIAN_POINT ( 'NONE',  ( 9.396859518459999450, -94.80026553589999594, -22.54656200069999983 ) ) ;
#6448=VERTEX_POINT ( 'NONE', #3004 ) ;
#6454=ORIENTED_EDGE ( 'NONE', *, *, #3806, .T. ) ;
#6455=CARTESIAN_POINT ( 'NONE',  ( -1.396721017910000029, -100.9938510739999913, -15.46647101679999992 ) ) ;
#6458=AXIS2_PLACEMENT_3D ( 'NONE', #21681, #17310, #26203 ) ;
#6461=CARTESIAN_POINT ( 'NONE',  ( -14.57802700750000113, -101.2141579089999937, 4.464741364610000041 ) ) ;
#6463=CARTESIAN_POINT ( 'NONE',  ( -7.177518981630000461, -101.0875971110000080, 13.63542055629999972 ) ) ;
#6464=CIRCLE ( 'NONE', #23234, 16.00000000000000000 ) ;
#6471=CARTESIAN_POINT ( 'NONE',  ( 26.37317065237687430, -92.86910576385687932, 13.16124730488680683 ) ) ;
#6474=( LENGTH_UNIT ( ) NAMED_UNIT ( * ) SI_UNIT ( .MILLI., .METRE. ) );
#6475=CARTESIAN_POINT ( 'NONE',  ( 20.39090231782646612, -94.79128788299946962, 14.04608546598787910 ) ) ;
#6479=ADVANCED_FACE ( 'NONE', ( #18434 ), #828, .F. ) ;
#6484=CARTESIAN_POINT ( 'NONE',  ( -24.61280144410000048, -93.91547326130000783, -2.656926711870000180 ) ) ;
#6489=CARTESIAN_POINT ( 'NONE',  ( 15.50655985760000100, -100.4792519539999915, 4.667916574389999518 ) ) ;
#6491=CARTESIAN_POINT ( 'NONE',  ( -13.32816333360000094, -99.92967571559999840, -11.12411022969999941 ) ) ;
#6495=EDGE_LOOP ( 'NONE', ( #15601, #16614, #4734, #1298 ) ) ;
#6497=B_SPLINE_CURVE_WITH_KNOTS ( 'NONE', 5,
 ( #3815, #17212, #16941, #8457, #21589, #1647 ),
 .UNSPECIFIED., .F., .F.,
 ( 6, 6 ),
 ( 0.000000000000000000, 1.000000000000000000 ),
 .UNSPECIFIED. ) ;
#6500=CARTESIAN_POINT ( 'NONE',  ( -14.96437297340000150, -101.1411470200000053, 3.591084556139999773 ) ) ;
#6506=CARTESIAN_POINT ( 'NONE',  ( -12.35404653890000048, -101.0640712160000021, -10.32358696690000066 ) ) ;
#6512=EDGE_CURVE ( 'NONE', #8949, #19113, #3958, .T. ) ;
#6514=DIRECTION ( 'NONE',  ( 0.7778035323410003032, 0.000000000000000000, 0.6285074900730003300 ) ) ;
#6517=EDGE_CURVE ( 'NONE', #23865, #3774, #11746, .T. ) ;
#6521=CARTESIAN_POINT ( 'NONE',  ( 12.77500000340000064, -92.50000200359998814, 27.05403400520000190 ) ) ;
#6524=CARTESIAN_POINT ( 'NONE',  ( -14.03104053434696930, -94.16483583410587244, -21.61783809625667274 ) ) ;
#6526=CARTESIAN_POINT ( 'NONE',  ( 19.89027466199999949, -94.80026553589999594, 14.17834266530000065 ) ) ;
#6538=CARTESIAN_POINT ( 'NONE',  ( 12.47562891269999952, -101.2902355740000075, -9.903343504470001335 ) ) ;
#6540=CARTESIAN_POINT ( 'NONE',  ( -11.77049175740000209, -94.59276292389999696, -20.68200892780000189 ) ) ;
#6542=CARTESIAN_POINT ( 'NONE',  ( 29.81958713258436688, -92.61393927540532900, 6.406587609757409041 ) ) ;
#6544=ORIENTED_EDGE ( 'NONE', *, *, #23044, .T. ) ;
#6545=EDGE_CURVE ( 'NONE', #10101, #17438, #9893, .T. ) ;
#6547=CARTESIAN_POINT ( 'NONE',  ( -16.57262063419999976, -111.0000000000000000, 13.26958147880000105 ) ) ;
#6548=CARTESIAN_POINT ( 'NONE',  ( -23.82443726134325956, -92.82709422631620555, -19.04327167594423287 ) ) ;
#6550=CARTESIAN_POINT ( 'NONE',  ( 16.79922297439999923, -99.53431386179998697, 4.586272525910000120 ) ) ;
#6551=AXIS2_PLACEMENT_3D ( 'NONE', #22200, #11251, #2834 ) ;
#6554=ADVANCED_FACE ( 'NONE', ( #19695 ), #25893, .T. ) ;
#6560=CARTESIAN_POINT ( 'NONE',  ( 21.95870570019999946, -95.72998413979999555, -4.498066912960000607 ) ) ;
#6563=FACE_OUTER_BOUND ( 'NONE', #6818, .T. ) ;
#6567=CARTESIAN_POINT ( 'NONE',  ( -11.18835985219999962, -94.77533619469998882, -20.78534805609999836 ) ) ;
#6569=DIRECTION ( 'NONE',  ( -0.000000000000000000, 1.000000000000000000, 0.000000000000000000 ) ) ;
#6572=CARTESIAN_POINT ( 'NONE',  ( 11.60714335010259290, -98.09459568849395339, -16.83342208755517078 ) ) ;
#6582=CARTESIAN_POINT ( 'NONE',  ( -14.94824859369999892, -92.53413156150000418, 24.89531834309999780 ) ) ;
#6583=CARTESIAN_POINT ( 'NONE',  ( -23.24818410940000035, -92.50000000000000000, -18.83197690249999923 ) ) ;
#6587=CARTESIAN_POINT ( 'NONE',  ( 0.7986093652169999890, -100.7776802639999971, -15.78831820859999802 ) ) ;
#6588=DIRECTION ( 'NONE',  ( 0.000000000000000000, -1.000000000000000000, 0.000000000000000000 ) ) ;
#6592=EDGE_CURVE ( 'NONE', #26789, #10004, #7085, .T. ) ;
#6599=CARTESIAN_POINT ( 'NONE',  ( 27.96402436456293117, -92.54687141712491893, 12.17634571817241529 ) ) ;
#6600=CARTESIAN_POINT ( 'NONE',  ( 16.48132342839999964, -111.0000000000000000, 2.988055897779999803 ) ) ;
#6601=CARTESIAN_POINT ( 'NONE',  ( -2.934901053329999954, -94.89196973819998959, 23.49669094599999752 ) ) ;
#6602=CARTESIAN_POINT ( 'NONE',  ( 22.56214152920000160, -93.14733690350000472, 15.53136258500000011 ) ) ;
#6603=B_SPLINE_SURFACE_WITH_KNOTS ( 'NONE', 5, 5, ( 
 ( #16481, #21414, #1472, #21149, #8015, #25512 ),
 ( #25795, #20865, #10313, #16617, #19226, #5550 ),
 ( #25654, #3511, #3371, #3100, #5684, #1204 ),
 ( #925, #16905, #21275, #5824, #14706, #3641 ),
 ( #5269, #25242, #10448, #26355, #8278, #19367 ),
 ( #3781, #19641, #28242, #28531, #19502, #17178 ) ),
 .UNSPECIFIED., .F., .F., .F.,
 ( 6, 6 ),
 ( 6, 6 ),
 ( 53.49743275559999489, 69.76497130679999259 ),
 ( 0.000000000000000000, 0.5000000000000000000 ),
 .UNSPECIFIED. ) ;
#6606=CARTESIAN_POINT ( 'NONE',  ( -6.850910565599999558, -101.0956037589999994, 13.95379404589999872 ) ) ;
#6609=CARTESIAN_POINT ( 'NONE',  ( -13.16293296443088678, -100.0863963178061056, -11.12354968663382238 ) ) ;
#6613=CARTESIAN_POINT ( 'NONE',  ( 7.007938636740000504, -99.64579651319999698, 15.84020959899999959 ) ) ;
#6615=LINE ( 'NONE', #22350, #10236 ) ;
#6617=CARTESIAN_POINT ( 'NONE',  ( -19.43609242099999790, -92.50000000000000000, -23.50506990850000122 ) ) ;
#6620=FACE_OUTER_BOUND ( 'NONE', #13862, .T. ) ;
#6621=CARTESIAN_POINT ( 'NONE',  ( -8.226221597980000411, -100.1275643909999928, 14.47297520289999895 ) ) ;
#6627=CARTESIAN_POINT ( 'NONE',  ( 15.07154978059999983, -101.2141467319999890, 2.302521054160000080 ) ) ;
#6628=CARTESIAN_POINT ( 'NONE',  ( 21.46597110810399656, -94.35876167800067549, 13.63254091422909298 ) ) ;
#6629=ORIENTED_EDGE ( 'NONE', *, *, #18939, .T. ) ;
#6632=EDGE_LOOP ( 'NONE', ( #20254, #25747, #14340, #26601 ) ) ;
#6636=CARTESIAN_POINT ( 'NONE',  ( -23.69409928740000026, -94.52419443349998573, -3.934983043100000355 ) ) ;
#6641=ORIENTED_EDGE ( 'NONE', *, *, #26296, .F. ) ;
#6643=CARTESIAN_POINT ( 'NONE',  ( -13.41619510559999995, -101.2306310700000012, -9.103917256129998137 ) ) ;
#6645=CARTESIAN_POINT ( 'NONE',  ( 7.845180177321567250, -92.53708507728565280, 29.47379534260642586 ) ) ;
#6647=CIRCLE ( 'NONE', #21100, 21.14285714289999873 ) ;
#6650=CARTESIAN_POINT ( 'NONE',  ( 23.75537003280000192, -92.54628605920001405, -18.53955413979999989 ) ) ;
#6653=CARTESIAN_POINT ( 'NONE',  ( -16.65305080357083867, -98.39905935350182631, 8.896395905759751699 ) ) ;
#6657=CARTESIAN_POINT ( 'NONE',  ( -12.79195022560000083, -100.5229262450000078, -11.01668120969999976 ) ) ;
#6659=CARTESIAN_POINT ( 'NONE',  ( 0.000000000000000000, -108.5000000000000000, 0.000000000000000000 ) ) ;
#6661=ORIENTED_EDGE ( 'NONE', *, *, #3456, .T. ) ;
#6668=CARTESIAN_POINT ( 'NONE',  ( 12.80450063680000028, -93.00000194650000651, 27.55316300550000008 ) ) ;
#6669=B_SPLINE_CURVE_WITH_KNOTS ( 'NONE', 5,
 ( #11874, #20786, #25307, #841, #7536, #23111 ),
 .UNSPECIFIED., .F., .F.,
 ( 6, 6 ),
 ( 0.000000000000000000, 1.000000000000000000 ),
 .UNSPECIFIED. ) ;
#6672=CARTESIAN_POINT ( 'NONE',  ( -19.37994895511149451, -96.88257430336904008, 7.664418457435713705 ) ) ;
#6673=ORIENTED_EDGE ( 'NONE', *, *, #7253, .T. ) ;
#6681=EDGE_CURVE ( 'NONE', #7956, #27080, #13121, .T. ) ;
#6683=EDGE_CURVE ( 'NONE', #25457, #3331, #24304, .T. ) ;
#6685=CARTESIAN_POINT ( 'NONE',  ( -16.36167018629999959, -93.01125874779999947, -20.97227418339999971 ) ) ;
#6687=ORIENTED_EDGE ( 'NONE', *, *, #13481, .T. ) ;
#6688=EDGE_CURVE ( 'NONE', #22989, #26789, #4721, .T. ) ;
#6689=CARTESIAN_POINT ( 'NONE',  ( -6.075137112332721578, -101.5902664364218708, 14.84893169810246327 ) ) ;
#6691=CARTESIAN_POINT ( 'NONE',  ( 13.77551190490000188, -100.0482783049999966, -10.29143743870000094 ) ) ;
#6694=AXIS2_PLACEMENT_3D ( 'NONE', #5475, #16975, #1267 ) ;
#6695=CARTESIAN_POINT ( 'NONE',  ( 23.96368475870000125, -111.0000000000000000, 8.717328305520000598 ) ) ;
#6701=CARTESIAN_POINT ( 'NONE',  ( -23.86210134984825615, -92.77521214514680992, -18.99609179358898103 ) ) ;
#6703=CARTESIAN_POINT ( 'NONE',  ( 0.1200718050890000055, -93.00000000000000000, -30.49976365090000030 ) ) ;
#6704=CARTESIAN_POINT ( 'NONE',  ( -14.74973743588710207, -100.9709810896216027, 4.950683569343071966 ) ) ;
#6710=CARTESIAN_POINT ( 'NONE',  ( 23.25684308690000179, -94.57749834670001121, -6.685466565999999666 ) ) ;
#6718=CARTESIAN_POINT ( 'NONE',  ( -4.790709198910000133, -98.40794110039999509, -18.33800208579999946 ) ) ;
#6719=CARTESIAN_POINT ( 'NONE',  ( 7.257715839349999420, -101.2520799100000062, 13.34996420839999942 ) ) ;
#6721=CARTESIAN_POINT ( 'NONE',  ( -17.12546904050000052, -99.53431416519998720, 3.156803742540000179 ) ) ;
#6722=AXIS2_PLACEMENT_3D ( 'NONE', #11858, #27750, #1242 ) ;
#6724=CARTESIAN_POINT ( 'NONE',  ( 9.374849361280000792, -94.98812477599999227, -22.63660904189999812 ) ) ;
#6727=CARTESIAN_POINT ( 'NONE',  ( 12.19843450850000011, -94.07620464490000245, -21.73166345290000123 ) ) ;
#6728=DIRECTION ( 'NONE',  ( 0.000000000000000000, 1.000000000000000000, 0.000000000000000000 ) ) ;
#6730=CARTESIAN_POINT ( 'NONE',  ( -12.88144346130615148, -92.61393927531646852, 27.64634796700016750 ) ) ;
#6734=CARTESIAN_POINT ( 'NONE',  ( -15.94773428150000250, -93.01843633099998954, 23.99750656370000002 ) ) ;
#6735=DIRECTION ( 'NONE',  ( 1.000000000000000000, 0.000000000000000000, 0.000000000000000000 ) ) ;
#6739=CARTESIAN_POINT ( 'NONE',  ( 1.131980963049999955, -100.1275643909999928, -16.60892386949999988 ) ) ;
#6745=CARTESIAN_POINT ( 'NONE',  ( 28.44395825459533711, -92.82334897395243445, 11.00868981448089023 ) ) ;
#6746=CARTESIAN_POINT ( 'NONE',  ( -11.32307664120000013, -111.0000000000000000, 9.421136869679999748 ) ) ;
#6751=CARTESIAN_POINT ( 'NONE',  ( 23.56161414842587121, -92.59735406120951495, -19.36752225149772499 ) ) ;
#6753=DIRECTION ( 'NONE',  ( 1.000000000000000000, 0.000000000000000000, 0.000000000000000000 ) ) ;
#6759=DIRECTION ( 'NONE',  ( 0.000000000000000000, -1.000000000000000000, 0.000000000000000000 ) ) ;
#6763=EDGE_CURVE ( 'NONE', #7139, #9479, #5209, .T. ) ;
#6764=CARTESIAN_POINT ( 'NONE',  ( 9.335817441729998833, -98.58684426249999433, 16.46450815360000064 ) ) ;
#6768=CARTESIAN_POINT ( 'NONE',  ( -19.91159696475570939, -92.54687141712489051, -23.10364386895400912 ) ) ;
#6770=CARTESIAN_POINT ( 'NONE',  ( -15.38634734859999931, -101.2489796309999974, 4.678841008770000975 ) ) ;
#6771=DIRECTION ( 'NONE',  ( -0.9487039977520664857, 0.000000000000000000, 0.3161656601360223195 ) ) ;
#6772=CARTESIAN_POINT ( 'NONE',  ( 15.96495049010557565, -94.81439201244758408, 17.25884178542835556 ) ) ;
#6773=CARTESIAN_POINT ( 'NONE',  ( 13.79877908105553530, -99.99762666413948864, -10.44370536661393878 ) ) ;
#6776=CARTESIAN_POINT ( 'NONE',  ( 24.68551128330313205, -93.11247489649196041, -15.04102508485111578 ) ) ;
#6777=CARTESIAN_POINT ( 'NONE',  ( 27.46738388089225680, -93.08494709829906810, 9.611772595438951683 ) ) ;
#6778=ORIENTED_EDGE ( 'NONE', *, *, #8336, .F. ) ;
#6784=CARTESIAN_POINT ( 'NONE',  ( -24.15516222109999944, -94.98812477599999227, -4.102682939769999315 ) ) ;
#6789=ORIENTED_EDGE ( 'NONE', *, *, #9439, .T. ) ;
#6793=VERTEX_POINT ( 'NONE', #26282 ) ;
#6801=CARTESIAN_POINT ( 'NONE',  ( 24.60702460379999934, -92.65997669530000280, -15.35181526640000094 ) ) ;
#6804=CARTESIAN_POINT ( 'NONE',  ( -16.92961152516845047, -97.87901546888585358, 9.782674744978539394 ) ) ;
#6805=ORIENTED_EDGE ( 'NONE', *, *, #5285, .F. ) ;
#6808=CYLINDRICAL_SURFACE ( 'NONE', #16014, 5.999999999999999112 ) ;
#6810=EDGE_LOOP ( 'NONE', ( #9704, #13954, #23547, #13042, #25183, #21310, #3433, #17543, #12710, #20831, #9332, #21638, #8832, #1262, #8255, #24367, #11266, #16752, #5820, #23904, #12601, #23708, #9906, #25886, #23422, #1399, #10445, #10786 ) ) ;
#6811=EDGE_CURVE ( 'NONE', #22871, #5855, #1850, .T. ) ;
#6813=ORIENTED_EDGE ( 'NONE', *, *, #25839, .T. ) ;
#6817=CARTESIAN_POINT ( 'NONE',  ( 12.02738831950660092, -101.4628082233756174, -10.51158039492587193 ) ) ;
#6818=EDGE_LOOP ( 'NONE', ( #14207, #7029, #20671, #2515, #24117, #6813, #22991 ) ) ;
#6824=CARTESIAN_POINT ( 'NONE',  ( 6.114061450890000415, -93.00000000000000000, -13.40104985119999981 ) ) ;
#6828=ADVANCED_FACE ( 'NONE', ( #17530 ), #26146, .F. ) ;
#6829=CARTESIAN_POINT ( 'NONE',  ( 12.23878306329999788, -101.1716782170000073, -9.887962090940000337 ) ) ;
#6831=DIRECTION ( 'NONE',  ( 1.000000000000000000, 0.000000000000000000, 0.000000000000000000 ) ) ;
#6834=CARTESIAN_POINT ( 'NONE',  ( 13.87966546279999847, -99.77922884479998800, -10.06442417530000100 ) ) ;
#6838=DIRECTION ( 'NONE',  ( 0.4794255386042041156, 0.000000000000000000, 0.8775825618903722036 ) ) ;
#6842=DIRECTION ( 'NONE',  ( 0.4794255386042040601, 0.000000000000000000, 0.8775825618903720926 ) ) ;
#6843=EDGE_CURVE ( 'NONE', #2923, #2579, #22901, .T. ) ;
#6846=CARTESIAN_POINT ( 'NONE',  ( 8.067175576580000396, -93.91547326120000605, -23.40448531159999845 ) ) ;
#6849=CARTESIAN_POINT ( 'NONE',  ( -14.71230273950800616, -101.0166390262131983, 4.876656405776244263 ) ) ;
#6854=VECTOR ( 'NONE', #27377, 1000.000000000000000 ) ;
#6856=CARTESIAN_POINT ( 'NONE',  ( 16.08037956160000093, -101.3150700380000018, 2.354225989130000141 ) ) ;
#6860=ORIENTED_EDGE ( 'NONE', *, *, #13572, .T. ) ;
#6861=CARTESIAN_POINT ( 'NONE',  ( 13.40713319760000033, -96.04856473240000980, 17.39417937919999702 ) ) ;
#6863=CARTESIAN_POINT ( 'NONE',  ( 5.750188325161174951, -93.39299082539562846, -27.04284275823775729 ) ) ;
#6864=CARTESIAN_POINT ( 'NONE',  ( 1.316303147800000017, -94.80026829419999501, 24.39090705379999946 ) ) ;
#6865=PLANE ( 'NONE',  #9921 ) ;
#6867=VERTEX_POINT ( 'NONE', #3840 ) ;
#6871=CARTESIAN_POINT ( 'NONE',  ( -12.43631275050667639, -92.52249206702077799, 27.84938838431781605 ) ) ;
#6878=AXIS2_PLACEMENT_3D ( 'NONE', #17532, #3843, #4120 ) ;
#6879=CARTESIAN_POINT ( 'NONE',  ( -14.79537535560000094, -100.9197064490000031, 5.022278568880000016 ) ) ;
#6880=CARTESIAN_POINT ( 'NONE',  ( 0.6036065640569999724, -99.94751438429999268, -17.14557600869999732 ) ) ;
#6885=ADVANCED_FACE ( 'NONE', ( #19708 ), #17050, .T. ) ;
#6887=DIRECTION ( 'NONE',  ( 1.000000000000000000, 0.000000000000000000, 0.000000000000000000 ) ) ;
#6891=EDGE_CURVE ( 'NONE', #4490, #13918, #10607, .T. ) ;
#6893=ORIENTED_EDGE ( 'NONE', *, *, #2789, .F. ) ;
#6894=CARTESIAN_POINT ( 'NONE',  ( 28.14643818373028239, -92.62800705134026202, 11.74875853647297319 ) ) ;
#6898=CARTESIAN_POINT ( 'NONE',  ( 18.39097457039999739, -93.63284696350000047, 17.05711537220000196 ) ) ;
#6908=CARTESIAN_POINT ( 'NONE',  ( -29.52609378599999701, -92.68584525839999344, -0.4443637791730000175 ) ) ;
#6909=CARTESIAN_POINT ( 'NONE',  ( -3.941341475290000229, -96.93384555679999437, -20.91998619789999836 ) ) ;
#6912=CARTESIAN_POINT ( 'NONE',  ( 11.63640002800000062, -101.0314399550000104, -10.76925615409999892 ) ) ;
#6913=CYLINDRICAL_SURFACE ( 'NONE', #9730, 0.8000000000000002665 ) ;
#6914=CARTESIAN_POINT ( 'NONE',  ( -22.71111200904663363, -95.90275866728285337, -5.472871145369948565 ) ) ;
#6919=CARTESIAN_POINT ( 'NONE',  ( 14.98792925300000078, -101.2530993039999885, 2.502342737139999773 ) ) ;
#6920=CARTESIAN_POINT ( 'NONE',  ( 23.42170070327015807, -93.74885977147994254, 12.68526725471132899 ) ) ;
#6924=AXIS2_PLACEMENT_3D ( 'NONE', #11923, #27097, #27539 ) ;
#6925=CARTESIAN_POINT ( 'NONE',  ( 7.952856579429999684, -100.9640305859999927, 13.43340132319999825 ) ) ;
#6926=EDGE_CURVE ( 'NONE', #1588, #6867, #12179, .T. ) ;
#6927=ORIENTED_EDGE ( 'NONE', *, *, #22923, .T. ) ;
#6934=CARTESIAN_POINT ( 'NONE',  ( 15.95399948070000029, -100.1340845430000002, 4.725790154640000296 ) ) ;
#6936=CIRCLE ( 'NONE', #12033, 0.4999999999999995559 ) ;
#6937=CARTESIAN_POINT ( 'NONE',  ( 11.27094287870000144, -92.51078253369999516, 27.07599673740000057 ) ) ;
#6941=ORIENTED_EDGE ( 'NONE', *, *, #23278, .F. ) ;
#6942=AXIS2_PLACEMENT_3D ( 'NONE', #14700, #5678, #12090 ) ;
#6949=FACE_OUTER_BOUND ( 'NONE', #19108, .T. ) ;
#6951=DIRECTION ( 'NONE',  ( -0.000000000000000000, 1.000000000000000000, 0.000000000000000000 ) ) ;
#6953=CARTESIAN_POINT ( 'NONE',  ( -16.09618210462868504, -99.28123783267172087, 7.460060003079973967 ) ) ;
#6956=CARTESIAN_POINT ( 'NONE',  ( 5.273680924649999824, -107.1975888269999899, 9.653408180790000515 ) ) ;
#6957=CARTESIAN_POINT ( 'NONE',  ( -12.65137342600000103, -100.3517545579999961, -10.97941968159999959 ) ) ;
#6969=CARTESIAN_POINT ( 'NONE',  ( 10.50444872630000148, -92.78939691329999562, 27.51880632769999835 ) ) ;
#6973=CARTESIAN_POINT ( 'NONE',  ( 20.30842400699999928, -94.18458655290000081, 13.41360490589999976 ) ) ;
#6978=EDGE_CURVE ( 'NONE', #25061, #726, #430, .T. ) ;
#6979=DIRECTION ( 'NONE',  ( 0.000000000000000000, -1.000000000000000000, 0.000000000000000000 ) ) ;
#6981=CARTESIAN_POINT ( 'NONE',  ( -24.15516222759999820, -94.98812477599999227, -4.102682929219999330 ) ) ;
#6982=ORIENTED_EDGE ( 'NONE', *, *, #12072, .T. ) ;
#6985=CARTESIAN_POINT ( 'NONE',  ( -6.105475123031572693, -101.6077248516953091, 14.82224783260342882 ) ) ;
#6986=CARTESIAN_POINT ( 'NONE',  ( -16.99294773969999994, -99.88067626670000720, 3.462731254189999941 ) ) ;
#6993=ORIENTED_EDGE ( 'NONE', *, *, #4298, .F. ) ;
#6994=CARTESIAN_POINT ( 'NONE',  ( -8.404838270569999992, -94.10247623609998868, -22.94303993669999997 ) ) ;
#6998=CARTESIAN_POINT ( 'NONE',  ( 15.99276245056722701, -100.9510322832866223, 4.232737490328940311 ) ) ;
#7009=DIRECTION ( 'NONE',  ( 0.000000000000000000, -1.000000000000000000, 0.000000000000000000 ) ) ;
#7010=EDGE_LOOP ( 'NONE', ( #24743, #25985, #20685, #547 ) ) ;
#7011=CARTESIAN_POINT ( 'NONE',  ( 13.51459830149999952, -96.25026288549999265, 17.16122692649999948 ) ) ;
#7012=EDGE_CURVE ( 'NONE', #5746, #21862, #7077, .T. ) ;
#7013=CARTESIAN_POINT ( 'NONE',  ( 6.184287104840868743, -93.48480241466988616, -26.64338075428234376 ) ) ;
#7016=CARTESIAN_POINT ( 'NONE',  ( -18.94125844690000093, -97.58046871240000542, 6.456825720490000364 ) ) ;
#7020=CARTESIAN_POINT ( 'NONE',  ( 8.907716207360000027, -92.51556042380001088, -27.33482343870000264 ) ) ;
#7021=DIRECTION ( 'NONE',  ( 0.4794255386042041156, 0.000000000000000000, 0.8775825618903722036 ) ) ;
#7025=TOROIDAL_SURFACE ( 'NONE', #6551, 5.500000000000000000, 0.5000000000000000000 ) ;
#7026=CYLINDRICAL_SURFACE ( 'NONE', #21583, 20.64285714290000229 ) ;
#7029=ORIENTED_EDGE ( 'NONE', *, *, #10049, .T. ) ;
#7038=PLANE ( 'NONE',  #22388 ) ;
#7041=CARTESIAN_POINT ( 'NONE',  ( 28.20244470975386974, -92.65976904079265353, 11.61346045625293577 ) ) ;
#7042=FACE_OUTER_BOUND ( 'NONE', #13246, .T. ) ;
#7046=CARTESIAN_POINT ( 'NONE',  ( -20.20541094980000096, -94.98812148390000232, 12.40015412250000004 ) ) ;
#7050=CARTESIAN_POINT ( 'NONE',  ( -6.851093861369999871, -101.2010924020000004, 13.63775431790000070 ) ) ;
#7052=CARTESIAN_POINT ( 'NONE',  ( -12.45052468959800507, -101.4085864806826720, -10.34185987599518874 ) ) ;
#7057=ADVANCED_FACE ( 'NONE', ( #23145 ), #10740, .F. ) ;
#7060=CARTESIAN_POINT ( 'NONE',  ( -2.230088632699999796, -97.73638926269998706, -19.83206999720000141 ) ) ;
#7065=CARTESIAN_POINT ( 'NONE',  ( -18.51512085397209972, -98.37417905202403290, -7.778978700159559168 ) ) ;
#7069=CARTESIAN_POINT ( 'NONE',  ( -11.32307664120000013, -93.00000000000000000, 9.421136869679999748 ) ) ;
#7070=CARTESIAN_POINT ( 'NONE',  ( 24.73091569213457674, -93.38554229052955691, -12.41662862040795723 ) ) ;
#7071=CARTESIAN_POINT ( 'NONE',  ( 27.36513940969999936, -93.00000000000000000, 13.03937715500000039 ) ) ;
#7074=AXIS2_PLACEMENT_3D ( 'NONE', #11870, #25304, #9679 ) ;
#7077=B_SPLINE_CURVE_WITH_KNOTS ( 'NONE', 3,
 ( #7710, #24895, #16134, #590, #13807, #23008, #1026, #9866, #11609, #22713 ),
 .UNSPECIFIED., .F., .F.,
 ( 4, 2, 2, 2, 4 ),
 ( 0.000000000000000000, 0.2500000000000000000, 0.5000000000000000000, 0.7500000000000000000, 1.000000000000000000 ),
 .UNSPECIFIED. ) ;
#7078=CARTESIAN_POINT ( 'NONE',  ( 7.816430931350000222, -101.0685486349999991, 13.30758411539999919 ) ) ;
#7079=CARTESIAN_POINT ( 'NONE',  ( 22.51817718370000065, -95.94970068820001075, -0.7108459635960000522 ) ) ;
#7085=LINE ( 'NONE', #15948, #13615 ) ;
#7088=CARTESIAN_POINT ( 'NONE',  ( -23.55554596629999864, -94.54719592040000009, -3.773182298170000060 ) ) ;
#7091=CARTESIAN_POINT ( 'NONE',  ( -30.48995558417433216, -92.50638022835022412, 0.7959123993752857951 ) ) ;
#7095=CARTESIAN_POINT ( 'NONE',  ( -6.858694523154360567, -97.53591929605553901, 18.86159558765225341 ) ) ;
#7096=CARTESIAN_POINT ( 'NONE',  ( -13.14566783280000095, -99.53431386179998697, -11.42099844400000030 ) ) ;
#7101=CARTESIAN_POINT ( 'NONE',  ( -17.03020756475430275, -97.66307011826351925, 10.16080538950990331 ) ) ;
#7102=B_SPLINE_SURFACE_WITH_KNOTS ( 'NONE', 5, 5, ( 
 ( #6242, #12782, #27976, #3509, #17175, #8013 ),
 ( #5822, #12918, #10311, #7876, #8276, #26063 ),
 ( #16757, #6091, #14833, #3779, #12639, #5682 ),
 ( #14562, #21553, #8414, #1608, #23469, #10579 ),
 ( #12366, #16903, #1329, #17321, #14969, #25793 ),
 ( #19500, #15106, #19224, #21690, #10446, #3639 ) ),
 .UNSPECIFIED., .F., .F., .F.,
 ( 6, 6 ),
 ( 6, 6 ),
 ( 15.82768567759999989, 30.79603606510000091 ),
 ( 0.000000000000000000, 0.5000000000000000000 ),
 .UNSPECIFIED. ) ;
#7106=CARTESIAN_POINT ( 'NONE',  ( -13.17630453619999997, -99.61736775859999682, -11.27972924090000006 ) ) ;
#7112=EDGE_LOOP ( 'NONE', ( #26747, #1860, #23308, #24440 ) ) ;
#7116=CARTESIAN_POINT ( 'NONE',  ( 5.602404968130000107, -93.19697538779999491, 26.61643030870000004 ) ) ;
#7118=VERTEX_POINT ( 'NONE', #6166 ) ;
#7125=DIRECTION ( 'NONE',  ( 0.000000000000000000, 1.000000000000000000, 0.000000000000000000 ) ) ;
#7127=CARTESIAN_POINT ( 'NONE',  ( 0.000000000000000000, -91.50000000000000000, 0.000000000000000000 ) ) ;
#7131=CARTESIAN_POINT ( 'NONE',  ( -16.87609683389999660, -99.97540119910000556, 3.286633550649999957 ) ) ;
#7135=CARTESIAN_POINT ( 'NONE',  ( -12.29363612059999866, -101.2530993000000024, -8.928690578620001261 ) ) ;
#7136=DIRECTION ( 'NONE',  ( 1.000000000000000000, 0.000000000000000000, 0.000000000000000000 ) ) ;
#7137=CARTESIAN_POINT ( 'NONE',  ( 0.1178905558060000108, -101.2358105800000061, -15.21680457949999976 ) ) ;
#7139=VERTEX_POINT ( 'NONE', #5152 ) ;
#7142=CARTESIAN_POINT ( 'NONE',  ( 23.58655530659999755, -94.70873790539999959, -2.249368515490000053 ) ) ;
#7144=CARTESIAN_POINT ( 'NONE',  ( 15.62649610739214090, -101.5829753080984972, 3.664801835284849485 ) ) ;
#7152=CARTESIAN_POINT ( 'NONE',  ( 8.576875435287405480, -93.15740241113648779, 27.32333530169154301 ) ) ;
#7153=ORIENTED_EDGE ( 'NONE', *, *, #10145, .F. ) ;
#7155=ORIENTED_EDGE ( 'NONE', *, *, #6545, .T. ) ;
#7158=ORIENTED_EDGE ( 'NONE', *, *, #2789, .T. ) ;
#7163=CARTESIAN_POINT ( 'NONE',  ( 1.472192074426218689, -93.00000237470425191, -29.94733696998120820 ) ) ;
#7165=CARTESIAN_POINT ( 'NONE',  ( -19.50386435929999962, -96.83699978299999600, 8.450360047540000252 ) ) ;
#7171=CARTESIAN_POINT ( 'NONE',  ( -13.34145344800987942, -92.96960399592896351, 27.42727875496046508 ) ) ;
#7178=ORIENTED_EDGE ( 'NONE', *, *, #20752, .T. ) ;
#7179=CARTESIAN_POINT ( 'NONE',  ( -18.26050467580000003, -97.41004717059999507, 11.26842931770000078 ) ) ;
#7190=CARTESIAN_POINT ( 'NONE',  ( 12.40657046930000007, -98.24905629650000094, 14.77807252610000077 ) ) ;
#7197=CARTESIAN_POINT ( 'NONE',  ( 0.3872056760440000245, -99.92967571559999840, -17.35614698070000017 ) ) ;
#7201=CARTESIAN_POINT ( 'NONE',  ( 8.377755539869999879, -98.98742664769999067, 16.24331995230000203 ) ) ;
#7205=CARTESIAN_POINT ( 'NONE',  ( -14.85886005390000086, -100.9728335899999934, 4.751291413199999702 ) ) ;
#7207=CARTESIAN_POINT ( 'NONE',  ( 12.69276409558878882, -96.42123289902950489, 17.27298930703739543 ) ) ;
#7211=CARTESIAN_POINT ( 'NONE',  ( 24.63826343349942505, -93.08384138313128631, -15.50111966657502371 ) ) ;
#7212=DIRECTION ( 'NONE',  ( 0.4794255386042036715, 0.000000000000000000, 0.8775825618903723147 ) ) ;
#7214=CARTESIAN_POINT ( 'NONE',  ( 0.000000000000000000, -101.6484611540000031, 0.000000000000000000 ) ) ;
#7216=CARTESIAN_POINT ( 'NONE',  ( -20.20541094980000096, -94.98812148390000232, 12.40015412250000004 ) ) ;
#7218=CARTESIAN_POINT ( 'NONE',  ( 7.685241111800000802, -101.1376244509999935, 13.75999003799999976 ) ) ;
#7219=ADVANCED_FACE ( 'NONE', ( #20448 ), #6351, .T. ) ;
#7223=AXIS2_PLACEMENT_3D ( 'NONE', #5726, #1372, #23514 ) ;
#7224=EDGE_CURVE ( 'NONE', #12473, #21862, #959, .T. ) ;
#7228=CARTESIAN_POINT ( 'NONE',  ( -14.62558108616616614, -93.99439547214892343, -21.62054592744825854 ) ) ;
#7229=CARTESIAN_POINT ( 'NONE',  ( 16.81253980019999972, -99.88067631459999518, 4.253150432089999988 ) ) ;
#7232=CARTESIAN_POINT ( 'NONE',  ( -24.00582602940000143, -94.71481430550001335, -4.132763454370000034 ) ) ;
#7234=CARTESIAN_POINT ( 'NONE',  ( 8.504167659047778827, -92.65976904079447252, 29.29043331537584649 ) ) ;
#7236=CARTESIAN_POINT ( 'NONE',  ( 0.000000000000000000, -102.5000000000000000, 0.000000000000000000 ) ) ;
#7243=CARTESIAN_POINT ( 'NONE',  ( -17.03345617734097317, -97.65592479666719328, 10.17337226560459307 ) ) ;
#7247=CARTESIAN_POINT ( 'NONE',  ( -13.13284500319999992, -100.0994409990000094, -11.14317245900000053 ) ) ;
#7251=CARTESIAN_POINT ( 'NONE',  ( 27.19598314615092249, -92.50000000000001421, -13.80718576071233450 ) ) ;
#7253=EDGE_CURVE ( 'NONE', #10170, #28264, #18554, .T. ) ;
#7256=FACE_OUTER_BOUND ( 'NONE', #3102, .T. ) ;
#7258=CARTESIAN_POINT ( 'NONE',  ( -5.029458127119999844, -99.62155223700000306, 16.98269931899999818 ) ) ;
#7259=CARTESIAN_POINT ( 'NONE',  ( 4.039384380619999604, -93.70847541930001512, 26.05804507789999747 ) ) ;
#7262=CARTESIAN_POINT ( 'NONE',  ( -25.64971708790767835, -94.16483583517798195, -2.508592371179793279 ) ) ;
#7263=CARTESIAN_POINT ( 'NONE',  ( -21.97687417839999569, -92.51331408429999215, -19.45668579410000376 ) ) ;
#7267=PLANE ( 'NONE',  #22499 ) ;
#7268=CARTESIAN_POINT ( 'NONE',  ( -6.754619094799999779, -97.17811284689999241, -19.41490638410000003 ) ) ;
#7278=FACE_OUTER_BOUND ( 'NONE', #22734, .T. ) ;
#7281=FACE_OUTER_BOUND ( 'NONE', #9210, .T. ) ;
#7284=DIRECTION ( 'NONE',  ( -0.5012776526529407750, 0.000000000000000000, -0.8652864929898985702 ) ) ;
#7293=CARTESIAN_POINT ( 'NONE',  ( 12.80450217360000131, -93.00000000000000000, 27.55316291459999789 ) ) ;
#7296=LINE ( 'NONE', #12219, #20544 ) ;
#7297=CARTESIAN_POINT ( 'NONE',  ( 23.05498405910000059, -94.52419709919999491, -6.735184622040000235 ) ) ;
#7299=CARTESIAN_POINT ( 'NONE',  ( 26.02259374959999860, -93.00000000000000000, -15.90831903569999994 ) ) ;
#7300=CARTESIAN_POINT ( 'NONE',  ( -14.79537251110000007, -100.9197086940000077, 5.022279785309999411 ) ) ;
#7306=CARTESIAN_POINT ( 'NONE',  ( 23.05498378868082909, -94.52419745020957009, -6.735183927839049289 ) ) ;
#7312=CARTESIAN_POINT ( 'NONE',  ( 14.89070032189999893, -101.0875971110000080, 3.963397078339999879 ) ) ;
#7318=CARTESIAN_POINT ( 'NONE',  ( -18.21762735589999949, -97.23113437169998008, 11.17752812540000029 ) ) ;
#7319=B_SPLINE_CURVE_WITH_KNOTS ( 'NONE', 5,
 ( #602, #154, #18052, #20380, #9594, #13820, #20532, #308, #16146, #7137, #25051, #16004 ),
 .UNSPECIFIED., .F., .F.,
 ( 6, 3, 3, 6 ),
 ( 0.000000000000000000, 0.4964111757615225495, 0.7833083924343531290, 1.000000000000000000 ),
 .UNSPECIFIED. ) ;
#7320=CARTESIAN_POINT ( 'NONE',  ( 0.8950076880280000147, -99.72202992580000114, -17.14962640039999897 ) ) ;
#7322=EDGE_CURVE ( 'NONE', #17051, #16242, #18107, .T. ) ;
#7324=EDGE_CURVE ( 'NONE', #7420, #17308, #22281, .T. ) ;
#7330=VERTEX_POINT ( 'NONE', #23912 ) ;
#7334=CARTESIAN_POINT ( 'NONE',  ( 23.31078553111326457, -92.52640451556820267, -19.66869558794967432 ) ) ;
#7338=CARTESIAN_POINT ( 'NONE',  ( -8.157403593650000673, -100.1340845430000002, 14.50241216579999914 ) ) ;
#7339=CARTESIAN_POINT ( 'NONE',  ( 6.136951313910000039, -92.68584525849999523, 28.88469321279999846 ) ) ;
#7340=CARTESIAN_POINT ( 'NONE',  ( -11.42926189381041091, -93.65092297039508651, -23.40447979846856796 ) ) ;
#7344=AXIS2_PLACEMENT_3D ( 'NONE', #27896, #5334, #2864 ) ;
#7349=CARTESIAN_POINT ( 'NONE',  ( -3.633275807539999569, -96.53848370299999715, -21.05217880330000213 ) ) ;
#7352=CARTESIAN_POINT ( 'NONE',  ( 11.85649048139999984, -101.3399913430000083, -10.94058650880000094 ) ) ;
#7354=CARTESIAN_POINT ( 'NONE',  ( 15.50203935347336248, -95.03667172802255436, 17.29208320189042425 ) ) ;
#7359=CARTESIAN_POINT ( 'NONE',  ( 13.86995119186533110, -98.07255187705551691, 15.06288721130092512 ) ) ;
#7362=ADVANCED_FACE ( 'NONE', ( #5983 ), #1642, .T. ) ;
#7363=CARTESIAN_POINT ( 'NONE',  ( 6.879827010689999689, -101.5964542560000012, 14.49003032519999934 ) ) ;
#7364=CARTESIAN_POINT ( 'NONE',  ( -17.91778080311958377, -92.49838891740266433, -23.83053502024295156 ) ) ;
#7366=CARTESIAN_POINT ( 'NONE',  ( 22.54736958690000037, -95.60035679240000661, -0.4727289621530000319 ) ) ;
#7375=CARTESIAN_POINT ( 'NONE',  ( -13.32816333360000094, -101.1889999979999999, -11.12411022969999941 ) ) ;
#7379=CARTESIAN_POINT ( 'NONE',  ( -30.45126014524323566, -92.64884742710843568, 1.723988062537378241 ) ) ;
#7381=CARTESIAN_POINT ( 'NONE',  ( 0.5734641406102992667, -100.3041487037959882, -17.04849403054064183 ) ) ;
#7382=EDGE_CURVE ( 'NONE', #23896, #2628, #23081, .T. ) ;
#7383=CARTESIAN_POINT ( 'NONE',  ( -11.98370860700000051, -101.2530993010000060, -9.340542411159999503 ) ) ;
#7385=B_SPLINE_CURVE_WITH_KNOTS ( 'NONE', 5,
 ( #26940, #13514, #2470, #22574, #11323, #440, #4792, #299, #6981 ),
 .UNSPECIFIED., .F., .F.,
 ( 6, 3, 6 ),
 ( 0.000000000000000000, 0.5000000000000000000, 1.000000000000000000 ),
 .UNSPECIFIED. ) ;
#7390=CARTESIAN_POINT ( 'NONE',  ( 13.03263440049999922, -94.63960162979999780, -19.83860502579999974 ) ) ;
#7399=ORIENTED_EDGE ( 'NONE', *, *, #3414, .F. ) ;
#7400=ORIENTED_EDGE ( 'NONE', *, *, #4334, .T. ) ;
#7403=CARTESIAN_POINT ( 'NONE',  ( -4.778856212590000041, -99.55619081999999764, 16.81624398279999966 ) ) ;
#7404=CARTESIAN_POINT ( 'NONE',  ( 10.50533355230000154, -92.65222886450000317, 27.42001380359999985 ) ) ;
#7405=ORIENTED_EDGE ( 'NONE', *, *, #9898, .T. ) ;
#7407=AXIS2_PLACEMENT_3D ( 'NONE', #5225, #7416, #16435 ) ;
#7409=CARTESIAN_POINT ( 'NONE',  ( -28.92399207428294972, -93.08384138316088752, 3.275884373694147200 ) ) ;
#7415=CARTESIAN_POINT ( 'NONE',  ( -4.724916302899999643, -98.37119197950001137, -18.40548062020000231 ) ) ;
#7416=DIRECTION ( 'NONE',  ( -0.6147555381618261539, 7.777821624297800830E-17, 0.7887177114147772006 ) ) ;
#7420=VERTEX_POINT ( 'NONE', #20563 ) ;
#7423=CARTESIAN_POINT ( 'NONE',  ( -16.57647362440000194, -100.3252744939999985, 3.114049206399999825 ) ) ;
#7434=AXIS2_PLACEMENT_3D ( 'NONE', #20860, #2797, #13552 ) ;
#7436=CARTESIAN_POINT ( 'NONE',  ( -9.503513001449999109, -93.67083441959999845, -23.28128293860000042 ) ) ;
#7438=CIRCLE ( 'NONE', #12506, 23.79684788999999867 ) ;
#7443=VERTEX_POINT ( 'NONE', #9905 ) ;
#7452=CARTESIAN_POINT ( 'NONE',  ( 3.624928909112701714, -94.04663295064030137, 25.74405677523981950 ) ) ;
#7457=CARTESIAN_POINT ( 'NONE',  ( -5.845306076740000023, -101.1045726949999874, 14.39333474509999888 ) ) ;
#7460=CARTESIAN_POINT ( 'NONE',  ( 0.000000000000000000, -101.2530993010000060, 0.000000000000000000 ) ) ;
#7461=CIRCLE ( 'NONE', #18618, 23.79684788999999867 ) ;
#7471=CARTESIAN_POINT ( 'NONE',  ( 18.32884736220000121, -98.65110728940000229, 3.454506764930000084 ) ) ;
#7479=CARTESIAN_POINT ( 'NONE',  ( -18.45777030029999821, -95.98445299990001445, 13.67729003380000030 ) ) ;
#7480=CARTESIAN_POINT ( 'NONE',  ( 0.4578259502959999838, -99.78393592979999482, -17.31657152750000250 ) ) ;
#7481=CARTESIAN_POINT ( 'NONE',  ( -16.54318588419999969, -91.50000000000000000, 25.62368046950000178 ) ) ;
#7484=AXIS2_PLACEMENT_3D ( 'NONE', #16, #15417, #22444 ) ;
#7490=CARTESIAN_POINT ( 'NONE',  ( 8.188639545130001807, -100.9197082849999987, 13.30686044670000001 ) ) ;
#7495=CARTESIAN_POINT ( 'NONE',  ( -8.092637767860001219, -100.1512121650000040, 14.53899152610000201 ) ) ;
#7499=CARTESIAN_POINT ( 'NONE',  ( 7.585614467160000096, -101.4252535300000062, 14.05241625360000057 ) ) ;
#7500=VERTEX_POINT ( 'NONE', #27708 ) ;
#7507=EDGE_LOOP ( 'NONE', ( #14256, #18616, #5360, #13627 ) ) ;
#7508=CARTESIAN_POINT ( 'NONE',  ( -11.31667057079999950, -95.23931402160000914, -21.36056405359999744 ) ) ;
#7509=CARTESIAN_POINT ( 'NONE',  ( 12.04737265750000041, -101.6484611540000031, -10.52904611299999971 ) ) ;
#7511=CARTESIAN_POINT ( 'NONE',  ( -17.48265869433503639, -92.69183043860316218, 24.99229797076763049 ) ) ;
#7514=B_SPLINE_CURVE_WITH_KNOTS ( 'NONE', 5,
 ( #12061, #18792, #23158, #20690, #16147, #5237, #21118, #16296, #18928, #11777, #13970, #7848 ),
 .UNSPECIFIED., .F., .F.,
 ( 6, 3, 3, 6 ),
 ( -25.08217527269999891, -18.82032368775269759, -10.56887946808384804, -7.186327137960567768 ),
 .UNSPECIFIED. ) ;
#7515=CARTESIAN_POINT ( 'NONE',  ( 11.93197532131579486, -101.6077248516953233, -10.70531747399618006 ) ) ;
#7519=ORIENTED_EDGE ( 'NONE', *, *, #3500, .T. ) ;
#7520=CARTESIAN_POINT ( 'NONE',  ( 6.669404441700000241, -101.1848541609999899, 13.75051561090000085 ) ) ;
#7521=CARTESIAN_POINT ( 'NONE',  ( -7.333297298759998917, -94.59276292389999696, -22.63874378639999563 ) ) ;
#7522=B_SPLINE_CURVE_WITH_KNOTS ( 'NONE', 5,
 ( #22304, #2350, #182, #18227, #8728, #2650, #9031, #11501, #20409, #24198, #27124, #13105 ),
 .UNSPECIFIED., .F., .F.,
 ( 6, 3, 3, 6 ),
 ( -25.08217526769999850, -18.82032368487667640, -10.56887946683943547, -7.186327137019109301 ),
 .UNSPECIFIED. ) ;
#7523=CARTESIAN_POINT ( 'NONE',  ( 7.743429286519999621, -101.6328744999999998, 14.01526831580000021 ) ) ;
#7525=CIRCLE ( 'NONE', #9821, 11.00000000000000000 ) ;
#7532=CARTESIAN_POINT ( 'NONE',  ( -19.33030770744392868, -93.18010901131746948, -20.96669272993039357 ) ) ;
#7533=LINE ( 'NONE', #20922, #9358 ) ;
#7536=CARTESIAN_POINT ( 'NONE',  ( -19.58183770029999948, -93.00000000000000000, 20.70264511730000123 ) ) ;
#7538=CARTESIAN_POINT ( 'NONE',  ( 9.718892398710000435, -93.00000000000000000, 28.91008700340000104 ) ) ;
#7540=EDGE_CURVE ( 'NONE', #23975, #4037, #16762, .T. ) ;
#7542=CARTESIAN_POINT ( 'NONE',  ( 0.5662235371520514260, -100.9570234915770897, -16.52900152527487876 ) ) ;
#7543=CARTESIAN_POINT ( 'NONE',  ( 6.496108347790000792, -101.2358105800000061, 13.76101799030000095 ) ) ;
#7550=CARTESIAN_POINT ( 'NONE',  ( 12.83908660400000024, -94.89196973819998959, -19.89638119809999850 ) ) ;
#7562=AXIS2_PLACEMENT_3D ( 'NONE', #491, #4975, #15600 ) ;
#7563=CARTESIAN_POINT ( 'NONE',  ( 8.025111386280000758, -92.67508346670000208, 27.00340670960000011 ) ) ;
#7578=CARTESIAN_POINT ( 'NONE',  ( -15.75068343869999765, -101.2375447300000104, 3.306461786589999896 ) ) ;
#7590=CARTESIAN_POINT ( 'NONE',  ( 16.39558919584665730, -100.4211561361363181, 4.355600236979787709 ) ) ;
#7593=B_SPLINE_SURFACE_WITH_KNOTS ( 'NONE', 5, 5, ( 
 ( #27018, #15923, #2547, #13892, #11694, #17832 ),
 ( #9370, #24527, #2244, #26728, #9518, #13296 ),
 ( #2395, #15772, #7060, #16069, #20606, #17977 ),
 ( #6909, #24683, #11398, #523, #18419, #7349 ),
 ( #15628, #24385, #22351, #24828, #18272, #26869 ),
 ( #11087, #4564, #20301, #13442, #4425, #2689 ) ),
 .UNSPECIFIED., .F., .F., .F.,
 ( 6, 6 ),
 ( 6, 6 ),
 ( 15.82768567739999988, 30.79603606530000093 ),
 ( 0.000000000000000000, 0.5000000000000000000 ),
 .UNSPECIFIED. ) ;
#7595=CARTESIAN_POINT ( 'NONE',  ( 6.552802695180705683, -93.39297675734871973, 26.85969955741595783 ) ) ;
#7597=VERTEX_POINT ( 'NONE', #21981 ) ;
#7598=DIRECTION ( 'NONE',  ( 0.000000000000000000, 1.000000000000000000, 0.000000000000000000 ) ) ;
#7601=TOROIDAL_SURFACE ( 'NONE', #20630, 29.91857981989999971, 10.00000000000000000 ) ;
#7603=CARTESIAN_POINT ( 'NONE',  ( -5.873419970429999637, -101.3150705500000157, 15.15334666360000071 ) ) ;
#7610=CARTESIAN_POINT ( 'NONE',  ( -20.22328559685182370, -94.79580598126329960, 12.30740073859241157 ) ) ;
#7611=CARTESIAN_POINT ( 'NONE',  ( -13.09202710664791880, -101.6077248516953091, -9.250658545580620284 ) ) ;
#7612=CARTESIAN_POINT ( 'NONE',  ( 7.610177731959999470, -101.4231532209999926, 14.04048934709999941 ) ) ;
#7615=CARTESIAN_POINT ( 'NONE',  ( 12.88056670439999962, -94.79581646409999962, -19.86310537439999990 ) ) ;
#7618=FACE_OUTER_BOUND ( 'NONE', #12692, .T. ) ;
#7625=VECTOR ( 'NONE', #7834, 1000.000000000000000 ) ;
#7636=VERTEX_POINT ( 'NONE', #2314 ) ;
#7639=EDGE_CURVE ( 'NONE', #23549, #2616, #10117, .T. ) ;
#7640=CARTESIAN_POINT ( 'NONE',  ( -18.05095942279999832, -92.84292204339999444, -23.30076308079999592 ) ) ;
#7644=CARTESIAN_POINT ( 'NONE',  ( 7.614853083119999866, -101.6475450410000008, 14.07253421090000067 ) ) ;
#7645=ORIENTED_EDGE ( 'NONE', *, *, #22086, .T. ) ;
#7647=DIRECTION ( 'NONE',  ( 1.000000000000000000, 0.000000000000000000, 0.000000000000000000 ) ) ;
#7649=CARTESIAN_POINT ( 'NONE',  ( 11.89990227600000061, -99.62155223610000121, -13.11868328289999930 ) ) ;
#7652=CARTESIAN_POINT ( 'NONE',  ( 11.39953095620000134, -101.1130130960000031, -10.39219190439999885 ) ) ;
#7657=CIRCLE ( 'NONE', #20184, 11.00000000000000000 ) ;
#7665=EDGE_CURVE ( 'NONE', #1616, #22947, #12419, .T. ) ;
#7666=CARTESIAN_POINT ( 'NONE',  ( 7.473372113619999979, -101.1715639399999986, 13.35082447569999964 ) ) ;
#7669=CARTESIAN_POINT ( 'NONE',  ( -11.27251375949999890, -95.14587498419999179, -21.35311122079999890 ) ) ;
#7675=ADVANCED_FACE ( 'NONE', ( #13364 ), #24543, .F. ) ;
#7676=ORIENTED_EDGE ( 'NONE', *, *, #25458, .T. ) ;
#7683=CARTESIAN_POINT ( 'NONE',  ( 7.772412540220105193, -93.00000166546708158, -27.92889321292422977 ) ) ;
#7684=CARTESIAN_POINT ( 'NONE',  ( 6.186462384450000407, -100.1275643909999928, 15.45527146859999945 ) ) ;
#7695=SURFACE_SIDE_STYLE ('',( #18757 ) ) ;
#7697=AXIS2_PLACEMENT_3D ( 'NONE', #3128, #9938, #14597 ) ;
#7701=CARTESIAN_POINT ( 'NONE',  ( -28.93075099380000026, -92.79907188619999658, 3.128477965899999713 ) ) ;
#7702=CARTESIAN_POINT ( 'NONE',  ( 9.374849361280000792, -94.98812477599999227, -22.63660904189999812 ) ) ;
#7705=ORIENTED_EDGE ( 'NONE', *, *, #16495, .T. ) ;
#7706=CARTESIAN_POINT ( 'NONE',  ( -28.54678744650632893, -93.15741110514920820, 2.281750724203968073 ) ) ;
#7710=CARTESIAN_POINT ( 'NONE',  ( 7.202169761539999548, -101.2530994060000040, 13.37848089600000101 ) ) ;
#7713=CARTESIAN_POINT ( 'NONE',  ( -13.83118819819999956, -101.1889999979999999, 21.42307711379999802 ) ) ;
#7715=DIRECTION ( 'NONE',  ( -0.9249989688977252600, 0.000000000000000000, -0.3799696139668871098 ) ) ;
#7716=CARTESIAN_POINT ( 'NONE',  ( -15.77992973249999942, -100.6801306890000092, 2.860126966069999721 ) ) ;
#7718=CARTESIAN_POINT ( 'NONE',  ( -6.033294948010268222, -101.1604341566371090, 14.12216738089541401 ) ) ;
#7719=EDGE_CURVE ( 'NONE', #27440, #17051, #9288, .T. ) ;
#7723=CARTESIAN_POINT ( 'NONE',  ( -7.913737673819251306, -100.3041487039959350, 15.11134560035235630 ) ) ;
#7724=ORIENTED_EDGE ( 'NONE', *, *, #24293, .F. ) ;
#7731=UNCERTAINTY_MEASURE_WITH_UNIT (LENGTH_MEASURE( 1.000000000000000082E-05 ), #6474, 'distance_accuracy_value', 'NONE');
#7734=ORIENTED_EDGE ( 'NONE', *, *, #27637, .T. ) ;
#7739=CARTESIAN_POINT ( 'NONE',  ( -5.893649827409999986, -101.1042759770000004, 14.64611091109999919 ) ) ;
#7740=VERTEX_POINT ( 'NONE', #9215 ) ;
#7741=CARTESIAN_POINT ( 'NONE',  ( -18.06041830838391249, -92.73900887645281443, -23.35381297765049169 ) ) ;
#7745=CARTESIAN_POINT ( 'NONE',  ( 23.25684281378446983, -94.57749869811812005, -6.685465864614543285 ) ) ;
#7748=ORIENTED_EDGE ( 'NONE', *, *, #1851, .F. ) ;
#7753=VERTEX_POINT ( 'NONE', #19923 ) ;
#7760=CARTESIAN_POINT ( 'NONE',  ( -15.50938341620000216, -101.3150683030000039, 4.855931779240000523 ) ) ;
#7767=CARTESIAN_POINT ( 'NONE',  ( 0.000000000000000000, -101.1889999979999999, 0.000000000000000000 ) ) ;
#7770=CARTESIAN_POINT ( 'NONE',  ( -13.36314309979999848, -101.1461874320000049, -9.085681040479999027 ) ) ;
#7773=CARTESIAN_POINT ( 'NONE',  ( 7.288000680640000617, -101.1840739500000126, 13.43345668080000088 ) ) ;
#7776=CARTESIAN_POINT ( 'NONE',  ( -27.23152091140000053, -92.68419354089999729, -4.429291780269999812 ) ) ;
#7777=CARTESIAN_POINT ( 'NONE',  ( 10.70182951049999964, -96.07623048470000526, -20.38439291359999928 ) ) ;
#7779=CARTESIAN_POINT ( 'NONE',  ( 0.000000000000000000, -90.50000000000000000, 0.000000000000000000 ) ) ;
#7780=EDGE_CURVE ( 'NONE', #9549, #5628, #7385, .T. ) ;
#7786=CARTESIAN_POINT ( 'NONE',  ( -14.42556421679999978, -93.00000000000000000, -2.978755036369999942 ) ) ;
#7788=ADVANCED_FACE ( 'NONE', ( #27085 ), #19421, .F. ) ;
#7793=CARTESIAN_POINT ( 'NONE',  ( 7.088263367210000609, -101.4254868729999970, 14.30958083260000002 ) ) ;
#7794=DIRECTION ( 'NONE',  ( 0.000000000000000000, 1.000000000000000000, 0.000000000000000000 ) ) ;
#7795=CARTESIAN_POINT ( 'NONE',  ( -11.42656773010000038, -94.70364946070000656, -21.14532863000000162 ) ) ;
#7802=EDGE_LOOP ( 'NONE', ( #24667, #13799, #19675, #28616 ) ) ;
#7805=ORIENTED_EDGE ( 'NONE', *, *, #9736, .F. ) ;
#7807=CARTESIAN_POINT ( 'NONE',  ( 0.5792533394982878336, -100.3266728692868384, -17.03019214104271484 ) ) ;
#7810=CARTESIAN_POINT ( 'NONE',  ( -12.49680195650000059, -94.36515553520000310, -21.45929620349999567 ) ) ;
#7815=CARTESIAN_POINT ( 'NONE',  ( 14.36321081490000040, -97.53592492880000009, -14.01782339449999881 ) ) ;
#7816=B_SPLINE_SURFACE_WITH_KNOTS ( 'NONE', 5, 5, ( 
 ( #14319, #24964, #7339, #9933, #27156, #4995 ),
 ( #13883, #27859, #14994, #8043, #19527, #12391 ),
 ( #17061, #19389, #16788, #10340, #4082, #1354 ),
 ( #23627, #25955, #16931, #8448, #17350, #14592 ),
 ( #3667, #28142, #21863, #23908, #26244, #10065 ),
 ( #21719, #14861, #1500, #12809, #21302, #23765 ) ),
 .UNSPECIFIED., .F., .F., .F.,
 ( 6, 6 ),
 ( 6, 6 ),
 ( 7.179431121690000417, 23.44689954090000228 ),
 ( 0.000000000000000000, 0.5000000000000000000 ),
 .UNSPECIFIED. ) ;
#7818=CARTESIAN_POINT ( 'NONE',  ( -14.83395525719950570, -101.1411475039999317, 4.096596759523888132 ) ) ;
#7820=FACE_OUTER_BOUND ( 'NONE', #28238, .T. ) ;
#7823=EDGE_CURVE ( 'NONE', #20072, #16053, #2906, .T. ) ;
#7829=CARTESIAN_POINT ( 'NONE',  ( -28.60727976599999778, -92.54807930229999613, 3.225833196760000021 ) ) ;
#7834=DIRECTION ( 'NONE',  ( 0.000000000000000000, 1.000000000000000000, 0.000000000000000000 ) ) ;
#7836=CIRCLE ( 'NONE', #20891, 5.000000000000000888 ) ;
#7840=CARTESIAN_POINT ( 'NONE',  ( -22.29269500190000386, -94.98812477769999418, -8.065858985560000249 ) ) ;
#7842=CARTESIAN_POINT ( 'NONE',  ( -15.98611562060000146, -101.1238234200000079, 3.186158858430000240 ) ) ;
#7845=CARTESIAN_POINT ( 'NONE',  ( 14.28941763439999946, -111.0000000000000000, -3.575252188409999921 ) ) ;
#7846=ADVANCED_FACE ( 'NONE', ( #20677 ), #740, .T. ) ;
#7848=CARTESIAN_POINT ( 'NONE',  ( 23.53302756460000111, -92.50000000000000000, -18.47479450719999861 ) ) ;
#7850=B_SPLINE_CURVE_WITH_KNOTS ( 'NONE', 5,
 ( #6136, #24210, #8741, #3821, #19542, #19684 ),
 .UNSPECIFIED., .F., .F.,
 ( 6, 6 ),
 ( 0.000000000000000000, 1.000000000000000000 ),
 .UNSPECIFIED. ) ;
#7855=ORIENTED_EDGE ( 'NONE', *, *, #20104, .F. ) ;
#7857=CYLINDRICAL_SURFACE ( 'NONE', #23769, 30.50000000000002132 ) ;
#7865=CARTESIAN_POINT ( 'NONE',  ( -5.935386223770000136, -101.3399913430000083, 15.00146626390000115 ) ) ;
#7869=CIRCLE ( 'NONE', #20925, 23.79684788999999867 ) ;
#7872=CARTESIAN_POINT ( 'NONE',  ( 22.03755794377824273, -95.57586223393636260, -4.946538409496142208 ) ) ;
#7876=CARTESIAN_POINT ( 'NONE',  ( -15.01486654579999858, -98.65110728940000229, -11.06499187650000060 ) ) ;
#7881=CARTESIAN_POINT ( 'NONE',  ( 15.16019776770000149, -100.8023006570000035, 4.366346884840000442 ) ) ;
#7886=ORIENTED_EDGE ( 'NONE', *, *, #8998, .F. ) ;
#7887=CARTESIAN_POINT ( 'NONE',  ( -17.80822692750000158, -93.00000000000000000, -18.25149456069999943 ) ) ;
#7891=CARTESIAN_POINT ( 'NONE',  ( 0.000000000000000000, -92.50000000000000000, 0.000000000000000000 ) ) ;
#7892=DIRECTION ( 'NONE',  ( 0.4794255386042040601, 0.000000000000000000, 0.8775825618903720926 ) ) ;
#7896=AXIS2_PLACEMENT_3D ( 'NONE', #3097, #9480, #16329 ) ;
#7898=EDGE_CURVE ( 'NONE', #18837, #7960, #24394, .T. ) ;
#7902=CARTESIAN_POINT ( 'NONE',  ( 19.64032682080000214, -94.52419709919999491, 13.82579343989999998 ) ) ;
#7903=ORIENTED_EDGE ( 'NONE', *, *, #18637, .F. ) ;
#7904=CARTESIAN_POINT ( 'NONE',  ( -12.78466493160000006, -101.0848057460000007, -8.608125847929999352 ) ) ;
#7905=FACE_OUTER_BOUND ( 'NONE', #9447, .T. ) ;
#7906=CARTESIAN_POINT ( 'NONE',  ( -7.696682359570000465, -100.6809449770000100, 14.52276816779999891 ) ) ;
#7907=FACE_OUTER_BOUND ( 'NONE', #5471, .T. ) ;
#7908=FACE_OUTER_BOUND ( 'NONE', #24839, .T. ) ;
#7909=CARTESIAN_POINT ( 'NONE',  ( 7.483210945499999767, -101.1711668239999966, 13.84080871329999773 ) ) ;
#7912=CARTESIAN_POINT ( 'NONE',  ( -23.97050053409999748, -93.63284696379999161, -7.388385114300000112 ) ) ;
#7916=CARTESIAN_POINT ( 'NONE',  ( 11.71858627609999992, -101.1499348409999897, -10.52473037210000051 ) ) ;
#7919=CARTESIAN_POINT ( 'NONE',  ( -17.21128535244866242, -92.77481473473854123, 25.17988932136048064 ) ) ;
#7920=VECTOR ( 'NONE', #14895, 1000.000000000000000 ) ;
#7922=CARTESIAN_POINT ( 'NONE',  ( -0.01895569543850000177, -101.5216621940000152, -16.01048889870000025 ) ) ;
#7925=CARTESIAN_POINT ( 'NONE',  ( 8.185346967789998374, -101.3150701389999995, 14.03998109830000018 ) ) ;
#7927=ORIENTED_EDGE ( 'NONE', *, *, #3723, .F. ) ;
#7928=CARTESIAN_POINT ( 'NONE',  ( 6.749096951940000366, -101.2063419769999939, 14.49232149449999874 ) ) ;
#7929=CARTESIAN_POINT ( 'NONE',  ( 13.87577342641885103, -97.43430234697039793, -15.18291532359526919 ) ) ;
#7941=VERTEX_POINT ( 'NONE', #19053 ) ;
#7946=CARTESIAN_POINT ( 'NONE',  ( 0.5907866879554720674, -100.3796496172627144, -16.98725527372521782 ) ) ;
#7947=CARTESIAN_POINT ( 'NONE',  ( 6.355965434729999863, -99.91102932029998840, 15.68918534660000041 ) ) ;
#7948=DIRECTION ( 'NONE',  ( 1.000000000000000000, 0.000000000000000000, 0.000000000000000000 ) ) ;
#7951=CARTESIAN_POINT ( 'NONE',  ( 20.51721036366772921, -93.01584921895947389, 16.65400312716379005 ) ) ;
#7952=CARTESIAN_POINT ( 'NONE',  ( 23.92053897610000135, -111.0000000000000000, -18.92241567810000191 ) ) ;
#7955=CIRCLE ( 'NONE', #5623, 0.4999999999999990008 ) ;
#7956=VERTEX_POINT ( 'NONE', #21373 ) ;
#7960=VERTEX_POINT ( 'NONE', #19185 ) ;
#7962=CARTESIAN_POINT ( 'NONE',  ( -27.88330092360000023, -92.65715406920001840, 1.774534369700000003 ) ) ;
#7966=B_SPLINE_CURVE_WITH_KNOTS ( 'NONE', 3,
 ( #4640, #26942, #20084, #17467, #6985, #6689, #28529, #26353, #19639, #13518, #4491, #26646 ),
 .UNSPECIFIED., .F., .F.,
 ( 4, 2, 2, 2, 2, 4 ),
 ( 0.000000000000000000, 0.2500000000000262568, 0.3750000000000481837, 0.4375000000000474065, 0.5000000000000466294, 1.000000000000000000 ),
 .UNSPECIFIED. ) ;
#7970=TOROIDAL_SURFACE ( 'NONE', #9840, 21.14285714289999873, 0.5000000000000000000 ) ;
#7977=CARTESIAN_POINT ( 'NONE',  ( -15.39442787059999951, -101.4333525140000063, 4.601335728080000465 ) ) ;
#7978=CARTESIAN_POINT ( 'NONE',  ( -16.54845023329999876, -100.2711349300000023, 3.073083695130000237 ) ) ;
#7980=CARTESIAN_POINT ( 'NONE',  ( -6.285925807789999986, -101.6484611540000031, 14.71350185169999847 ) ) ;
#7985=CARTESIAN_POINT ( 'NONE',  ( -7.685338361321690570, -100.9510322833058495, 14.64991780641961938 ) ) ;
#7988=FACE_OUTER_BOUND ( 'NONE', #17148, .T. ) ;
#7995=CARTESIAN_POINT ( 'NONE',  ( 6.661118870793237612, -100.9616911410331994, 15.13395055016176016 ) ) ;
#7998=ADVANCED_FACE ( 'NONE', ( #6949 ), #111, .F. ) ;
#8000=ORIENTED_EDGE ( 'NONE', *, *, #15909, .T. ) ;
#8001=FACE_OUTER_BOUND ( 'NONE', #20329, .T. ) ;
#8002=CARTESIAN_POINT ( 'NONE',  ( -5.912079742529999571, -101.4309749570000037, 15.04392878760000052 ) ) ;
#8013=CARTESIAN_POINT ( 'NONE',  ( -13.14564498500000056, -99.53431242750001218, -11.42100405340000080 ) ) ;
#8015=CARTESIAN_POINT ( 'NONE',  ( -20.20033130439999880, -94.89196636830000386, 12.35535293270000068 ) ) ;
#8016=CARTESIAN_POINT ( 'NONE',  ( 24.76017301490000122, -92.96321827549999739, -15.38621121709999962 ) ) ;
#8018=CARTESIAN_POINT ( 'NONE',  ( 29.72507353699757715, -92.83865970264098166, 6.831545584289306028 ) ) ;
#8021=CARTESIAN_POINT ( 'NONE',  ( -15.48259164459999937, -101.2306293330000102, 4.813005033020000489 ) ) ;
#8023=CARTESIAN_POINT ( 'NONE',  ( 6.089256317429503795, -92.55389105863930865, 29.05547583162038805 ) ) ;
#8028=B_SPLINE_CURVE_WITH_KNOTS ( 'NONE', 3,
 ( #8410, #15102, #8561, #28234, #13068, #17316 ),
 .UNSPECIFIED., .F., .F.,
 ( 4, 2, 4 ),
 ( 0.000000000000000000, 0.5000000000000000000, 1.000000000000000000 ),
 .UNSPECIFIED. ) ;
#8035=DIRECTION ( 'NONE',  ( 1.000000000000000000, 0.000000000000000000, 0.000000000000000000 ) ) ;
#8036=CARTESIAN_POINT ( 'NONE',  ( 19.60651811670000200, -94.52293512109999085, 13.72233059890000106 ) ) ;
#8038=CARTESIAN_POINT ( 'NONE',  ( 9.119802927630001221, -98.28914429610000525, 16.69368728350000097 ) ) ;
#8039=B_SPLINE_SURFACE_WITH_KNOTS ( 'NONE', 5, 5, ( 
 ( #13220, #9138, #24898, #11462, #4789, #16676, #4636, #24753, #26797 ),
 ( #28658, #10867, #17607, #4929, #6829, #22421, #2027, #26495, #2467 ),
 ( #15392, #2169, #26938, #13667, #11005, #8843, #26639, #17322, #10447 ),
 ( #26501, #10872, #14970, #6538, #8696, #14834, #12783, #15107, #4353 ),
 ( #15246, #23882, #19782, #12919, #28664, #21835, #8566, #23736, #21691 ),
 ( #13225, #15398, #3918, #24313, #3780, #22133, #1889, #1739, #13075 ),
 ( #6383, #5950, #10580, #26064, #17177, #19640, #12641, #4052, #21984 ),
 ( #17612, #19501, #2174, #10726, #19225, #8277, #2032, #28113, #17037 ),
 ( #8150, #25927, #21554, #1609, #24167, #19366, #28385, #17469, #28241 ),
 ( #8416, #26216, #6244, #24019, #6092, #28530, #26354, #4200, #11327 ),
 ( #8848, #6691, #13815, #15998, #16140, #6834, #22720, #18348, #15553 ),
 ( #20085, #4795, #9293, #17909, #1, #2319, #26802, #2473, #2620 ) ),
 .UNSPECIFIED., .F., .F., .F.,
 ( 6, 3, 3, 6 ),
 ( 6, 3, 6 ),
 ( 3.852920539479999906, 4.834764074430000669, 6.134713715070000184, 8.383984506250000024 ),
 ( 0.000000000000000000, 0.2500000000000000000, 0.5000000000000000000 ),
 .UNSPECIFIED. ) ;
#8040=CARTESIAN_POINT ( 'NONE',  ( -18.11118464990000021, -92.50000169800000549, -23.63835352659999955 ) ) ;
#8041=CARTESIAN_POINT ( 'NONE',  ( -8.238075515089999357, -99.92384627689999377, 14.76899840829999988 ) ) ;
#8043=CARTESIAN_POINT ( 'NONE',  ( 3.892082198189999787, -92.58502644590001296, 28.36234172580000390 ) ) ;
#8045=CARTESIAN_POINT ( 'NONE',  ( 7.563340576460000797, -101.3249909679999945, 13.99392069269999972 ) ) ;
#8048=DIRECTION ( 'NONE',  ( 1.000000000000000000, 0.000000000000000000, 0.000000000000000000 ) ) ;
#8056=CARTESIAN_POINT ( 'NONE',  ( -18.17993916029999824, -94.51629284240000572, 17.35042103430000182 ) ) ;
#8058=DIRECTION ( 'NONE',  ( 0.000000000000000000, -1.000000000000000000, 0.000000000000000000 ) ) ;
#8060=CARTESIAN_POINT ( 'NONE',  ( -0.1769176043900000106, -101.3256027139999986, -15.90570293400000246 ) ) ;
#8065=ORIENTED_EDGE ( 'NONE', *, *, #4911, .F. ) ;
#8066=CARTESIAN_POINT ( 'NONE',  ( 6.641904396630000207, -100.8746138070000029, 15.21662664139999954 ) ) ;
#8067=CARTESIAN_POINT ( 'NONE',  ( -17.01539865379871586, -92.51381484706730873, -23.94002819195306841 ) ) ;
#8069=CARTESIAN_POINT ( 'NONE',  ( -5.520527781993984640, -97.05288879771497079, 20.32268517453738710 ) ) ;
#8071=FACE_OUTER_BOUND ( 'NONE', #14249, .T. ) ;
#8073=CARTESIAN_POINT ( 'NONE',  ( 4.413832159080181228, -92.82044061125340306, -30.17893592457920349 ) ) ;
#8074=CARTESIAN_POINT ( 'NONE',  ( -6.595572254019999470, -97.73638926229999413, 18.83567684839999856 ) ) ;
#8076=CARTESIAN_POINT ( 'NONE',  ( 6.595758072439999786, -93.30149055180000062, -26.35103330869999994 ) ) ;
#8078=DIRECTION ( 'NONE',  ( 1.000000000000000000, 0.000000000000000000, 0.000000000000000000 ) ) ;
#8079=ORIENTED_EDGE ( 'NONE', *, *, #14230, .F. ) ;
#8082=CARTESIAN_POINT ( 'NONE',  ( -0.9804619217829999567, -101.6095085860000040, -16.00001407889999783 ) ) ;
#8083=CARTESIAN_POINT ( 'NONE',  ( -17.00715350810000004, -111.0000000000000000, 3.484608414699999823 ) ) ;
#8085=CARTESIAN_POINT ( 'NONE',  ( 13.19216279811974424, -92.83865970264201906, 27.49939731263290099 ) ) ;
#8090=FACE_OUTER_BOUND ( 'NONE', #17030, .T. ) ;
#8096=ORIENTED_EDGE ( 'NONE', *, *, #21049, .T. ) ;
#8107=CIRCLE ( 'NONE', #11831, 0.7500000000000006661 ) ;
#8113=CARTESIAN_POINT ( 'NONE',  ( -15.52809674979999954, -101.4254868729999970, 3.726364514469999722 ) ) ;
#8118=CARTESIAN_POINT ( 'NONE',  ( -12.44238872350000058, -101.2251655520000071, -10.41030240340000113 ) ) ;
#8121=CARTESIAN_POINT ( 'NONE',  ( -7.896941525246588434, -100.4103893717344960, 15.02389615286374180 ) ) ;
#8122=EDGE_LOOP ( 'NONE', ( #11737, #10330, #28260, #6641 ) ) ;
#8131=CARTESIAN_POINT ( 'NONE',  ( 0.000000000000000000, -108.5000000000000000, 0.000000000000000000 ) ) ;
#8132=CARTESIAN_POINT ( 'NONE',  ( 6.860655828344782492, -100.3379349521298565, 15.58801274157079320 ) ) ;
#8146=CARTESIAN_POINT ( 'NONE',  ( 7.318052426040000391, -101.1822553929999913, 13.41977313900000013 ) ) ;
#8149=CARTESIAN_POINT ( 'NONE',  ( -1.604070449259999753, -100.9197075889999979, -15.54198650660000069 ) ) ;
#8150=CARTESIAN_POINT ( 'NONE',  ( 13.58694672230000045, -100.5229262450000078, -10.01978713429999956 ) ) ;
#8152=CARTESIAN_POINT ( 'NONE',  ( 24.28845093110000164, -92.54030566109999256, -15.30821873470000050 ) ) ;
#8159=CARTESIAN_POINT ( 'NONE',  ( -15.03194159329999913, -100.8816813800000034, 4.847769557329999479 ) ) ;
#8170=PLANE ( 'NONE',  #1861 ) ;
#8172=CARTESIAN_POINT ( 'NONE',  ( -12.87035238900000067, -101.3256027139999986, -9.347551286109998969 ) ) ;
#8173=CARTESIAN_POINT ( 'NONE',  ( -15.07852873310000064, -92.61407321170000273, -23.93835657210000178 ) ) ;
#8176=CARTESIAN_POINT ( 'NONE',  ( -1.271815980439999993, -100.9405338520000015, -15.89396502050000137 ) ) ;
#8184=ORIENTED_EDGE ( 'NONE', *, *, #6592, .F. ) ;
#8187=CARTESIAN_POINT ( 'NONE',  ( -17.35994848780000055, -93.69758091459999605, 18.14149070599999902 ) ) ;
#8192=CARTESIAN_POINT ( 'NONE',  ( 0.04086140067849999835, -101.3852859389999992, -15.99338919589999719 ) ) ;
#8197=ORIENTED_EDGE ( 'NONE', *, *, #14848, .T. ) ;
#8198=EDGE_CURVE ( 'NONE', #17518, #14137, #3691, .T. ) ;
#8199=CARTESIAN_POINT ( 'NONE',  ( 6.634701928220000156, -100.3517545579999961, 15.38134052770000082 ) ) ;
#8200=CARTESIAN_POINT ( 'NONE',  ( 15.06296946009999971, -101.0147083550000104, 3.854692841859999941 ) ) ;
#8201=CARTESIAN_POINT ( 'NONE',  ( -5.909937095737705093, -97.43022994549096438, 19.70649122759998662 ) ) ;
#8206=CARTESIAN_POINT ( 'NONE',  ( 3.339696405680000257, -92.65997669530000280, -28.81024678410000206 ) ) ;
#8214=CARTESIAN_POINT ( 'NONE',  ( -1.469243280769999993, -101.0356131030000029, -15.40539586329999899 ) ) ;
#8220=CARTESIAN_POINT ( 'NONE',  ( -15.33274302073847828, -101.3256032149999299, 4.234343774312764985 ) ) ;
#8230=FACE_OUTER_BOUND ( 'NONE', #12781, .T. ) ;
#8231=CARTESIAN_POINT ( 'NONE',  ( -0.6842253573819999657, -101.2530993000000024, -15.17849927279999989 ) ) ;
#8233=ADVANCED_FACE ( 'NONE', ( #23999 ), #24290, .F. ) ;
#8234=CARTESIAN_POINT ( 'NONE',  ( 15.93242396329999977, -100.7430069139999915, 4.261870627000000411 ) ) ;
#8242=CARTESIAN_POINT ( 'NONE',  ( -7.441474466189999859, -94.70873790539999959, -22.49465953780000049 ) ) ;
#8244=CARTESIAN_POINT ( 'NONE',  ( -14.81560312829999937, -101.2530993080000030, 3.374019817609999805 ) ) ;
#8248=CARTESIAN_POINT ( 'NONE',  ( 17.74427621692063894, -100.1470170784672149, 1.201385877241859967 ) ) ;
#8249=CARTESIAN_POINT ( 'NONE',  ( -12.45064030709999869, -101.3090757639999993, -10.46249930100000114 ) ) ;
#8250=CARTESIAN_POINT ( 'NONE',  ( 20.34398966297630196, -93.66270333196790432, 16.17952385861759979 ) ) ;
#8251=CARTESIAN_POINT ( 'NONE',  ( -6.858401400031342909, -101.6484611539999747, 14.45577953271265059 ) ) ;
#8252=ORIENTED_EDGE ( 'NONE', *, *, #24639, .T. ) ;
#8255=ORIENTED_EDGE ( 'NONE', *, *, #19373, .F. ) ;
#8259=ORIENTED_EDGE ( 'NONE', *, *, #21359, .T. ) ;
#8263=ORIENTED_EDGE ( 'NONE', *, *, #19373, .T. ) ;
#8266=ORIENTED_EDGE ( 'NONE', *, *, #5285, .T. ) ;
#8269=ADVANCED_FACE ( 'NONE', ( #15377 ), #21953, .F. ) ;
#8272=CARTESIAN_POINT ( 'NONE',  ( 21.75659477429999811, -93.00000000000000000, -13.30039788230000042 ) ) ;
#8276=CARTESIAN_POINT ( 'NONE',  ( -14.99536030859999869, -98.58303758080000989, -11.15547849020000015 ) ) ;
#8277=CARTESIAN_POINT ( 'NONE',  ( 13.21950097729999918, -100.5027207520000019, -9.453354134850000534 ) ) ;
#8278=CARTESIAN_POINT ( 'NONE',  ( -19.58495966999999993, -92.85282696620001275, 20.69528026369999907 ) ) ;
#8279=CARTESIAN_POINT ( 'NONE',  ( 24.70831025289999872, -92.79907188629998416, -15.37124366699999989 ) ) ;
#8284=CIRCLE ( 'NONE', #16667, 5.000000000000000888 ) ;
#8290=B_SPLINE_CURVE_WITH_KNOTS ( 'NONE', 3,
 ( #21952, #1999, #10841, #19750, #10281, #9406, #22545, #20199, #18315, #24868, #2728, #13637, #272, #27059, #24568, #9114, #26772, #22392, #27203, #11583, #13191, #17730, #7243, #7101, #15964, #16108, #26913, #6804, #19895, #17873, #18160, #26613, #6653, #2287, #2589, #15815, #4902, #22099, #25008, #15665, #2142, #18014, #8814, #24727, #13484, #15516, #6953, #20052, #115, #4761, #11436, #10979 ),
 .UNSPECIFIED., .F., .F.,
 ( 4, 2, 2, 1, 1, 1, 1, 2, 2, 2, 2, 1, 1, 1, 1, 1, 2, 2, 2, 2, 1, 1, 2, 2, 2, 2, 1, 1, 1, 1, 1, 2, 2, 4 ),
 ( 0.000000000000000000, 0.1249999999999993339, 0.1874999999999988343, 0.2187499999999984457, 0.2343749999999982514, 0.2421874999999974742, 0.2460937499999971967, 0.2480468749999965861, 0.2499999999999960032, 0.3750000000000502931, 0.4375000000000773270, 0.4687500000000909273, 0.4843750000000984213, 0.4921875000001021405, 0.4960937500001039724, 0.4980468750001043055, 0.4990234375001045275, 0.5000000000001048051, 0.5625000000001960654, 0.5937500000002408074, 0.6093750000002631229, 0.6171875000002737810, 0.6210937500002799982, 0.6250000000002862155, 0.6875000000003996803, 0.7187500000004555245, 0.7343750000004828360, 0.7421875000004953815, 0.7460937500005029310, 0.7480468750005067058, 0.7490234375005088152, 0.7495117187505085932, 0.7500000000005083711, 1.000000000000000000 ),
 .UNSPECIFIED. ) ;
#8292=DIRECTION ( 'NONE',  ( 0.000000000000000000, -1.000000000000000000, 0.000000000000000000 ) ) ;
#8293=DIRECTION ( 'NONE',  ( 0.000000000000000000, 1.000000000000000000, 0.000000000000000000 ) ) ;
#8297=ORIENTED_EDGE ( 'NONE', *, *, #13150, .T. ) ;
#8298=CARTESIAN_POINT ( 'NONE',  ( -12.73176082490000027, -101.1045726949999874, -8.901570339680000998 ) ) ;
#8302=CARTESIAN_POINT ( 'NONE',  ( -13.18688158500000007, -93.32822950609998713, -23.58441611189999776 ) ) ;
#8303=CARTESIAN_POINT ( 'NONE',  ( -2.743624554930000237, -99.80676450699999691, -17.57271110129999769 ) ) ;
#8305=DIRECTION ( 'NONE',  ( 0.8960873909912637769, 0.000000000000000000, -0.4438776720071309079 ) ) ;
#8308=CARTESIAN_POINT ( 'NONE',  ( 13.11884685345288304, -101.1451610291512964, -9.826322704137346875 ) ) ;
#8315=CARTESIAN_POINT ( 'NONE',  ( -17.63662161710000120, -94.54718950359999496, 16.06392408140000327 ) ) ;
#8316=DIRECTION ( 'NONE',  ( -0.9206947212159483085, 0.000000000000000000, 0.3902835255619780952 ) ) ;
#8317=ORIENTED_EDGE ( 'NONE', *, *, #3212, .T. ) ;
#8322=CARTESIAN_POINT ( 'NONE',  ( 15.81703362330000040, -101.6095085860000040, 2.604458381759999774 ) ) ;
#8325=ORIENTED_EDGE ( 'NONE', *, *, #18579, .F. ) ;
#8328=CARTESIAN_POINT ( 'NONE',  ( 6.018657797749999538, -100.4792519539999915, 15.03391506150000012 ) ) ;
#8329=CARTESIAN_POINT ( 'NONE',  ( 15.62063516470000124, -101.5369810359999860, 3.464403400670000188 ) ) ;
#8331=CARTESIAN_POINT ( 'NONE',  ( 6.258798239620000814, -92.50000000000000000, -29.85092033080000107 ) ) ;
#8332=ADVANCED_FACE ( 'NONE', ( #15977 ), #22995, .T. ) ;
#8335=CARTESIAN_POINT ( 'NONE',  ( 8.074823624729997817, -93.81709628030000658, -24.47602660240000105 ) ) ;
#8336=EDGE_CURVE ( 'NONE', #23975, #25484, #28358, .T. ) ;
#8338=CARTESIAN_POINT ( 'NONE',  ( -6.807494426549999922, -101.1617736559999940, 14.19398353890000131 ) ) ;
#8342=CARTESIAN_POINT ( 'NONE',  ( -12.60783569927363601, -100.8738282927339043, -10.80472408861342437 ) ) ;
#8347=ADVANCED_FACE ( 'NONE', ( #18905 ), #16703, .T. ) ;
#8348=AXIS2_PLACEMENT_3D ( 'NONE', #22949, #23364, #3407 ) ;
#8349=CARTESIAN_POINT ( 'NONE',  ( -1.137727369580000092, -101.2490009469999990, -16.04170511839999946 ) ) ;
#8352=CARTESIAN_POINT ( 'NONE',  ( 13.12517053680000068, -93.00000000000000000, 27.53143473160000099 ) ) ;
#8353=CARTESIAN_POINT ( 'NONE',  ( 16.25687204636146177, -94.67499508575106404, 17.23253240788842078 ) ) ;
#8357=CARTESIAN_POINT ( 'NONE',  ( 24.32621394512662860, -94.00303307109788875, -9.416846555509286176 ) ) ;
#8360=DIRECTION ( 'NONE',  ( 0.000000000000000000, 1.000000000000000000, 0.000000000000000000 ) ) ;
#8367=CARTESIAN_POINT ( 'NONE',  ( 16.83483077069999823, -111.0000000000000000, 4.239603657359999112 ) ) ;
#8375=ORIENTED_EDGE ( 'NONE', *, *, #14196, .F. ) ;
#8380=VECTOR ( 'NONE', #23162, 1000.000000000000000 ) ;
#8386=CARTESIAN_POINT ( 'NONE',  ( -12.05323405150000049, -101.1848541609999899, -9.394733094839999410 ) ) ;
#8388=CARTESIAN_POINT ( 'NONE',  ( -7.679059309326275340, -100.9616911410546578, 14.64373627150416546 ) ) ;
#8394=ORIENTED_EDGE ( 'NONE', *, *, #15047, .T. ) ;
#8395=CARTESIAN_POINT ( 'NONE',  ( 6.668334764284620242, -100.8945630386159706, 15.18849496292583545 ) ) ;
#8405=AXIS2_PLACEMENT_3D ( 'NONE', #22541, #15661, #21949 ) ;
#8406=CARTESIAN_POINT ( 'NONE',  ( 8.074115162410000934, -92.66424957140000629, 26.74225754210000261 ) ) ;
#8408=CARTESIAN_POINT ( 'NONE',  ( -6.860733622652498198, -95.36087494180328861, -22.20122310548567057 ) ) ;
#8410=CARTESIAN_POINT ( 'NONE',  ( -29.91144828099999842, -92.50000000000000000, -0.6532076026720000650 ) ) ;
#8411=CARTESIAN_POINT ( 'NONE',  ( -18.86782185830000103, -92.76550115769998683, -21.02010845870000111 ) ) ;
#8414=CARTESIAN_POINT ( 'NONE',  ( -18.73266888770000094, -96.73974214399999028, -10.02540521279999908 ) ) ;
#8416=CARTESIAN_POINT ( 'NONE',  ( 13.70361515709999978, -100.3063911739999980, -10.15418389529999921 ) ) ;
#8419=B_SPLINE_CURVE_WITH_KNOTS ( 'NONE', 3,
 ( #23460, #12358, #16897, #3633, #2310, #294, #11161, #26796, #4191, #11003 ),
 .UNSPECIFIED., .F., .F.,
 ( 4, 2, 2, 2, 4 ),
 ( 0.000000000000000000, 0.2500000000000000000, 0.5000000000000000000, 0.7500000000000000000, 1.000000000000000000 ),
 .UNSPECIFIED. ) ;
#8429=CARTESIAN_POINT ( 'NONE',  ( 22.71044028429788852, -95.75133629245080158, -1.098555083257358289 ) ) ;
#8431=CARTESIAN_POINT ( 'NONE',  ( -0.3395873122069730243, -92.62938374248859930, -30.49812602705775078 ) ) ;
#8432=DIRECTION ( 'NONE',  ( 0.000000000000000000, 1.000000000000000000, 0.000000000000000000 ) ) ;
#8433=ADVANCED_FACE ( 'NONE', ( #8230 ), #16157, .T. ) ;
#8435=EDGE_CURVE ( 'NONE', #24426, #19799, #10190, .T. ) ;
#8436=EDGE_CURVE ( 'NONE', #19835, #3921, #16733, .T. ) ;
#8445=CARTESIAN_POINT ( 'NONE',  ( -13.08734813130000063, -101.2459394079999981, -9.124757622539998891 ) ) ;
#8448=CARTESIAN_POINT ( 'NONE',  ( -0.07556308132799999244, -93.13207089459999111, 26.24589193079999916 ) ) ;
#8449=CARTESIAN_POINT ( 'NONE',  ( -30.34790777679999962, -93.00000000000000000, 3.042119914239999723 ) ) ;
#8451=CARTESIAN_POINT ( 'NONE',  ( -29.62058833974716165, -92.58608763742402914, 7.271233193961131214 ) ) ;
#8452=DIRECTION ( 'NONE',  ( 0.000000000000000000, 1.000000000000000000, 0.000000000000000000 ) ) ;
#8453=VERTEX_POINT ( 'NONE', #8367 ) ;
#8454=CARTESIAN_POINT ( 'NONE',  ( 13.07944802186373856, -101.1884902309573704, -9.822393493178296353 ) ) ;
#8457=CARTESIAN_POINT ( 'NONE',  ( 7.073120017670000870, -99.73367811500000357, 15.79835279589999963 ) ) ;
#8458=ORIENTED_EDGE ( 'NONE', *, *, #6512, .F. ) ;
#8462=CARTESIAN_POINT ( 'NONE',  ( -20.43932202180000246, -94.59276292389999696, 12.18704577789999988 ) ) ;
#8463=EDGE_LOOP ( 'NONE', ( #20502, #16023, #24854, #2061 ) ) ;
#8466=AXIS2_PLACEMENT_3D ( 'NONE', #26243, #21861, #1913 ) ;
#8467=CARTESIAN_POINT ( 'NONE',  ( -0.1724647388530000103, -101.1292389600000092, -15.50536992770000033 ) ) ;
#8469=CARTESIAN_POINT ( 'NONE',  ( 15.23243409989999897, -101.1130130960000031, 2.433086515549999884 ) ) ;
#8475=CARTESIAN_POINT ( 'NONE',  ( 6.410511849489999747, -99.92384627689999377, 15.64910668389999771 ) ) ;
#8476=CARTESIAN_POINT ( 'NONE',  ( -17.28030528624062967, -92.50821026832076655, -23.91007388581562054 ) ) ;
#8477=EDGE_CURVE ( 'NONE', #7330, #24436, #17421, .T. ) ;
#8481=CARTESIAN_POINT ( 'NONE',  ( 5.525098516430999140, -92.56492639272521217, -29.99554189593663622 ) ) ;
#8484=CARTESIAN_POINT ( 'NONE',  ( 1.761322637119999923, -92.49537389370000540, -29.34428460070000000 ) ) ;
#8486=CARTESIAN_POINT ( 'NONE',  ( -23.50862727400000196, -94.59276292389999696, -3.692480628369999796 ) ) ;
#8487=CARTESIAN_POINT ( 'NONE',  ( -6.714989711430000341, -101.1700440390000040, 13.74992627059999961 ) ) ;
#8489=CARTESIAN_POINT ( 'NONE',  ( -13.15133833870000046, -100.9197081840000010, -8.436152112259998503 ) ) ;
#8491=CARTESIAN_POINT ( 'NONE',  ( -12.97150031818777016, -100.3041487039710518, -11.07791448419877511 ) ) ;
#8492=VERTEX_POINT ( 'NONE', #27183 ) ;
#8495=CARTESIAN_POINT ( 'NONE',  ( 23.70295720520000060, -94.59276479689999917, -2.111852433950000218 ) ) ;
#8500=CARTESIAN_POINT ( 'NONE',  ( -19.85646363226101840, -92.53708507728565280, -23.15107591307967994 ) ) ;
#8502=CARTESIAN_POINT ( 'NONE',  ( 0.4184115225550000261, -93.00000000000000000, -30.38020727889999861 ) ) ;
#8503=CARTESIAN_POINT ( 'NONE',  ( 16.42966103859999905, -94.59276292389999696, 17.21499949629999904 ) ) ;
#8514=AXIS2_PLACEMENT_3D ( 'NONE', #23004, #24750, #13955 ) ;
#8520=FACE_OUTER_BOUND ( 'NONE', #15092, .T. ) ;
#8525=DIRECTION ( 'NONE',  ( 0.000000000000000000, 1.000000000000000000, 0.000000000000000000 ) ) ;
#8527=DIRECTION ( 'NONE',  ( 0.000000000000000000, -1.000000000000000000, 0.000000000000000000 ) ) ;
#8532=CARTESIAN_POINT ( 'NONE',  ( -23.50862727400000196, -94.59276292389999696, -3.692480628369999796 ) ) ;
#8533=CARTESIAN_POINT ( 'NONE',  ( -13.14571786560000000, -100.8733988930000010, -8.628954981190000595 ) ) ;
#8536=CARTESIAN_POINT ( 'NONE',  ( -11.77131553929999974, -101.2010924020000004, -9.714008462309999814 ) ) ;
#8538=CARTESIAN_POINT ( 'NONE',  ( -6.781378104809999030, -101.6484611540000031, 14.49182221120000058 ) ) ;
#8541=AXIS2_PLACEMENT_3D ( 'NONE', #11477, #20383, #6842 ) ;
#8546=CARTESIAN_POINT ( 'NONE',  ( -11.84764223884960010, -93.03217576144683676, -23.86221593305796063 ) ) ;
#8547=ORIENTED_EDGE ( 'NONE', *, *, #22780, .T. ) ;
#8552=CARTESIAN_POINT ( 'NONE',  ( -16.97479393769052436, -93.48480241359186493, -21.44694654164490188 ) ) ;
#8554=CARTESIAN_POINT ( 'NONE',  ( 26.20138505510000115, -92.90721318149999775, 10.82755978760000204 ) ) ;
#8555=DIRECTION ( 'NONE',  ( -0.2333505288839994030, 1.612292758439994142E-16, -0.9723926833689966465 ) ) ;
#8556=ORIENTED_EDGE ( 'NONE', *, *, #23044, .F. ) ;
#8560=ORIENTED_EDGE ( 'NONE', *, *, #14386, .F. ) ;
#8561=CARTESIAN_POINT ( 'NONE',  ( -29.68198139278343461, -92.55389105863635280, -0.5288656702900278450 ) ) ;
#8562=CARTESIAN_POINT ( 'NONE',  ( -23.36079593639999885, -92.54628605920001405, -19.03433440690000111 ) ) ;
#8564=ORIENTED_EDGE ( 'NONE', *, *, #10874, .F. ) ;
#8565=CARTESIAN_POINT ( 'NONE',  ( -1.271820802479999957, -100.9405348700000076, -15.89396400309999891 ) ) ;
#8566=CARTESIAN_POINT ( 'NONE',  ( 12.40532806309999891, -101.0147083550000104, -9.373342067159999402 ) ) ;
#8573=CARTESIAN_POINT ( 'NONE',  ( -11.32307664120000013, -93.00000000000000000, 9.421136869679999748 ) ) ;
#8574=EDGE_CURVE ( 'NONE', #24926, #11541, #24022, .T. ) ;
#8576=CARTESIAN_POINT ( 'NONE',  ( -23.79797125454739515, -92.87422005959625437, -19.07634091649623542 ) ) ;
#8581=CARTESIAN_POINT ( 'NONE',  ( -11.25326567110000120, -94.84395216780001192, -20.59896464009999661 ) ) ;
#8582=DIRECTION ( 'NONE',  ( 0.000000000000000000, 1.000000000000000000, 0.000000000000000000 ) ) ;
#8585=CARTESIAN_POINT ( 'NONE',  ( 15.91666814759999937, -101.0685845459999967, 2.371727654049999856 ) ) ;
#8586=ORIENTED_EDGE ( 'NONE', *, *, #21224, .T. ) ;
#8592=CARTESIAN_POINT ( 'NONE',  ( -16.07900805970000135, -92.88046764189999749, -23.59102352649999901 ) ) ;
#8594=CARTESIAN_POINT ( 'NONE',  ( -6.644771110830000715, -97.11988490479998859, -19.57974298529999757 ) ) ;
#8599=ORIENTED_EDGE ( 'NONE', *, *, #3531, .T. ) ;
#8600=CARTESIAN_POINT ( 'NONE',  ( 13.09247055681168348, -101.1742791178134411, -9.823544259465782247 ) ) ;
#8607=CARTESIAN_POINT ( 'NONE',  ( -14.34532190269999852, -92.62623300010000094, 26.10005267279999686 ) ) ;
#8608=CARTESIAN_POINT ( 'NONE',  ( -20.66035133919229949, -93.50335891207949146, 15.02327711490973172 ) ) ;
#8609=ORIENTED_EDGE ( 'NONE', *, *, #12413, .F. ) ;
#8611=CARTESIAN_POINT ( 'NONE',  ( 0.6965880932790000646, -100.8815367389999977, -15.65919131430000277 ) ) ;
#8612=CARTESIAN_POINT ( 'NONE',  ( -14.42556421679999978, -111.0000000000000000, -2.978755036369999942 ) ) ;
#8616=VERTEX_POINT ( 'NONE', #25300 ) ;
#8618=CARTESIAN_POINT ( 'NONE',  ( -15.59566370272417046, -92.58075529924404634, -24.03361414823421072 ) ) ;
#8619=CARTESIAN_POINT ( 'NONE',  ( 27.81583421292586067, -92.50638022835023833, 12.51200364096112949 ) ) ;
#8621=CARTESIAN_POINT ( 'NONE',  ( 3.129685915889999670, -92.55031878719999838, -28.46238550929999889 ) ) ;
#8622=CARTESIAN_POINT ( 'NONE',  ( 6.766442258106934560, -101.4728631013423268, 14.64836155655668648 ) ) ;
#8625=CARTESIAN_POINT ( 'NONE',  ( -12.78944265896493881, -100.5550990431279672, -10.98195346763384528 ) ) ;
#8628=EDGE_CURVE ( 'NONE', #17884, #8673, #18471, .T. ) ;
#8632=CARTESIAN_POINT ( 'NONE',  ( -1.133529748880000021, -101.1659666750000071, -15.97345870559999881 ) ) ;
#8635=CARTESIAN_POINT ( 'NONE',  ( -20.78903514689297793, -92.80045754870498342, -22.31742311452316585 ) ) ;
#8636=ORIENTED_EDGE ( 'NONE', *, *, #12108, .T. ) ;
#8638=CARTESIAN_POINT ( 'NONE',  ( -15.36545425250000108, -101.4254867220000023, 4.349819274109999689 ) ) ;
#8643=CARTESIAN_POINT ( 'NONE',  ( 13.73273575384635414, -100.1994045927716712, -10.26021908260778659 ) ) ;
#8649=EDGE_LOOP ( 'NONE', ( #26644, #16213, #25374, #10095 ) ) ;
#8654=CARTESIAN_POINT ( 'NONE',  ( -24.63095457940000088, -94.45168166349999694, -3.620300214920000315 ) ) ;
#8656=B_SPLINE_CURVE_WITH_KNOTS ( 'NONE', 3,
 ( #20599, #658, #9511, #7340, #18413, #25118, #14033, #22939, #2979, #11838, #9651, #18557, #27451, #16932, #19253 ),
 .UNSPECIFIED., .F., .F.,
 ( 4, 2, 2, 1, 1, 1, 2, 2, 4 ),
 ( 0.000000000000000000, 0.2499999999999624745, 0.3749999999999431566, 0.4374999999999333866, 0.4687499999999291123, 0.4843749999999272804, 0.4921874999999277800, 0.4999999999999282796, 1.000000000000000000 ),
 .UNSPECIFIED. ) ;
#8658=ORIENTED_EDGE ( 'NONE', *, *, #26998, .T. ) ;
#8660=FACE_OUTER_BOUND ( 'NONE', #8869, .T. ) ;
#8667=CARTESIAN_POINT ( 'NONE',  ( -15.51746188589999953, -101.3079808070000070, 3.547079192720000052 ) ) ;
#8673=VERTEX_POINT ( 'NONE', #16539 ) ;
#8679=CARTESIAN_POINT ( 'NONE',  ( 12.78866345099999968, -92.54627856989999657, 27.28520986150000027 ) ) ;
#8681=CARTESIAN_POINT ( 'NONE',  ( -12.27720009871537776, -94.79128788117789384, -21.50236666293719878 ) ) ;
#8683=CARTESIAN_POINT ( 'NONE',  ( 21.12092159740000241, -93.86380950250000410, 13.35475519379999909 ) ) ;
#8685=EDGE_LOOP ( 'NONE', ( #8599, #17655, #5673, #26632 ) ) ;
#8688=EDGE_CURVE ( 'NONE', #16619, #26053, #21384, .T. ) ;
#8691=CARTESIAN_POINT ( 'NONE',  ( -16.39360122190000268, -92.99570653139998910, -21.25352984659999933 ) ) ;
#8693=VERTEX_POINT ( 'NONE', #21063 ) ;
#8694=EDGE_CURVE ( 'NONE', #24500, #842, #28171, .T. ) ;
#8696=CARTESIAN_POINT ( 'NONE',  ( 12.35324891399999991, -101.1417990620000040, -9.783258604670001191 ) ) ;
#8698=CARTESIAN_POINT ( 'NONE',  ( -11.80896971761302794, -94.89420224084436484, -21.43714084844935641 ) ) ;
#8699=CIRCLE ( 'NONE', #22207, 20.64285714289999873 ) ;
#8703=VERTEX_POINT ( 'NONE', #1526 ) ;
#8706=CARTESIAN_POINT ( 'NONE',  ( 8.831064126840001194, -94.59276292389999696, -22.09756266850000017 ) ) ;
#8708=CARTESIAN_POINT ( 'NONE',  ( -0.5776010673831374342, -92.56772982776919889, -30.49459145784739533 ) ) ;
#8714=CARTESIAN_POINT ( 'NONE',  ( 22.14044571250000004, -95.71128647349999596, -4.387446428019999622 ) ) ;
#8716=B_SPLINE_CURVE_WITH_KNOTS ( 'NONE', 5,
 ( #15739, #14298, #28118, #12239, #21153, #1208 ),
 .UNSPECIFIED., .F., .F.,
 ( 6, 6 ),
 ( 0.000000000000000000, 1.000000000000000000 ),
 .UNSPECIFIED. ) ;
#8723=ADVANCED_FACE ( 'NONE', ( #25713 ), #116, .T. ) ;
#8724=B_SPLINE_CURVE_WITH_KNOTS ( 'NONE', 3,
 ( #19478, #17020, #5804, #3761, #12624, #21536, #22253, #6817, #24439, #20067 ),
 .UNSPECIFIED., .F., .F.,
 ( 4, 2, 2, 2, 4 ),
 ( 0.000000000000000000, 0.2500000000000000000, 0.5000000000000000000, 0.7500000000000000000, 1.000000000000000000 ),
 .UNSPECIFIED. ) ;
#8726=CARTESIAN_POINT ( 'NONE',  ( -14.08277339220000179, -92.72294953669999984, -23.91615244109999949 ) ) ;
#8728=CARTESIAN_POINT ( 'NONE',  ( -26.32352847549999808, -93.13202907830000754, -0.6218978954889999855 ) ) ;
#8729=CARTESIAN_POINT ( 'NONE',  ( -20.10936447829999807, -95.60043714340001486, 10.20867317439999944 ) ) ;
#8730=CARTESIAN_POINT ( 'NONE',  ( -29.65790904711468912, -92.62938374240729900, 7.117544636880208664 ) ) ;
#8733=AXIS2_PLACEMENT_3D ( 'NONE', #19930, #11175, #13522 ) ;
#8738=ORIENTED_EDGE ( 'NONE', *, *, #7719, .T. ) ;
#8740=CARTESIAN_POINT ( 'NONE',  ( -15.53919574999999931, -92.59715193510000120, 23.72508021810000045 ) ) ;
#8741=CARTESIAN_POINT ( 'NONE',  ( 26.58750744064022342, -92.65509297688441848, -7.785012216743809610 ) ) ;
#8745=CARTESIAN_POINT ( 'NONE',  ( 0.2554224435499999890, -101.2010924020000004, -15.25977029010000052 ) ) ;
#8747=CARTESIAN_POINT ( 'NONE',  ( 15.71280846430000366, -101.4254868729999970, 2.848724509360000212 ) ) ;
#8750=EDGE_CURVE ( 'NONE', #14137, #16242, #28591, .T. ) ;
#8759=CARTESIAN_POINT ( 'NONE',  ( -19.97974349676479378, -95.94979037552315049, 10.41052685295677982 ) ) ;
#8763=CARTESIAN_POINT ( 'NONE',  ( -6.569756907160000381, -101.2530993010000060, 13.70087252790000143 ) ) ;
#8764=VERTEX_POINT ( 'NONE', #15309 ) ;
#8766=CARTESIAN_POINT ( 'NONE',  ( -13.09565534707698298, -100.1585711159101777, -11.11278395076808501 ) ) ;
#8767=ORIENTED_EDGE ( 'NONE', *, *, #17642, .F. ) ;
#8769=CARTESIAN_POINT ( 'NONE',  ( 23.58467268920000137, -94.98812656910000385, -2.405348287990000333 ) ) ;
#8770=CARTESIAN_POINT ( 'NONE',  ( 8.765232847019998275, -98.65049302040000612, 16.41568421879999917 ) ) ;
#8773=CIRCLE ( 'NONE', #12493, 5.500000000000000000 ) ;
#8775=CARTESIAN_POINT ( 'NONE',  ( -14.94683085009999957, -101.1292394720000090, 4.127768892550000679 ) ) ;
#8779=AXIS2_PLACEMENT_3D ( 'NONE', #11170, #148, #8999 ) ;
#8784=DIRECTION ( 'NONE',  ( 0.000000000000000000, -1.000000000000000000, 0.000000000000000000 ) ) ;
#8786=CARTESIAN_POINT ( 'NONE',  ( 22.38748998554977021, -94.04667188344215845, 13.21713613643446550 ) ) ;
#8790=EDGE_CURVE ( 'NONE', #9549, #9768, #7461, .T. ) ;
#8796=CARTESIAN_POINT ( 'NONE',  ( -24.82370543889999936, -93.86380869120000625, -2.868192742509999782 ) ) ;
#8802=CARTESIAN_POINT ( 'NONE',  ( 15.87132499590000023, -100.6809449770000100, 4.272090527209999600 ) ) ;
#8803=EDGE_LOOP ( 'NONE', ( #16857, #5973, #16449, #17122 ) ) ;
#8814=CARTESIAN_POINT ( 'NONE',  ( -16.12089651170244053, -99.24541079440805902, 7.516693469902168800 ) ) ;
#8817=CARTESIAN_POINT ( 'NONE',  ( -12.27960098470000005, -100.1275643909999928, -11.24051300700000056 ) ) ;
#8828=CARTESIAN_POINT ( 'NONE',  ( -18.24886321459684524, -94.80026206438209613, 16.23660667693922477 ) ) ;
#8831=DIRECTION ( 'NONE',  ( 0.000000000000000000, 1.000000000000000000, 0.000000000000000000 ) ) ;
#8832=ORIENTED_EDGE ( 'NONE', *, *, #1406, .T. ) ;
#8843=CARTESIAN_POINT ( 'NONE',  ( 12.14638440039999878, -101.1180794200000008, -9.660115219679999754 ) ) ;
#8844=CARTESIAN_POINT ( 'NONE',  ( -16.37879490400000293, -92.97898997919999431, -21.15867040639999885 ) ) ;
#8848=CARTESIAN_POINT ( 'NONE',  ( 13.78612279620000081, -100.0994409990000094, -10.32398801709999958 ) ) ;
#8855=CARTESIAN_POINT ( 'NONE',  ( 0.000000000000000000, -92.50000000000000000, 0.000000000000000000 ) ) ;
#8857=DIRECTION ( 'NONE',  ( 0.000000000000000000, 1.000000000000000000, 0.000000000000000000 ) ) ;
#8859=CARTESIAN_POINT ( 'NONE',  ( -0.8435683774100874999, -92.52640451561843804, -30.48833712424519149 ) ) ;
#8860=CIRCLE ( 'NONE', #19559, 0.4999999999999995559 ) ;
#8865=CARTESIAN_POINT ( 'NONE',  ( -6.285925807789999986, -101.1889999979999999, 14.71350185169999847 ) ) ;
#8867=ORIENTED_EDGE ( 'NONE', *, *, #14950, .F. ) ;
#8868=CARTESIAN_POINT ( 'NONE',  ( 21.03420648150000360, -97.01677119799998650, -2.189672962029999947 ) ) ;
#8869=EDGE_LOOP ( 'NONE', ( #26986, #26205, #10395, #10328 ) ) ;
#8871=CARTESIAN_POINT ( 'NONE',  ( -16.33619708059999809, -101.1889999979999999, 3.920288885250000188 ) ) ;
#8874=CARTESIAN_POINT ( 'NONE',  ( -4.536235172729999654, -98.62857337580000205, -18.99292533490000068 ) ) ;
#8876=CARTESIAN_POINT ( 'NONE',  ( 1.495914020609999895, -94.52293512119999264, 23.88472631159999793 ) ) ;
#8882=CARTESIAN_POINT ( 'NONE',  ( 11.37272679149999988, -93.24058218660000819, -23.59428585010000035 ) ) ;
#8883=VECTOR ( 'NONE', #20703, 1000.000000000000000 ) ;
#8887=ORIENTED_EDGE ( 'NONE', *, *, #21049, .F. ) ;
#8889=CARTESIAN_POINT ( 'NONE',  ( -18.01708526109999653, -94.13770192399999814, 18.41653692539999909 ) ) ;
#8891=EDGE_LOOP ( 'NONE', ( #25499, #14631, #19097, #4308, #21569, #24524, #3674 ) ) ;
#8893=CARTESIAN_POINT ( 'NONE',  ( 0.4823327075950000209, -101.1976625110000043, -16.34256275559999949 ) ) ;
#8899=FACE_OUTER_BOUND ( 'NONE', #2969, .T. ) ;
#8904=CARTESIAN_POINT ( 'NONE',  ( 28.43118412462271749, -92.81370807102868525, 11.04165370930220291 ) ) ;
#8906=CARTESIAN_POINT ( 'NONE',  ( -4.556385078139999933, -95.60035679210000126, 22.08725204710000156 ) ) ;
#8907=ORIENTED_EDGE ( 'NONE', *, *, #17445, .T. ) ;
#8908=CARTESIAN_POINT ( 'NONE',  ( 23.60108036107897789, -92.61393927529991288, -19.31944997532723818 ) ) ;
#8909=CARTESIAN_POINT ( 'NONE',  ( 26.37318040470000113, -92.84292488370000740, 13.16123784829999899 ) ) ;
#8913=CARTESIAN_POINT ( 'NONE',  ( -7.139781038299999771, -101.0403179300000005, 13.72406621880000088 ) ) ;
#8915=LINE ( 'NONE', #4419, #18040 ) ;
#8916=CARTESIAN_POINT ( 'NONE',  ( -12.92645032892205137, -100.3617719037092400, -11.05940935245897627 ) ) ;
#8920=CARTESIAN_POINT ( 'NONE',  ( 7.873312524909999333, -99.14867886189999524, 16.15069897069999882 ) ) ;
#8930=CARTESIAN_POINT ( 'NONE',  ( 14.59338748251070506, -95.47757552516759461, 17.32730085737816950 ) ) ;
#8932=CARTESIAN_POINT ( 'NONE',  ( 26.37318901919999803, -93.00000450890000536, 13.16123549989999830 ) ) ;
#8933=DIRECTION ( 'NONE',  ( -0.8981584475625417063, 0.000000000000000000, -0.4396719266362648648 ) ) ;
#8935=CARTESIAN_POINT ( 'NONE',  ( 23.00000922585108043, -93.86130746320593232, 12.91398536192384050 ) ) ;
#8939=ADVANCED_FACE ( 'NONE', ( #7042 ), #20595, .F. ) ;
#8940=ORIENTED_EDGE ( 'NONE', *, *, #6978, .F. ) ;
#8944=CARTESIAN_POINT ( 'NONE',  ( -24.26314771630000067, -94.16701134380001292, -3.424815318739999892 ) ) ;
#8949=VERTEX_POINT ( 'NONE', #16780 ) ;
#8953=CARTESIAN_POINT ( 'NONE',  ( 7.894252205549937784, -92.54383083955175948, 29.46067132498288643 ) ) ;
#8956=EDGE_CURVE ( 'NONE', #5288, #10781, #12680, .T. ) ;
#8957=CARTESIAN_POINT ( 'NONE',  ( 19.98296175649999995, -94.98812477599999227, 14.17692170039999944 ) ) ;
#8962=CARTESIAN_POINT ( 'NONE',  ( 24.25366699300000306, -93.99830544900000007, -8.983265665619999396 ) ) ;
#8966=CARTESIAN_POINT ( 'NONE',  ( 14.04045377689999796, -98.83667233820000320, -12.27759081110000139 ) ) ;
#8970=DIRECTION ( 'NONE',  ( 0.000000000000000000, 1.000000000000000000, 0.000000000000000000 ) ) ;
#8971=CARTESIAN_POINT ( 'NONE',  ( -12.85008966630000060, -99.72202992580000114, -11.39236235390000118 ) ) ;
#8986=CARTESIAN_POINT ( 'NONE',  ( 19.83535700790000078, -94.71481161159999829, 14.13921680270000003 ) ) ;
#8989=AXIS2_PLACEMENT_3D ( 'NONE', #10545, #24127, #26323 ) ;
#8993=FACE_OUTER_BOUND ( 'NONE', #1052, .T. ) ;
#8995=CARTESIAN_POINT ( 'NONE',  ( -12.45881531480000071, -94.16309976670001447, -20.99847364200000044 ) ) ;
#8998=EDGE_CURVE ( 'NONE', #21862, #7753, #5742, .T. ) ;
#8999=DIRECTION ( 'NONE',  ( 1.000000000000000000, 0.000000000000000000, 0.000000000000000000 ) ) ;
#9001=CARTESIAN_POINT ( 'NONE',  ( -16.94128954410000176, -99.70025030589999915, 2.976402637920000149 ) ) ;
#9004=CARTESIAN_POINT ( 'NONE',  ( -5.736172046443546613, -98.20750306712106692, -19.47271301003372912 ) ) ;
#9006=CARTESIAN_POINT ( 'NONE',  ( -2.876553231629999985, -91.50000000000000000, -5.265495371340000119 ) ) ;
#9008=CYLINDRICAL_SURFACE ( 'NONE', #17868, 0.7500000000000003331 ) ;
#9012=CARTESIAN_POINT ( 'NONE',  ( -10.80471582220000037, -93.74976927969998997, -23.35275943390000108 ) ) ;
#9014=CARTESIAN_POINT ( 'NONE',  ( -24.08680547314210330, -92.61393927537839943, -18.71036994979779777 ) ) ;
#9016=CARTESIAN_POINT ( 'NONE',  ( 0.1125757948539710535, -92.93978723898268868, -30.49979579639168037 ) ) ;
#9023=CIRCLE ( 'NONE', #9967, 21.14285714290000229 ) ;
#9027=DIRECTION ( 'NONE',  ( 0.000000000000000000, 1.000000000000000000, 0.000000000000000000 ) ) ;
#9029=CARTESIAN_POINT ( 'NONE',  ( 6.640361864253258695, -93.59825775159440298, -26.19609744338800894 ) ) ;
#9031=CARTESIAN_POINT ( 'NONE',  ( -27.85075384980000024, -92.68283714880000446, 2.027630021949999861 ) ) ;
#9032=CARTESIAN_POINT ( 'NONE',  ( -19.98881959580000256, -95.75655295469999828, 10.31208380220000009 ) ) ;
#9040=CIRCLE ( 'NONE', #23494, 0.4999999999999988343 ) ;
#9042=CARTESIAN_POINT ( 'NONE',  ( -17.42719211919999722, -93.34960223970000470, 19.28404990989999845 ) ) ;
#9048=CARTESIAN_POINT ( 'NONE',  ( 1.014221318129999938, -99.92384627689999377, -16.88077478359999972 ) ) ;
#9058=CARTESIAN_POINT ( 'NONE',  ( 19.98296746440000149, -94.98812769030000425, 14.17693333179999904 ) ) ;
#9059=ORIENTED_EDGE ( 'NONE', *, *, #24311, .T. ) ;
#9061=CARTESIAN_POINT ( 'NONE',  ( 24.53438756210000093, -92.85282594270000800, 14.48885364650000085 ) ) ;
#9062=CARTESIAN_POINT ( 'NONE',  ( -18.34989813179999985, -111.0000000000000000, 23.56346505449999995 ) ) ;
#9067=CARTESIAN_POINT ( 'NONE',  ( -12.48345623946794269, -101.5740747342345855, -10.09958814640085478 ) ) ;
#9068=ORIENTED_EDGE ( 'NONE', *, *, #1888, .F. ) ;
#9072=CARTESIAN_POINT ( 'NONE',  ( -15.55828293390000105, -101.1889999979999999, 3.733608462140000306 ) ) ;
#9077=CARTESIAN_POINT ( 'NONE',  ( 11.85391586600000124, -101.4309749570000037, -10.98895622390000071 ) ) ;
#9079=CARTESIAN_POINT ( 'NONE',  ( -18.99420542959347458, -98.09459568842703447, -7.570339228046596425 ) ) ;
#9085=CARTESIAN_POINT ( 'NONE',  ( 15.19718069640000024, -101.1364147039999892, 2.131293228500000581 ) ) ;
#9086=CARTESIAN_POINT ( 'NONE',  ( 25.08528495285458249, -93.39299082550714104, 11.62361772614930722 ) ) ;
#9092=CYLINDRICAL_SURFACE ( 'NONE', #24402, 0.7499999999999992228 ) ;
#9097=CARTESIAN_POINT ( 'NONE',  ( 16.44163546059999703, -100.2522625769999962, 4.388208817439999798 ) ) ;
#9100=CARTESIAN_POINT ( 'NONE',  ( -19.72803626430000179, -96.95622423829999548, -6.895699102770000977 ) ) ;
#9102=CARTESIAN_POINT ( 'NONE',  ( -1.604070449259999753, -100.9197075889999979, -15.54198650660000069 ) ) ;
#9103=ORIENTED_EDGE ( 'NONE', *, *, #11114, .T. ) ;
#9105=EDGE_CURVE ( 'NONE', #20556, #2020, #6264, .T. ) ;
#9106=CARTESIAN_POINT ( 'NONE',  ( 23.96368475870000125, -93.00000000000000000, 8.717328305520000598 ) ) ;
#9114=CARTESIAN_POINT ( 'NONE',  ( -17.31257399851914869, -96.95293637055524982, 11.43669896296266586 ) ) ;
#9117=CARTESIAN_POINT ( 'NONE',  ( -3.663740619795967213, -98.56104012213324950, 19.49859454066769970 ) ) ;
#9118=CARTESIAN_POINT ( 'NONE',  ( -12.53380938399999955, -99.91102932029998840, -11.37771751150000021 ) ) ;
#9121=ORIENTED_EDGE ( 'NONE', *, *, #14883, .F. ) ;
#9122=CARTESIAN_POINT ( 'NONE',  ( 27.12516731730879371, -92.50638022835022412, -13.94618822762715027 ) ) ;
#9126=CARTESIAN_POINT ( 'NONE',  ( 14.95019707169999990, -101.2530993000000024, 2.710463435110000319 ) ) ;
#9128=CARTESIAN_POINT ( 'NONE',  ( 7.999597942409999440, -93.06863555389999476, 27.33126122210000020 ) ) ;
#9129=EDGE_LOOP ( 'NONE', ( #6200, #4743, #4247, #13492, #6941, #26920 ) ) ;
#9132=CARTESIAN_POINT ( 'NONE',  ( 20.29323830529999739, -94.22763361239999824, 13.32192879709999822 ) ) ;
#9136=CARTESIAN_POINT ( 'NONE',  ( 16.54057195470140584, -94.89197151649931072, 16.94454422099984114 ) ) ;
#9138=CARTESIAN_POINT ( 'NONE',  ( 12.39757656149999931, -101.5369810359999860, -10.11435096289999969 ) ) ;
#9139=CARTESIAN_POINT ( 'NONE',  ( -11.69298206670000084, -94.57749572790000059, -21.18607573959999968 ) ) ;
#9145=CARTESIAN_POINT ( 'NONE',  ( -11.31667057079999950, -95.23931402160000914, -21.36056405359999744 ) ) ;
#9152=CARTESIAN_POINT ( 'NONE',  ( -24.64364036189999752, -92.50000000000000000, -17.97055897050000084 ) ) ;
#9153=CARTESIAN_POINT ( 'NONE',  ( -8.209463884390000743, -99.53431386179998697, 15.35748973489999969 ) ) ;
#9155=B_SPLINE_SURFACE_WITH_KNOTS ( 'NONE', 5, 5, ( 
 ( #4864, #15920, #24826, #6613, #13440, #11543 ),
 ( #15625, #11396, #4713, #13745, #224, #521 ),
 ( #9367, #22501, #2687, #8920, #22645, #28733 ),
 ( #26725, #18269, #7201, #16067, #2393, #5000 ),
 ( #24969, #13890, #10943, #8770, #13294, #17685 ),
 ( #15473, #6764, #24525, #24382, #4423, #22198 ) ),
 .UNSPECIFIED., .F., .F., .F.,
 ( 6, 6 ),
 ( 6, 6 ),
 ( 15.82800262790000012, 19.56549066489999689 ),
 ( 0.000000000000000000, 0.5000000000000000000 ),
 .UNSPECIFIED. ) ;
#9165=CYLINDRICAL_SURFACE ( 'NONE', #9290, 0.7500000000000001110 ) ;
#9173=CARTESIAN_POINT ( 'NONE',  ( 1.338287881580000116, -94.89420189149998919, 24.43791688079999957 ) ) ;
#9174=CARTESIAN_POINT ( 'NONE',  ( -18.83859341579999835, -97.73640017439998928, 6.587273628740000220 ) ) ;
#9180=CARTESIAN_POINT ( 'NONE',  ( -13.30251043199831607, -92.87422005961661853, 27.44619162654865363 ) ) ;
#9183=CARTESIAN_POINT ( 'NONE',  ( -15.21475366910000027, -92.78573964340000657, 25.08891424309999962 ) ) ;
#9187=CARTESIAN_POINT ( 'NONE',  ( -16.97218413830000117, -98.25999569910000275, 8.877871485000001783 ) ) ;
#9188=CARTESIAN_POINT ( 'NONE',  ( -12.94585355959999973, -101.6484611540000031, -9.402386697720000797 ) ) ;
#9193=CARTESIAN_POINT ( 'NONE',  ( 6.977349081829999911, -99.61736775859999682, 15.87966916429999920 ) ) ;
#9196=ORIENTED_EDGE ( 'NONE', *, *, #10842, .T. ) ;
#9197=CARTESIAN_POINT ( 'NONE',  ( 27.96987275368786285, -92.54893169919633067, 12.16290556786634092 ) ) ;
#9199=CARTESIAN_POINT ( 'NONE',  ( 8.042002709780000202, -100.9405346150000042, 13.76814507859999814 ) ) ;
#9202=CARTESIAN_POINT ( 'NONE',  ( 9.374849370119999747, -94.98812477599999227, -22.63660903319999562 ) ) ;
#9204=CIRCLE ( 'NONE', #18063, 18.64285714289999873 ) ;
#9206=CARTESIAN_POINT ( 'NONE',  ( -7.091440874569999941, -101.0151300849999814, 13.93786069769999969 ) ) ;
#9207=DIRECTION ( 'NONE',  ( 0.000000000000000000, 1.000000000000000000, 0.000000000000000000 ) ) ;
#9210=EDGE_LOOP ( 'NONE', ( #8252, #6860, #20175, #20035, #23758, #17120, #14073, #10432, #10268, #23100, #11492, #13291, #10266, #15445, #14747, #27980, #3354, #573, #14927, #8325, #3661, #27949, #24632 ) ) ;
#9213=FACE_OUTER_BOUND ( 'NONE', #19948, .T. ) ;
#9215=CARTESIAN_POINT ( 'NONE',  ( -5.873418876839999747, -101.3150700380000018, 15.15334698740000086 ) ) ;
#9217=CARTESIAN_POINT ( 'NONE',  ( -15.42928178740000078, -101.3399685459999944, 4.712812228389999802 ) ) ;
#9219=CARTESIAN_POINT ( 'NONE',  ( -18.19446509544315660, -98.56104011354675265, -7.910728455679111093 ) ) ;
#9221=B_SPLINE_CURVE_WITH_KNOTS ( 'NONE', 3,
 ( #417, #18167, #4615, #11140, #13491, #10985 ),
 .UNSPECIFIED., .F., .F.,
 ( 4, 2, 4 ),
 ( 0.000000000000000000, 0.5000000000000000000, 1.000000000000000000 ),
 .UNSPECIFIED. ) ;
#9223=DIRECTION ( 'NONE',  ( 0.000000000000000000, 1.000000000000000000, 0.000000000000000000 ) ) ;
#9230=CARTESIAN_POINT ( 'NONE',  ( 7.797483723290000057, -101.0407491870000030, 13.41348730009999990 ) ) ;
#9231=ADVANCED_FACE ( 'NONE', ( #6563 ), #8170, .F. ) ;
#9241=ADVANCED_FACE ( 'NONE', ( #27262 ), #13544, .T. ) ;
#9242=CARTESIAN_POINT ( 'NONE',  ( 16.58138552489999995, -99.94751438429999268, 4.403722473940000270 ) ) ;
#9243=VERTEX_POINT ( 'NONE', #7300 ) ;
#9246=CARTESIAN_POINT ( 'NONE',  ( -20.03336705960000330, -97.14975611010000023, -7.249356197820000069 ) ) ;
#9248=DIRECTION ( 'NONE',  ( -0.9620897310213631926, 2.431777862510916489E-14, 0.2727331103171030668 ) ) ;
#9254=FACE_OUTER_BOUND ( 'NONE', #3687, .T. ) ;
#9255=AXIS2_PLACEMENT_3D ( 'NONE', #14287, #5261, #5676 ) ;
#9256=LINE ( 'NONE', #24863, #22994 ) ;
#9260=CARTESIAN_POINT ( 'NONE',  ( 9.895942579337763334, -99.82488179753744362, 13.91669341782708003 ) ) ;
#9261=CARTESIAN_POINT ( 'NONE',  ( 13.96412840480000028, -99.57787118740000665, -10.31025271900000106 ) ) ;
#9265=CARTESIAN_POINT ( 'NONE',  ( -13.25319097760000098, -99.78393592979999482, -11.15464849200000153 ) ) ;
#9266=CARTESIAN_POINT ( 'NONE',  ( -12.96048168789999977, -101.0356131030000029, -8.456406562079997968 ) ) ;
#9276=CARTESIAN_POINT ( 'NONE',  ( -4.592948295220000254, -99.60591459110000301, 16.75688848409999920 ) ) ;
#9277=CARTESIAN_POINT ( 'NONE',  ( 4.027230326479999789, -93.61421867219999626, 26.02828154170000019 ) ) ;
#9279=ORIENTED_EDGE ( 'NONE', *, *, #21910, .F. ) ;
#9284=FACE_OUTER_BOUND ( 'NONE', #14019, .T. ) ;
#9287=CARTESIAN_POINT ( 'NONE',  ( -11.80897031970000022, -94.89419905519999077, -21.43712780819999963 ) ) ;
#9288=LINE ( 'NONE', #24900, #9655 ) ;
#9289=VERTEX_POINT ( 'NONE', #2646 ) ;
#9290=AXIS2_PLACEMENT_3D ( 'NONE', #2788, #13701, #26672 ) ;
#9293=CARTESIAN_POINT ( 'NONE',  ( 13.81202799179999907, -99.83167681540000160, -10.46592613740000210 ) ) ;
#9296=EDGE_CURVE ( 'NONE', #21931, #11437, #17924, .T. ) ;
#9298=DIRECTION ( 'NONE',  ( 1.000000000000000000, 0.000000000000000000, 0.000000000000000000 ) ) ;
#9299=LINE ( 'NONE', #24610, #5323 ) ;
#9302=CARTESIAN_POINT ( 'NONE',  ( -13.16777714140000022, -93.19477243160000057, -23.58326759370000048 ) ) ;
#9304=CARTESIAN_POINT ( 'NONE',  ( 16.47431367404465519, -100.3266728692175604, 4.354304509586214067 ) ) ;
#9313=CARTESIAN_POINT ( 'NONE',  ( 2.936125748261882329, -94.27892262462431461, 25.39667714426032674 ) ) ;
#9315=VERTEX_POINT ( 'NONE', #11352 ) ;
#9316=DIRECTION ( 'NONE',  ( 1.000000000000000000, 0.000000000000000000, 0.000000000000000000 ) ) ;
#9319=FACE_OUTER_BOUND ( 'NONE', #3940, .T. ) ;
#9322=CARTESIAN_POINT ( 'NONE',  ( 3.287760219085154034, -93.08694455155865910, -28.89923981485827653 ) ) ;
#9324=CARTESIAN_POINT ( 'NONE',  ( -19.51835485619999844, -96.93405158080001627, 8.497257209180000714 ) ) ;
#9332=ORIENTED_EDGE ( 'NONE', *, *, #27264, .T. ) ;
#9333=AXIS2_PLACEMENT_3D ( 'NONE', #1362, #5582, #18986 ) ;
#9339=ADVANCED_FACE ( 'NONE', ( #9319 ), #9165, .T. ) ;
#9349=CARTESIAN_POINT ( 'NONE',  ( 29.70835240799999966, -111.0000000000000000, 6.903897247299999762 ) ) ;
#9353=CARTESIAN_POINT ( 'NONE',  ( 12.56967481719999924, -98.60488738940000530, 15.21211751169999893 ) ) ;
#9355=AXIS2_PLACEMENT_3D ( 'NONE', #1932, #6283, #12685 ) ;
#9357=CARTESIAN_POINT ( 'NONE',  ( 26.40928907389999836, -92.68584525839999344, 13.21124990449999892 ) ) ;
#9358=VECTOR ( 'NONE', #16541, 1000.000000000000000 ) ;
#9361=CARTESIAN_POINT ( 'NONE',  ( -7.177518981630000461, -101.0875971110000080, 13.63542055629999972 ) ) ;
#9365=CARTESIAN_POINT ( 'NONE',  ( 7.635702898730000854, -101.6454117330000031, 14.06304778130000166 ) ) ;
#9367=CARTESIAN_POINT ( 'NONE',  ( 8.044160629040000288, -99.43227399260000254, 16.10826361970000065 ) ) ;
#9370=CARTESIAN_POINT ( 'NONE',  ( -0.8840378704480000849, -98.93445099689999722, -18.66589242400000259 ) ) ;
#9372=FACE_OUTER_BOUND ( 'NONE', #13853, .T. ) ;
#9376=DIRECTION ( 'NONE',  ( 1.000000000000000000, 0.000000000000000000, 0.000000000000000000 ) ) ;
#9378=CARTESIAN_POINT ( 'NONE',  ( 24.52645331487275016, -93.02765837720220077, -16.48025453447625210 ) ) ;
#9379=CARTESIAN_POINT ( 'NONE',  ( -14.98639447530000091, -101.1747052350000047, 3.063292548799999793 ) ) ;
#9386=CARTESIAN_POINT ( 'NONE',  ( 7.853421650889998773, -101.2316184180000107, 13.89973574110000065 ) ) ;
#9387=CARTESIAN_POINT ( 'NONE',  ( 22.60879084260000127, -95.55433883439999931, -0.3969473061980000050 ) ) ;
#9390=CARTESIAN_POINT ( 'NONE',  ( 20.29323830529999739, -94.22763361239999824, 13.32192879709999822 ) ) ;
#9392=DIRECTION ( 'NONE',  ( 1.000000000000000000, 0.000000000000000000, 0.000000000000000000 ) ) ;
#9395=CARTESIAN_POINT ( 'NONE',  ( -24.12300435170000057, -94.89420189139998740, -4.133213877870000275 ) ) ;
#9398=CARTESIAN_POINT ( 'NONE',  ( 9.117424198366714805, -92.82044061133264279, 29.10537173539315603 ) ) ;
#9402=DIRECTION ( 'NONE',  ( 0.05900121837168146449, 0.000000000000000000, 0.9982579106777251798 ) ) ;
#9406=CARTESIAN_POINT ( 'NONE',  ( -17.57653423721919950, -95.76346916417317345, 13.69972344651582397 ) ) ;
#9407=B_SPLINE_SURFACE_WITH_KNOTS ( 'NONE', 5, 5, ( 
 ( #24686, #13894, #4568, #24830, #13750, #4718, #22650, #22353, #18275 ),
 ( #9077, #7352, #22797, #17980, #6912, #2838, #11697, #2691, #78 ),
 ( #11548, #18422, #670, #24389, #4428, #13299, #22203, #2248, #17834 ),
 ( #26732, #23508, #16215, #2989, #7916, #21046, #7652, #16801, #27460 ),
 ( #1105, #16520, #3273, #5308, #21183, #25694, #3134, #19127, #5720 ),
 ( #7509, #3545, #14603, #16370, #20761, #5585, #25281, #1366, #23091 ) ),
 .UNSPECIFIED., .F., .F., .F.,
 ( 6, 6 ),
 ( 6, 3, 6 ),
 ( 4.816191416729999730, 6.255250589880000156 ),
 ( 0.000000000000000000, 0.2500000000000000000, 0.5000000000000000000 ),
 .UNSPECIFIED. ) ;
#9411=CARTESIAN_POINT ( 'NONE',  ( 8.093994091077075126, -101.4116343943851177, 14.00832529574788943 ) ) ;
#9412=CARTESIAN_POINT ( 'NONE',  ( -13.15133833870000046, -100.9197081840000010, -8.436152112259998503 ) ) ;
#9413=CARTESIAN_POINT ( 'NONE',  ( 15.98190517250000120, -101.1461874320000049, 2.387865266659999985 ) ) ;
#9415=ADVANCED_FACE ( 'NONE', ( #25783 ), #5247, .T. ) ;
#9416=CARTESIAN_POINT ( 'NONE',  ( 26.94419639614420348, -92.55017404142731152, -14.29196685862621941 ) ) ;
#9423=CARTESIAN_POINT ( 'NONE',  ( 2.608016585090000117, -93.87272511149998877, 25.04074494509999838 ) ) ;
#9427=CARTESIAN_POINT ( 'NONE',  ( 27.25648091989999955, -92.50000000000000000, -13.26500883389999963 ) ) ;
#9439=EDGE_CURVE ( 'NONE', #3543, #23834, #20343, .T. ) ;
#9440=CARTESIAN_POINT ( 'NONE',  ( -16.98428476389999631, -99.78393587620000460, 3.406952114930000164 ) ) ;
#9443=EDGE_LOOP ( 'NONE', ( #17794, #5979 ) ) ;
#9444=CARTESIAN_POINT ( 'NONE',  ( 0.000000000000000000, -92.50000000000000000, 0.000000000000000000 ) ) ;
#9447=EDGE_LOOP ( 'NONE', ( #7155, #24333, #8609, #20413 ) ) ;
#9449=CARTESIAN_POINT ( 'NONE',  ( -8.456190936129999614, -94.17494422240000063, -22.86729140410000127 ) ) ;
#9451=CARTESIAN_POINT ( 'NONE',  ( -19.16019836899999618, -92.50000000000000000, 22.97842938279999814 ) ) ;
#9453=CARTESIAN_POINT ( 'NONE',  ( 15.98584715875140816, -100.9609609849234317, 4.228316488232548132 ) ) ;
#9457=DIRECTION ( 'NONE',  ( 0.9551367254897007442, 0.000000000000000000, -0.2961652167639068911 ) ) ;
#9463=CARTESIAN_POINT ( 'NONE',  ( 9.406883472537318269, -93.09720821804000934, 27.44372935570929428 ) ) ;
#9464=ORIENTED_EDGE ( 'NONE', *, *, #1151, .T. ) ;
#9465=ADVANCED_FACE ( 'NONE', ( #26052 ), #6231, .T. ) ;
#9476=CARTESIAN_POINT ( 'NONE',  ( 22.95301390182565981, -94.52293547160145692, -6.773259248599760696 ) ) ;
#9479=VERTEX_POINT ( 'NONE', #13320 ) ;
#9480=DIRECTION ( 'NONE',  ( -0.000000000000000000, 1.000000000000000000, 0.000000000000000000 ) ) ;
#9488=CARTESIAN_POINT ( 'NONE',  ( 0.000000000000000000, -92.50000000000000000, 29.91857981989999971 ) ) ;
#9490=CARTESIAN_POINT ( 'NONE',  ( -18.48852190589999722, -96.16769445330000110, 13.76947523039999943 ) ) ;
#9493=LINE ( 'NONE', #7481, #10477 ) ;
#9504=VERTEX_POINT ( 'NONE', #25775 ) ;
#9505=AXIS2_PLACEMENT_3D ( 'NONE', #749, #26807, #22726 ) ;
#9511=CARTESIAN_POINT ( 'NONE',  ( -12.16062739216652844, -93.49518251413884684, -23.50287856905526596 ) ) ;
#9518=CARTESIAN_POINT ( 'NONE',  ( -0.6277499419469999564, -98.58303758080000989, -18.67917185369999800 ) ) ;
#9519=ORIENTED_EDGE ( 'NONE', *, *, #20842, .T. ) ;
#9524=CARTESIAN_POINT ( 'NONE',  ( 15.55721680684482422, -95.01009333053707451, 17.28868226685500531 ) ) ;
#9529=DIRECTION ( 'NONE',  ( 0.000000000000000000, -1.000000000000000000, 0.000000000000000000 ) ) ;
#9531=CARTESIAN_POINT ( 'NONE',  ( 6.938098718590000047, -101.3138676899999950, 14.32202409469999971 ) ) ;
#9532=CARTESIAN_POINT ( 'NONE',  ( 13.87366454287167272, -97.42330309954748202, -15.20396809591327880 ) ) ;
#9533=AXIS2_PLACEMENT_3D ( 'NONE', #7767, #4986, #4852 ) ;
#9534=CARTESIAN_POINT ( 'NONE',  ( 8.137534397419999621, -101.2306315539999986, 14.02341335179999859 ) ) ;
#9535=CARTESIAN_POINT ( 'NONE',  ( 23.56065677060000496, -94.89196973819998959, -2.367188657780000316 ) ) ;
#9539=CARTESIAN_POINT ( 'NONE',  ( 28.24241828440000290, -92.51331410669999400, 7.994460720630000239 ) ) ;
#9542=CARTESIAN_POINT ( 'NONE',  ( -20.49585304202401304, -93.08996811592636789, -20.60571651767068602 ) ) ;
#9543=EDGE_CURVE ( 'NONE', #9289, #17308, #25569, .T. ) ;
#9545=CARTESIAN_POINT ( 'NONE',  ( 16.36531008860000114, -100.1459902240000019, 4.432835649019999380 ) ) ;
#9548=CARTESIAN_POINT ( 'NONE',  ( -15.65528393829999843, -99.91547912590000635, -8.850932903340000379 ) ) ;
#9549=VERTEX_POINT ( 'NONE', #8486 ) ;
#9550=EDGE_CURVE ( 'NONE', #2397, #20007, #4266, .T. ) ;
#9551=CARTESIAN_POINT ( 'NONE',  ( -30.47727153658393817, -92.54893169919638751, 1.177273713142487299 ) ) ;
#9553=ORIENTED_EDGE ( 'NONE', *, *, #4752, .F. ) ;
#9562=ORIENTED_EDGE ( 'NONE', *, *, #16252, .T. ) ;
#9567=CARTESIAN_POINT ( 'NONE',  ( 15.38949396259999958, -100.9938510739999913, 2.079911269780000183 ) ) ;
#9572=CARTESIAN_POINT ( 'NONE',  ( -3.818589290579999851, -98.24904979169998853, 18.91383438800000150 ) ) ;
#9573=CARTESIAN_POINT ( 'NONE',  ( 1.375221473979999942, -94.98812079580000045, 24.46248441310000032 ) ) ;
#9574=ORIENTED_EDGE ( 'NONE', *, *, #22180, .T. ) ;
#9576=CARTESIAN_POINT ( 'NONE',  ( -27.66915836665225115, -93.38554229045760735, 0.4566536595772645590 ) ) ;
#9580=AXIS2_PLACEMENT_3D ( 'NONE', #4540, #15747, #2368 ) ;
#9589=CARTESIAN_POINT ( 'NONE',  ( -15.69013080879999933, -101.5700432450000079, 3.430602099230000146 ) ) ;
#9594=CARTESIAN_POINT ( 'NONE',  ( 1.100347978140000071, -100.4792519539999915, -16.15648718290000119 ) ) ;
#9597=CARTESIAN_POINT ( 'NONE',  ( -11.95735878380000017, -93.37862425630000018, -23.50938391520000081 ) ) ;
#9600=CARTESIAN_POINT ( 'NONE',  ( 16.01243526655122196, -100.9229461893936701, 4.244774380830527605 ) ) ;
#9601=CARTESIAN_POINT ( 'NONE',  ( 19.60651740941162657, -94.52293547161876575, 13.72233081940722599 ) ) ;
#9612=ORIENTED_EDGE ( 'NONE', *, *, #6763, .T. ) ;
#9614=CARTESIAN_POINT ( 'NONE',  ( -6.005235968310000061, -101.3350617309999961, 14.85412936009999996 ) ) ;
#9630=CARTESIAN_POINT ( 'NONE',  ( -17.79736829950000043, -96.96042919349999067, 11.10778547589999832 ) ) ;
#9640=CIRCLE ( 'NONE', #17087, 0.7999999999999986011 ) ;
#9642=CARTESIAN_POINT ( 'NONE',  ( 17.29688842079999844, -95.76597000319999609, 14.77140804379999928 ) ) ;
#9646=EDGE_CURVE ( 'NONE', #22453, #2955, #19969, .T. ) ;
#9649=CARTESIAN_POINT ( 'NONE',  ( -7.936795339069999677, -100.2522625769999962, 15.05294100799999946 ) ) ;
#9651=CARTESIAN_POINT ( 'NONE',  ( -10.29133506492763495, -93.94301621637545452, -23.20339123508392376 ) ) ;
#9653=CARTESIAN_POINT ( 'NONE',  ( 7.302962794079999931, -101.1832940899999898, 13.42647164559999950 ) ) ;
#9655=VECTOR ( 'NONE', #24309, 1000.000000000000000 ) ;
#9657=CARTESIAN_POINT ( 'NONE',  ( -29.47186164440000056, -93.00000450890000536, -0.4149713922389999810 ) ) ;
#9658=CARTESIAN_POINT ( 'NONE',  ( 11.83897591930000104, -98.30614355250000358, -15.44231161390000118 ) ) ;
#9663=CARTESIAN_POINT ( 'NONE',  ( -17.59792109239500846, -92.65976904079671783, 24.91111247217822466 ) ) ;
#9671=CARTESIAN_POINT ( 'NONE',  ( 13.87165893064168820, -97.41291607268185260, -15.22385153909266187 ) ) ;
#9676=CARTESIAN_POINT ( 'NONE',  ( 21.75609418980000243, -93.65024019829999702, 12.77708436150000004 ) ) ;
#9678=CARTESIAN_POINT ( 'NONE',  ( 0.3164238574520000236, -92.54628605920001405, -30.13191910649999983 ) ) ;
#9679=DIRECTION ( 'NONE',  ( -0.9863585068926601362, 0.000000000000000000, -0.1646113479699435334 ) ) ;
#9684=CARTESIAN_POINT ( 'NONE',  ( -13.15133943750000078, -100.9197081840000010, -8.436149941960000120 ) ) ;
#9686=CARTESIAN_POINT ( 'NONE',  ( -30.41749109087852077, -92.77481473396083800, 2.243079458206835408 ) ) ;
#9688=CARTESIAN_POINT ( 'NONE',  ( 0.09569509352523042356, -101.5829753080977582, -16.05020235182843891 ) ) ;
#9691=CARTESIAN_POINT ( 'NONE',  ( -11.72126804459999860, -100.9137139110000021, -10.34406313869999927 ) ) ;
#9693=AXIS2_PLACEMENT_3D ( 'NONE', #25049, #27682, #24907 ) ;
#9694=CARTESIAN_POINT ( 'NONE',  ( 13.53498567739999991, -95.75647260690000451, -17.96385118539999937 ) ) ;
#9695=EDGE_LOOP ( 'NONE', ( #21551, #653, #9553, #12452 ) ) ;
#9701=CARTESIAN_POINT ( 'NONE',  ( 15.75037718549999965, -101.2459394079999981, 2.542735002740000194 ) ) ;
#9704=ORIENTED_EDGE ( 'NONE', *, *, #12711, .F. ) ;
#9708=CARTESIAN_POINT ( 'NONE',  ( -2.609756160320000351, -97.14975611439999170, 21.14422222710000199 ) ) ;
#9709=CARTESIAN_POINT ( 'NONE',  ( 12.02192718879999944, -92.50000321470000131, 27.08489650960000006 ) ) ;
#9726=CARTESIAN_POINT ( 'NONE',  ( -15.27515611620000158, -100.9817027879999927, 2.888957402029999511 ) ) ;
#9730=AXIS2_PLACEMENT_3D ( 'NONE', #20304, #24831, #6771 ) ;
#9736=EDGE_CURVE ( 'NONE', #13319, #5829, #10676, .T. ) ;
#9738=DIRECTION ( 'NONE',  ( 0.000000000000000000, 1.000000000000000000, 0.000000000000000000 ) ) ;
#9741=DIRECTION ( 'NONE',  ( 0.000000000000000000, -1.000000000000000000, 0.000000000000000000 ) ) ;
#9742=CARTESIAN_POINT ( 'NONE',  ( 13.91346788694689529, -99.62767017963102489, -10.34347588715546351 ) ) ;
#9749=CARTESIAN_POINT ( 'NONE',  ( 8.318977493526379163, -93.18009965537066819, 27.27745815282288433 ) ) ;
#9750=EDGE_LOOP ( 'NONE', ( #28518, #14300, #25943, #620 ) ) ;
#9751=CARTESIAN_POINT ( 'NONE',  ( 22.78266135780000212, -94.59276583640000524, -6.873198607739999133 ) ) ;
#9754=CARTESIAN_POINT ( 'NONE',  ( -6.166870861799999659, -101.6484611580000035, 14.76436469649999950 ) ) ;
#9757=AXIS2_PLACEMENT_3D ( 'NONE', #21503, #1561, #5770 ) ;
#9758=CIRCLE ( 'NONE', #17194, 20.64285714289999873 ) ;
#9766=CARTESIAN_POINT ( 'NONE',  ( 19.86697918760000192, -97.58045781670000451, 2.400950920309999681 ) ) ;
#9768=VERTEX_POINT ( 'NONE', #27155 ) ;
#9769=EDGE_CURVE ( 'NONE', #1054, #17152, #10261, .T. ) ;
#9770=CARTESIAN_POINT ( 'NONE',  ( 29.70835240799999966, -93.00000000000000000, 6.903897247299999762 ) ) ;
#9775=CARTESIAN_POINT ( 'NONE',  ( -16.70219504179999959, -100.0012196380000091, 6.767083061890000195 ) ) ;
#9780=CIRCLE ( 'NONE', #11211, 29.91857981989999971 ) ;
#9786=ORIENTED_EDGE ( 'NONE', *, *, #18095, .F. ) ;
#9794=DIRECTION ( 'NONE',  ( 1.000000000000000000, 0.000000000000000000, 0.000000000000000000 ) ) ;
#9797=CARTESIAN_POINT ( 'NONE',  ( -13.83118819819999956, -92.50000000000000000, 21.42307711379999802 ) ) ;
#9800=CARTESIAN_POINT ( 'NONE',  ( -28.43155917910000241, -92.70565333729999224, -2.447589390230000106 ) ) ;
#9813=CARTESIAN_POINT ( 'NONE',  ( 12.02710806035337399, -99.07183863203711383, 14.93578453548695961 ) ) ;
#9814=CARTESIAN_POINT ( 'NONE',  ( -16.54756449519999961, -100.0429506999999916, 2.640690120740000424 ) ) ;
#9815=ORIENTED_EDGE ( 'NONE', *, *, #6688, .F. ) ;
#9819=B_SPLINE_CURVE_WITH_KNOTS ( 'NONE', 5,
 ( #13506, #15545, #4485, #22417, #9136, #13358 ),
 .UNSPECIFIED., .F., .F.,
 ( 6, 6 ),
 ( 0.000000000000000000, 1.000000000000000000 ),
 .UNSPECIFIED. ) ;
#9821=AXIS2_PLACEMENT_3D ( 'NONE', #4390, #1645, #28276 ) ;
#9822=CARTESIAN_POINT ( 'NONE',  ( -11.71096632150000083, -94.52293512109999085, -20.87034205579999835 ) ) ;
#9826=CARTESIAN_POINT ( 'NONE',  ( -7.322964735850000295, -98.83667233820000320, 17.15365167710000094 ) ) ;
#9827=CARTESIAN_POINT ( 'NONE',  ( -21.52470944380124962, -93.02765837720517084, -20.24432229263281968 ) ) ;
#9830=CARTESIAN_POINT ( 'NONE',  ( -5.893951993130000346E-12, -111.0000000000000000, -1.129762949859999995E-12 ) ) ;
#9832=CARTESIAN_POINT ( 'NONE',  ( -5.598527377420000839, -101.2141467319999890, 14.18131542549999935 ) ) ;
#9836=CARTESIAN_POINT ( 'NONE',  ( 0.5154897680143201155, -100.1406256087915807, -17.18202921360721547 ) ) ;
#9838=CARTESIAN_POINT ( 'NONE',  ( -12.27960098470000005, -100.1275643909999928, -11.24051300700000056 ) ) ;
#9839=CARTESIAN_POINT ( 'NONE',  ( -14.12701123409999937, -93.90388142519999803, -21.62231189339999915 ) ) ;
#9840=AXIS2_PLACEMENT_3D ( 'NONE', #10489, #10355, #8316 ) ;
#9846=CARTESIAN_POINT ( 'NONE',  ( 23.89360401162774039, -92.87422005962199023, -18.95642123213606212 ) ) ;
#9853=ORIENTED_EDGE ( 'NONE', *, *, #11624, .F. ) ;
#9856=CARTESIAN_POINT ( 'NONE',  ( -4.028625675479999835, -98.69238697990000730, 19.35340251219999885 ) ) ;
#9865=DIRECTION ( 'NONE',  ( -0.9890497259025925469, 0.000000000000000000, -0.1475826537639393088 ) ) ;
#9866=CARTESIAN_POINT ( 'NONE',  ( 7.571687472095536720, -101.4628082770392297, 14.06488328537873045 ) ) ;
#9868=EDGE_CURVE ( 'NONE', #22409, #5288, #11639, .T. ) ;
#9870=ORIENTED_EDGE ( 'NONE', *, *, #4281, .F. ) ;
#9872=CARTESIAN_POINT ( 'NONE',  ( -16.08960165530000097, -101.0043489809999926, 3.145915650070000069 ) ) ;
#9874=CARTESIAN_POINT ( 'NONE',  ( -6.285925807512719565, -101.5555610555536248, 14.71350185178380343 ) ) ;
#9879=CARTESIAN_POINT ( 'NONE',  ( -7.919799262655152994, -100.2392017796619683, 15.16708595175554741 ) ) ;
#9882=CARTESIAN_POINT ( 'NONE',  ( 15.98858835731819994, -100.9570234913455664, 4.230075987765046897 ) ) ;
#9893=B_SPLINE_CURVE_WITH_KNOTS ( 'NONE', 3,
 ( #683, #27323, #7364, #8476, #8067, #17520, #17378, #26271, #6436, #17231, #17086, #10228, #1663, #14885, #21892, #8618, #3693, #14749, #19139 ),
 .UNSPECIFIED., .F., .F.,
 ( 4, 2, 2, 2, 1, 1, 1, 1, 1, 2, 2, 4 ),
 ( 0.000000000000000000, 0.2500000000000162648, 0.3750000000000244804, 0.4375000000000285882, 0.4687500000000299760, 0.4843750000000301981, 0.4921875000000297540, 0.4960937500000293654, 0.4980468750000286993, 0.4990234375000283662, 0.5000000000000279776, 1.000000000000000000 ),
 .UNSPECIFIED. ) ;
#9896=CIRCLE ( 'NONE', #4791, 15.19391340349999986 ) ;
#9898=EDGE_CURVE ( 'NONE', #27709, #19799, #14031, .T. ) ;
#9901=CARTESIAN_POINT ( 'NONE',  ( -20.43932202180000246, -94.59276292389999696, 12.18704577789999988 ) ) ;
#9902=CARTESIAN_POINT ( 'NONE',  ( -15.50938051129999984, -101.3150705480000084, 4.855933523060000034 ) ) ;
#9905=CARTESIAN_POINT ( 'NONE',  ( 8.188637977920000921, -100.9197082849999987, 13.30686163390000054 ) ) ;
#9906=ORIENTED_EDGE ( 'NONE', *, *, #1851, .T. ) ;
#9911=CARTESIAN_POINT ( 'NONE',  ( 23.99827830379999583, -92.84292833370000153, -18.61030780140000118 ) ) ;
#9912=ORIENTED_EDGE ( 'NONE', *, *, #17642, .T. ) ;
#9914=CARTESIAN_POINT ( 'NONE',  ( 7.584268328590000330, -101.6484612600000048, 14.08825304710000026 ) ) ;
#9921=AXIS2_PLACEMENT_3D ( 'NONE', #17647, #6569, #11043 ) ;
#9924=CARTESIAN_POINT ( 'NONE',  ( 0.000000000000000000, -111.0000000000000000, 0.000000000000000000 ) ) ;
#9928=ORIENTED_EDGE ( 'NONE', *, *, #8436, .F. ) ;
#9929=CARTESIAN_POINT ( 'NONE',  ( 27.23269985219999967, -92.50000000000000000, -12.38957130830000075 ) ) ;
#9932=CARTESIAN_POINT ( 'NONE',  ( -8.001416342079998856, -100.4792519539999915, 14.07906887139999874 ) ) ;
#9933=CARTESIAN_POINT ( 'NONE',  ( 6.103564891039999551, -92.56168957700000988, 29.00427579219999785 ) ) ;
#9936=EDGE_LOOP ( 'NONE', ( #7903, #19206, #14221, #14510 ) ) ;
#9938=DIRECTION ( 'NONE',  ( 0.000000000000000000, 1.000000000000000000, 0.000000000000000000 ) ) ;
#9944=CARTESIAN_POINT ( 'NONE',  ( -16.54318588419999969, -111.0000000000000000, 25.62368046950000178 ) ) ;
#9946=CARTESIAN_POINT ( 'NONE',  ( -17.56187199568302759, -92.66972459457754496, 24.93653312871382255 ) ) ;
#9947=AXIS2_PLACEMENT_3D ( 'NONE', #8573, #17477, #2040 ) ;
#9951=CARTESIAN_POINT ( 'NONE',  ( 13.86409537477300624, -98.07566823408926382, 15.06275398214450156 ) ) ;
#9957=CARTESIAN_POINT ( 'NONE',  ( -11.44873198189999819, -94.64875831279999829, -20.83031290489999776 ) ) ;
#9960=ADVANCED_FACE ( 'NONE', ( #7905 ), #11736, .F. ) ;
#9965=DIRECTION ( 'NONE',  ( 1.000000000000000000, 0.000000000000000000, 0.000000000000000000 ) ) ;
#9967=AXIS2_PLACEMENT_3D ( 'NONE', #18978, #3946, #21581 ) ;
#9969=CARTESIAN_POINT ( 'NONE',  ( 0.000000000000000000, -111.0000000000000000, 0.000000000000000000 ) ) ;
#9970=ORIENTED_EDGE ( 'NONE', *, *, #6313, .F. ) ;
#9973=CARTESIAN_POINT ( 'NONE',  ( 0.3020942853670610106, -101.4304678898396332, -16.16567993605933395 ) ) ;
#9975=CARTESIAN_POINT ( 'NONE',  ( 13.34729337145036965, -92.71619979444699311, 27.42443759431768058 ) ) ;
#9976=CARTESIAN_POINT ( 'NONE',  ( -13.38017493169999916, -94.34469964500000572, -21.61746068469999926 ) ) ;
#9977=( GEOMETRIC_REPRESENTATION_CONTEXT ( 3 ) GLOBAL_UNCERTAINTY_ASSIGNED_CONTEXT ( ( #7731 ) ) GLOBAL_UNIT_ASSIGNED_CONTEXT ( ( #6474, #25872, #1974 ) ) REPRESENTATION_CONTEXT ( 'NONE', 'WORKASPACE' ) );
#9980=CARTESIAN_POINT ( 'NONE',  ( -18.26810397560000254, -94.98812477769999418, 16.32728546869999775 ) ) ;
#9982=CARTESIAN_POINT ( 'NONE',  ( -14.73065703798407711, -101.1848546039999945, 4.068069545059747050 ) ) ;
#9991=CARTESIAN_POINT ( 'NONE',  ( -28.68689398529999934, -92.57423544259999915, 3.199804733899999754 ) ) ;
#9992=CARTESIAN_POINT ( 'NONE',  ( 1.776356839399999804E-15, -101.6484611540000031, -1.776356839399999804E-15 ) ) ;
#9994=CARTESIAN_POINT ( 'NONE',  ( -0.08129961819659545230, -95.57586223754451282, 22.58573869906598830 ) ) ;
#9998=CARTESIAN_POINT ( 'NONE',  ( 9.374849361280000792, -94.98812477599999227, -22.63660904189999812 ) ) ;
#10001=B_SPLINE_CURVE_WITH_KNOTS ( 'NONE', 3,
 ( #5659, #23448, #9742, #22881, #27394, #27547 ),
 .UNSPECIFIED., .F., .F.,
 ( 4, 2, 4 ),
 ( 0.000000000000000000, 0.5000000000000000000, 1.000000000000000000 ),
 .UNSPECIFIED. ) ;
#10002=CARTESIAN_POINT ( 'NONE',  ( 26.21017338629999927, -93.14733690340000294, -7.956146379909999844 ) ) ;
#10004=VERTEX_POINT ( 'NONE', #26242 ) ;
#10006=CARTESIAN_POINT ( 'NONE',  ( -15.63746481129999921, -100.7880644439999998, 2.916848959350000214 ) ) ;
#10015=AXIS2_PLACEMENT_3D ( 'NONE', #2476, #22136, #4798 ) ;
#10022=CARTESIAN_POINT ( 'NONE',  ( 6.748482936971252677, -100.5798851012459210, 15.42610337842955026 ) ) ;
#10026=ORIENTED_EDGE ( 'NONE', *, *, #6811, .F. ) ;
#10028=CARTESIAN_POINT ( 'NONE',  ( -6.285925807579999969, -101.6484611540000031, 14.71350185179999848 ) ) ;
#10030=CARTESIAN_POINT ( 'NONE',  ( -6.124560390765033446, -95.75133629536016144, -21.89659062549250734 ) ) ;
#10033=CARTESIAN_POINT ( 'NONE',  ( -12.97641886767416430, -101.6484611540000031, -9.360302276478243755 ) ) ;
#10038=CARTESIAN_POINT ( 'NONE',  ( 16.76737182020000105, -99.57787118749999422, 4.489257787179999681 ) ) ;
#10039=CARTESIAN_POINT ( 'NONE',  ( 16.22917866779999940, -99.91102932019998661, 4.812753184709999132 ) ) ;
#10043=CARTESIAN_POINT ( 'NONE',  ( -12.94585355959999973, -101.6484611540000031, -9.402386697720000797 ) ) ;
#10045=DIRECTION ( 'NONE',  ( 0.000000000000000000, -1.000000000000000000, 0.000000000000000000 ) ) ;
#10047=CARTESIAN_POINT ( 'NONE',  ( 23.17124894566643434, -95.36087493982624608, -1.748483809854802118 ) ) ;
#10049=EDGE_CURVE ( 'NONE', #25778, #27814, #520, .T. ) ;
#10063=CARTESIAN_POINT ( 'NONE',  ( -12.92849772029999933, -101.3256027080000052, -9.267492799690000282 ) ) ;
#10064=CARTESIAN_POINT ( 'NONE',  ( 23.92053897610000135, -91.50000000000000000, -18.92241567810000191 ) ) ;
#10065=CARTESIAN_POINT ( 'NONE',  ( -1.869204707399999776, -93.63284696360000225, 25.01358039600000183 ) ) ;
#10066=DIRECTION ( 'NONE',  ( 0.000000000000000000, -1.000000000000000000, 0.000000000000000000 ) ) ;
#10067=CARTESIAN_POINT ( 'NONE',  ( 7.243954325790000759, -101.1848542809999856, 13.45609835219999972 ) ) ;
#10073=DIRECTION ( 'NONE',  ( 0.000000000000000000, 1.000000000000000000, 0.000000000000000000 ) ) ;
#10080=CARTESIAN_POINT ( 'NONE',  ( -0.1776101844839999833, -101.4254868729999970, -15.96796905659999766 ) ) ;
#10081=CARTESIAN_POINT ( 'NONE',  ( 12.72804228091459144, -98.68740076101950365, 15.00358873733218168 ) ) ;
#10085=CARTESIAN_POINT ( 'NONE',  ( 6.638238976540000280, -100.0496341300000154, 15.55554575080000035 ) ) ;
#10086=CARTESIAN_POINT ( 'NONE',  ( 13.56781805022574439, -96.36359511437918002, -17.24825640581852326 ) ) ;
#10087=CARTESIAN_POINT ( 'NONE',  ( 7.642202223189999977, -101.1334489860000048, 13.31223315789999972 ) ) ;
#10092=CARTESIAN_POINT ( 'NONE',  ( 25.91186513281249404, -93.33134965530122429, -7.488690889712852794 ) ) ;
#10094=CIRCLE ( 'NONE', #7344, 23.79684788999999867 ) ;
#10095=ORIENTED_EDGE ( 'NONE', *, *, #4173, .F. ) ;
#10101=VERTEX_POINT ( 'NONE', #22007 ) ;
#10108=CARTESIAN_POINT ( 'NONE',  ( 11.77817022719999862, -101.0685849509999912, -10.96540529560000010 ) ) ;
#10110=DIRECTION ( 'NONE',  ( 0.9919319056295825554, 0.000000000000000000, 0.1267718209779474525 ) ) ;
#10117=CIRCLE ( 'NONE', #18965, 18.14285714289999873 ) ;
#10123=CARTESIAN_POINT ( 'NONE',  ( -29.43810879609999986, -92.99999932709999939, 4.713437748839999664 ) ) ;
#10124=CARTESIAN_POINT ( 'NONE',  ( 9.108768439514689064, -94.52419745025660802, -22.22443064656424383 ) ) ;
#10130=CIRCLE ( 'NONE', #9693, 23.79684788999999867 ) ;
#10136=CARTESIAN_POINT ( 'NONE',  ( -15.12545007849999834, -101.1042191290000005, 4.523950879969999228 ) ) ;
#10137=CARTESIAN_POINT ( 'NONE',  ( -15.12490670039999863, -101.0835132970000103, 3.210671277119999889 ) ) ;
#10143=CARTESIAN_POINT ( 'NONE',  ( -7.367195939092531454, -101.3586211803017960, 14.45516488556769907 ) ) ;
#10145=EDGE_CURVE ( 'NONE', #6448, #7597, #13247, .T. ) ;
#10154=CARTESIAN_POINT ( 'NONE',  ( 6.682768326704020545, -100.8061861241085353, 15.25838507520291287 ) ) ;
#10160=CARTESIAN_POINT ( 'NONE',  ( -6.003869784890000005, -101.1848541609999899, 14.05329173640000029 ) ) ;
#10161=ORIENTED_EDGE ( 'NONE', *, *, #3341, .T. ) ;
#10162=CARTESIAN_POINT ( 'NONE',  ( 13.69115815750000031, -100.1275643909999928, -9.470476298019999462 ) ) ;
#10170=VERTEX_POINT ( 'NONE', #20554 ) ;
#10174=CARTESIAN_POINT ( 'NONE',  ( 11.67094368468833387, -93.01584921746606938, -23.70866539702249653 ) ) ;
#10175=CARTESIAN_POINT ( 'NONE',  ( 24.17687301000000133, -92.98481302140000082, -11.27069079640000027 ) ) ;
#10178=CARTESIAN_POINT ( 'NONE',  ( 29.73294340391298007, -92.80442066025455006, 6.797243626917193637 ) ) ;
#10180=ORIENTED_EDGE ( 'NONE', *, *, #7540, .T. ) ;
#10181=CARTESIAN_POINT ( 'NONE',  ( 9.718892398710000435, -91.50000000000000000, 28.91008700340000104 ) ) ;
#10188=( LENGTH_UNIT ( ) NAMED_UNIT ( * ) SI_UNIT ( .MILLI., .METRE. ) );
#10190=CIRCLE ( 'NONE', #19979, 18.64285714289999873 ) ;
#10198=CARTESIAN_POINT ( 'NONE',  ( -12.86092766119999986, -101.0535396030000044, -8.816187549039998572 ) ) ;
#10200=CARTESIAN_POINT ( 'NONE',  ( -17.06630915629999734, -92.84728946610000833, -23.47642349310000043 ) ) ;
#10201=CARTESIAN_POINT ( 'NONE',  ( -1.229525073969999882, -101.0685839089999831, -16.04536366179999973 ) ) ;
#10202=CARTESIAN_POINT ( 'NONE',  ( -4.794255386040000566, -107.5000000000000000, -8.775825618900000791 ) ) ;
#10203=DIRECTION ( 'NONE',  ( 0.8091158474751271035, 0.000000000000000000, 0.5876491686070922649 ) ) ;
#10204=CARTESIAN_POINT ( 'NONE',  ( 7.569553306790000491, -101.4254870009999934, 14.06091893229999990 ) ) ;
#10205=VERTEX_POINT ( 'NONE', #7299 ) ;
#10206=ADVANCED_FACE ( 'NONE', ( #12224 ), #18660, .F. ) ;
#10207=CARTESIAN_POINT ( 'NONE',  ( 12.39757656149999931, -101.6484611540000031, -10.11435096289999969 ) ) ;
#10208=CARTESIAN_POINT ( 'NONE',  ( -25.63355024200000187, -93.05538537040000335, -6.006632896850000236 ) ) ;
#10209=CARTESIAN_POINT ( 'NONE',  ( 11.86656066179999947, -101.3150700380000018, -11.10431109579999820 ) ) ;
#10215=CARTESIAN_POINT ( 'NONE',  ( -17.58183917889999748, -94.05395947819999947, 17.08481454950000256 ) ) ;
#10218=ADVANCED_FACE ( 'NONE', ( #8001 ), #27109, .T. ) ;
#10221=CARTESIAN_POINT ( 'NONE',  ( -0.03691758196609999654, -101.3138676899999950, -15.91402604900000028 ) ) ;
#10223=CARTESIAN_POINT ( 'NONE',  ( 15.64667777420000050, -100.8816835080000089, 2.154424203329999621 ) ) ;
#10227=CARTESIAN_POINT ( 'NONE',  ( 6.678590877449999574, -99.74726900420000675, 15.80215313019999890 ) ) ;
#10228=CARTESIAN_POINT ( 'NONE',  ( -15.63967876733211249, -92.57787461316036115, -24.03209257557816514 ) ) ;
#10229=CARTESIAN_POINT ( 'NONE',  ( -11.67413748739999946, -94.95684267580000437, -21.41802841999999885 ) ) ;
#10231=CARTESIAN_POINT ( 'NONE',  ( 5.011613449249795238, -92.66777315147957950, -30.08544135070622616 ) ) ;
#10232=CARTESIAN_POINT ( 'NONE',  ( -7.302336599650000259, -98.93445099689999722, 17.20095762220000069 ) ) ;
#10235=CARTESIAN_POINT ( 'NONE',  ( 9.011184001060000170, -94.54647010780000471, -23.25409275959999889 ) ) ;
#10236=VECTOR ( 'NONE', #26727, 1000.000000000000000 ) ;
#10238=ORIENTED_EDGE ( 'NONE', *, *, #19214, .T. ) ;
#10240=CARTESIAN_POINT ( 'NONE',  ( -5.854053644989999583, -101.0685849509999912, 14.98984533339999992 ) ) ;
#10245=CARTESIAN_POINT ( 'NONE',  ( 0.5204107913287318032, -100.1517898586199493, -17.17286546631214961 ) ) ;
#10246=CARTESIAN_POINT ( 'NONE',  ( 6.072376808220000477, -100.9137139110000021, 14.40534646189999890 ) ) ;
#10247=CARTESIAN_POINT ( 'NONE',  ( -13.09441083470000144, -92.84549618469999643, -23.96915825600000005 ) ) ;
#10255=CARTESIAN_POINT ( 'NONE',  ( 24.33664649176833095, -93.98969193921543308, -9.464842905525378214 ) ) ;
#10261=B_SPLINE_CURVE_WITH_KNOTS ( 'NONE', 3,
 ( #20596, #17821, #11389, #4705, #18116, #2232 ),
 .UNSPECIFIED., .F., .F.,
 ( 4, 2, 4 ),
 ( 0.000000000000000000, 0.5000000000000002220, 1.000000000000000000 ),
 .UNSPECIFIED. ) ;
#10264=CARTESIAN_POINT ( 'NONE',  ( -29.66597372489999884, -92.76843000840000286, 6.359924916739999823 ) ) ;
#10266=ORIENTED_EDGE ( 'NONE', *, *, #2149, .F. ) ;
#10268=ORIENTED_EDGE ( 'NONE', *, *, #4741, .F. ) ;
#10279=CARTESIAN_POINT ( 'NONE',  ( -15.48764535020000110, -101.3256027289999963, 3.628077442809999997 ) ) ;
#10281=CARTESIAN_POINT ( 'NONE',  ( -17.59440688584024315, -95.56535007417228655, 14.09092167176237531 ) ) ;
#10282=VERTEX_POINT ( 'NONE', #9427 ) ;
#10284=CARTESIAN_POINT ( 'NONE',  ( -12.36549121539999874, -100.9678331089999972, -10.43708019790000030 ) ) ;
#10286=CARTESIAN_POINT ( 'NONE',  ( -7.787505644985010633, -100.7538407668029379, 14.77225502553302583 ) ) ;
#10292=TOROIDAL_SURFACE ( 'NONE', #25237, 5.500000000000000000, 0.5000000000000000000 ) ;
#10293=AXIS2_PLACEMENT_3D ( 'NONE', #24325, #2044, #26964 ) ;
#10296=VERTEX_POINT ( 'NONE', #20512 ) ;
#10299=CARTESIAN_POINT ( 'NONE',  ( 27.11204721459999689, -92.54030572580001035, 9.444959058340000269 ) ) ;
#10303=CARTESIAN_POINT ( 'NONE',  ( -3.219077971254640236, -97.43430234703029669, -20.31490937506839600 ) ) ;
#10305=EDGE_CURVE ( 'NONE', #10296, #23041, #3183, .T. ) ;
#10307=CARTESIAN_POINT ( 'NONE',  ( 7.629218925470000023, -101.5342894280000081, 14.06592359269999903 ) ) ;
#10311=CARTESIAN_POINT ( 'NONE',  ( -15.04902548439999954, -98.73889367950000917, -10.99609012540000030 ) ) ;
#10313=CARTESIAN_POINT ( 'NONE',  ( -20.52074439609999956, -93.75380055729999640, 14.17856059480000042 ) ) ;
#10314=CARTESIAN_POINT ( 'NONE',  ( 24.04401824170000168, -94.24983875559999547, -8.202559790829997866 ) ) ;
#10326=AXIS2_PLACEMENT_3D ( 'NONE', #13086, #9741, #7284 ) ;
#10328=ORIENTED_EDGE ( 'NONE', *, *, #3414, .T. ) ;
#10330=ORIENTED_EDGE ( 'NONE', *, *, #8956, .T. ) ;
#10334=CARTESIAN_POINT ( 'NONE',  ( 9.279094190520000396, -98.48918237500001283, 16.48187022329999962 ) ) ;
#10335=EDGE_CURVE ( 'NONE', #22088, #21458, #2605, .T. ) ;
#10336=B_SPLINE_SURFACE_WITH_KNOTS ( 'NONE', 5, 5, ( 
 ( #25241, #12367, #23596, #3640, #10038, #18678 ),
 ( #12501, #21413, #27418, #7471, #23055, #3099 ),
 ( #924, #25653, #5683, #11952, #9766, #16480 ),
 ( #25382, #3237, #12094, #22368, #685, #27036 ),
 ( #7079, #22811, #18137, #22662, #7366, #9387 ),
 ( #18438, #9535, #11713, #24987, #386, #2854 ) ),
 .UNSPECIFIED., .F., .F., .F.,
 ( 6, 6 ),
 ( 6, 6 ),
 ( 15.82767921900000019, 30.79602961229999991 ),
 ( 0.000000000000000000, 0.5000000000000000000 ),
 .UNSPECIFIED. ) ;
#10337=CARTESIAN_POINT ( 'NONE',  ( -14.13789956389999958, -93.18831369829999289, -23.64158520889999693 ) ) ;
#10340=CARTESIAN_POINT ( 'NONE',  ( 1.810422456229999977, -92.75885938639999040, 27.42763845990000249 ) ) ;
#10344=ORIENTED_EDGE ( 'NONE', *, *, #7719, .F. ) ;
#10346=CARTESIAN_POINT ( 'NONE',  ( -27.14282719570000069, -92.75885938639999040, -4.338192340750000042 ) ) ;
#10352=AXIS2_PLACEMENT_3D ( 'NONE', #16790, #10066, #10203 ) ;
#10355=DIRECTION ( 'NONE',  ( 0.000000000000000000, 1.000000000000000000, 0.000000000000000000 ) ) ;
#10358=CARTESIAN_POINT ( 'NONE',  ( -0.1689899845689999958, -101.2530993010000060, -15.19297360289999865 ) ) ;
#10365=CARTESIAN_POINT ( 'NONE',  ( 6.266701257130000258, -100.8685038539999965, 14.42968300090000078 ) ) ;
#10366=CARTESIAN_POINT ( 'NONE',  ( 15.37132493649999887, -101.0678230150000019, 3.755183840060000389 ) ) ;
#10371=CARTESIAN_POINT ( 'NONE',  ( 25.33393120808624843, -93.66270333200125719, -5.817803472910904716 ) ) ;
#10373=TOROIDAL_SURFACE ( 'NONE', #8989, 21.14285714289999873, 0.5000000000000000000 ) ;
#10374=CARTESIAN_POINT ( 'NONE',  ( 3.220763788040000186, -92.54807930229999613, -28.60785095109999787 ) ) ;
#10376=CARTESIAN_POINT ( 'NONE',  ( -3.215510237749999778, -94.59276292389999696, 23.57860181210000405 ) ) ;
#10380=ORIENTED_EDGE ( 'NONE', *, *, #20788, .F. ) ;
#10383=TOROIDAL_SURFACE ( 'NONE', #21138, 18.14285714289999873, 0.5000000000000000000 ) ;
#10386=CARTESIAN_POINT ( 'NONE',  ( 13.22388793010019548, -92.80442066019948300, 27.48416330172907607 ) ) ;
#10391=CARTESIAN_POINT ( 'NONE',  ( -12.03627366839999802, -92.50000000000000000, 28.02459841239999960 ) ) ;
#10392=AXIS2_PLACEMENT_3D ( 'NONE', #20496, #17878, #2734 ) ;
#10395=ORIENTED_EDGE ( 'NONE', *, *, #15649, .T. ) ;
#10396=ORIENTED_EDGE ( 'NONE', *, *, #6006, .T. ) ;
#10400=CIRCLE ( 'NONE', #16948, 0.5000000000000013323 ) ;
#10405=CARTESIAN_POINT ( 'NONE',  ( -29.37337778839999913, -92.51542729400000553, 6.408755614549999535 ) ) ;
#10406=CARTESIAN_POINT ( 'NONE',  ( 8.920183199378271865, -94.54719627018464223, -22.12534656354277374 ) ) ;
#10408=ORIENTED_EDGE ( 'NONE', *, *, #3378, .F. ) ;
#10410=DIRECTION ( 'NONE',  ( 0.000000000000000000, 1.000000000000000000, 0.000000000000000000 ) ) ;
#10420=CARTESIAN_POINT ( 'NONE',  ( 23.54313657600000198, -94.98812477599999227, -6.784142512209999865 ) ) ;
#10421=CARTESIAN_POINT ( 'NONE',  ( -11.97505089750000096, -101.1848541609999899, -9.495040346209998816 ) ) ;
#10423=CARTESIAN_POINT ( 'NONE',  ( -7.693802629154737005, -100.9364580240060292, 14.65842723137789960 ) ) ;
#10424=ORIENTED_EDGE ( 'NONE', *, *, #15323, .T. ) ;
#10432=ORIENTED_EDGE ( 'NONE', *, *, #12108, .F. ) ;
#10437=CARTESIAN_POINT ( 'NONE',  ( 29.52540672639999997, -93.00000902169999506, 7.168157281560000982 ) ) ;
#10438=CARTESIAN_POINT ( 'NONE',  ( 15.50925563669999896, -100.9197081840000010, 1.894558565230000102 ) ) ;
#10443=DIRECTION ( 'NONE',  ( 1.000000000000000000, 0.000000000000000000, 0.000000000000000000 ) ) ;
#10445=ORIENTED_EDGE ( 'NONE', *, *, #20364, .F. ) ;
#10446=CARTESIAN_POINT ( 'NONE',  ( -22.24124375720000302, -94.63960162979999780, -8.291374127620001033 ) ) ;
#10447=CARTESIAN_POINT ( 'NONE',  ( 11.97048044210000128, -101.2358105800000061, -9.395351924210000760 ) ) ;
#10448=CARTESIAN_POINT ( 'NONE',  ( -19.74785546080000032, -92.58502690130001156, 20.72667931229999994 ) ) ;
#10449=CARTESIAN_POINT ( 'NONE',  ( 24.43035140000000283, -92.76004107139999633, -17.00416254499999980 ) ) ;
#10456=DIRECTION ( 'NONE',  ( 0.000000000000000000, 1.000000000000000000, 0.000000000000000000 ) ) ;
#10457=CARTESIAN_POINT ( 'NONE',  ( 20.53702927206556339, -97.42330310008513550, 1.367348661909628227 ) ) ;
#10461=ADVANCED_FACE ( 'NONE', ( #20626 ), #22684, .T. ) ;
#10462=EDGE_CURVE ( 'NONE', #9315, #11556, #12985, .T. ) ;
#10463=ORIENTED_EDGE ( 'NONE', *, *, #13273, .T. ) ;
#10470=ORIENTED_EDGE ( 'NONE', *, *, #23651, .F. ) ;
#10471=FACE_OUTER_BOUND ( 'NONE', #21119, .T. ) ;
#10473=CARTESIAN_POINT ( 'NONE',  ( -14.09262705500000123, -92.79515029379999191, -23.78749435689999814 ) ) ;
#10475=CARTESIAN_POINT ( 'NONE',  ( -1.604075271319999940, -100.9197075889999979, -15.54198525189999813 ) ) ;
#10477=VECTOR ( 'NONE', #14014, 1000.000000000000000 ) ;
#10480=CARTESIAN_POINT ( 'NONE',  ( 13.29192986090826878, -100.9364580246202081, -9.868570734956325197 ) ) ;
#10488=CARTESIAN_POINT ( 'NONE',  ( -17.83719336599999750, -93.71758747490000019, 18.24690405790000014 ) ) ;
#10489=CARTESIAN_POINT ( 'NONE',  ( 0.3059185938709999553, -93.00000000000000000, 14.72672055670000013 ) ) ;
#10492=CARTESIAN_POINT ( 'NONE',  ( -0.1779554536940000098, -101.5369810359999860, -15.99901033990000165 ) ) ;
#10493=CARTESIAN_POINT ( 'NONE',  ( 27.23269985219999967, -92.50000000000000000, -12.38957130830000075 ) ) ;
#10498=ADVANCED_FACE ( 'NONE', ( #24812, #8899 ), #7038, .T. ) ;
#10500=CARTESIAN_POINT ( 'NONE',  ( 6.523512041040000042, -100.2511768809999921, 15.35682148189999907 ) ) ;
#10501=CARTESIAN_POINT ( 'NONE',  ( 15.01705834989999921, -101.1411470200000053, 3.365801592560000000 ) ) ;
#10506=CARTESIAN_POINT ( 'NONE',  ( 8.149626591600000580, -93.87552273900000444, -23.44626940270000048 ) ) ;
#10507=DIRECTION ( 'NONE',  ( 1.000000000000000000, 0.000000000000000000, 0.000000000000000000 ) ) ;
#10509=CARTESIAN_POINT ( 'NONE',  ( 6.019093083229999586, -92.50000000000000000, 29.30685818879999971 ) ) ;
#10512=CARTESIAN_POINT ( 'NONE',  ( -12.49059627124878347, -101.1742791177312597, -10.57827074192917571 ) ) ;
#10515=CARTESIAN_POINT ( 'NONE',  ( -1.381305061119999955, -100.8816835080000089, -15.73378738089999729 ) ) ;
#10518=DIRECTION ( 'NONE',  ( 0.4794255386042038936, 0.000000000000000000, 0.8775825618903723147 ) ) ;
#10519=CARTESIAN_POINT ( 'NONE',  ( -13.32816333360000094, -111.0000000000000000, -11.12411022969999941 ) ) ;
#10521=CARTESIAN_POINT ( 'NONE',  ( 16.09608533816492226, -94.75169073774321760, 17.24760066427640837 ) ) ;
#10525=CARTESIAN_POINT ( 'NONE',  ( 24.24250217843501076, -94.10917102468839346, -9.048685009091679277 ) ) ;
#10532=CARTESIAN_POINT ( 'NONE',  ( -28.98397190429999881, -92.96321827540000982, 3.119460853480000129 ) ) ;
#10535=CARTESIAN_POINT ( 'NONE',  ( 15.58177396959999861, -100.4808658609999981, 4.510597657439999963 ) ) ;
#10545=CARTESIAN_POINT ( 'NONE',  ( 11.70455088819999823, -93.00000000000000000, 8.942783294160001617 ) ) ;
#10550=CARTESIAN_POINT ( 'NONE',  ( -12.07947227870000084, -101.0956037589999994, -9.784155217600000398 ) ) ;
#10551=EDGE_CURVE ( 'NONE', #21931, #25380, #11235, .T. ) ;
#10553=FACE_OUTER_BOUND ( 'NONE', #20731, .T. ) ;
#10561=B_SPLINE_SURFACE_WITH_KNOTS ( 'NONE', 5, 5, ( 
 ( #21600, #10492, #10080, #8060, #3682, #8467, #27875, #14613, #10358 ),
 ( #23643, #26113, #21318, #1787, #19273, #15013, #23515, #19545, #18996 ),
 ( #1374, #7922, #16806, #10221, #25841, #5863, #12545, #21460, #14877 ),
 ( #17078, #28159, #8192, #25972, #3824, #19407, #22476, #24360, #8745 ),
 ( #26546, #15152, #12971, #20129, #11060, #4688, #24502, #15449, #24656 ),
 ( #20277, #2367, #26399, #19975, #15603, #24216, #6286, #8611, #4250 ),
 ( #8893, #26698, #6429, #13122, #10921, #28705, #17662, #6587, #4539 ),
 ( #11374, #19687, #21884, #15746, #15292, #48, #11223, #19828, #198 ),
 ( #24062, #1935, #2518, #4401, #13268, #344, #22177, #17369, #6739 ),
 ( #17807, #22034, #2217, #13417, #22319, #17513, #26265, #9048, #17952 ),
 ( #26846, #4101, #10775, #6880, #13567, #28577, #2082, #7320, #16489 ),
 ( #23066, #18244, #2959, #7480, #16047, #26993, #494, #24949, #642 ) ),
 .UNSPECIFIED., .F., .F., .F.,
 ( 6, 3, 3, 6 ),
 ( 6, 3, 6 ),
 ( 3.852920539459999905, 4.834764074400000666, 6.134713715030000181, 8.383984506220000910 ),
 ( 0.000000000000000000, 0.2500000000000000000, 0.5000000000000000000 ),
 .UNSPECIFIED. ) ;
#10566=CARTESIAN_POINT ( 'NONE',  ( -19.49896612583845013, -96.70003212931756309, 8.002497787980619393 ) ) ;
#10571=ORIENTED_EDGE ( 'NONE', *, *, #3212, .F. ) ;
#10572=CARTESIAN_POINT ( 'NONE',  ( -3.225656763162762175, -97.43022994611277454, -20.31916069606105069 ) ) ;
#10575=FACE_OUTER_BOUND ( 'NONE', #16119, .T. ) ;
#10577=EDGE_LOOP ( 'NONE', ( #6661, #22850, #10161, #18708, #1887, #25631, #12356 ) ) ;
#10579=CARTESIAN_POINT ( 'NONE',  ( -18.72456657609999908, -96.53848370309999893, -10.28520937999999951 ) ) ;
#10580=CARTESIAN_POINT ( 'NONE',  ( 12.97255956529999921, -101.0405520670000072, -9.781797840599999461 ) ) ;
#10592=DIRECTION ( 'NONE',  ( 0.000000000000000000, 1.000000000000000000, 0.000000000000000000 ) ) ;
#10593=CARTESIAN_POINT ( 'NONE',  ( 0.03892854975575889276, -92.83160374581088092, -30.49997535110724911 ) ) ;
#10603=CARTESIAN_POINT ( 'NONE',  ( -12.76745321220000129, -101.1364147039999892, -8.514038431850000421 ) ) ;
#10607=LINE ( 'NONE', #1767, #21051 ) ;
#10609=CIRCLE ( 'NONE', #4601, 30.50000000000000000 ) ;
#10611=DIRECTION ( 'NONE',  ( 0.4794255386042038936, 0.000000000000000000, 0.8775825618903723147 ) ) ;
#10614=CARTESIAN_POINT ( 'NONE',  ( -29.70568929799252800, -92.71346081467955003, 6.915347693732913470 ) ) ;
#10617=CARTESIAN_POINT ( 'NONE',  ( 12.73554887757679310, -101.5026031440401368, -9.870240380742313135 ) ) ;
#10620=CARTESIAN_POINT ( 'NONE',  ( -15.84587239670000258, -101.4177331369999990, 3.264600553649999792 ) ) ;
#10626=CARTESIAN_POINT ( 'NONE',  ( -20.57915330399717746, -93.03394437611173373, 17.00111121841682760 ) ) ;
#10630=VECTOR ( 'NONE', #15894, 1000.000000000000000 ) ;
#10639=CARTESIAN_POINT ( 'NONE',  ( 6.737873477499999986, -100.1459902240000019, 15.55874246810000017 ) ) ;
#10640=CARTESIAN_POINT ( 'NONE',  ( 15.75714761940000308, -101.3090757639999993, 4.024255779760000706 ) ) ;
#10641=ORIENTED_EDGE ( 'NONE', *, *, #129, .T. ) ;
#10644=CARTESIAN_POINT ( 'NONE',  ( 0.000000000000000000, -94.59276292389999696, 0.000000000000000000 ) ) ;
#10646=CARTESIAN_POINT ( 'NONE',  ( 1.957052877659999801, -92.91851489729999969, -29.74816621520000126 ) ) ;
#10647=CARTESIAN_POINT ( 'NONE',  ( 7.102042752109999135, -101.6484611540000031, 14.33739825589999839 ) ) ;
#10648=CARTESIAN_POINT ( 'NONE',  ( -6.752147290549999958, -101.1180794200000008, 13.97358175370000133 ) ) ;
#10649=ORIENTED_EDGE ( 'NONE', *, *, #27516, .T. ) ;
#10651=CARTESIAN_POINT ( 'NONE',  ( -12.48059356133589226, -101.2111896144776324, -10.54544150875332065 ) ) ;
#10659=CARTESIAN_POINT ( 'NONE',  ( -29.21843812340000213, -92.50000000000000000, 6.434616699369999360 ) ) ;
#10668=CARTESIAN_POINT ( 'NONE',  ( 13.75075768692672540, -100.1517898586340038, -10.30023294644368903 ) ) ;
#10671=CARTESIAN_POINT ( 'NONE',  ( 8.125631349740000786, -93.00000000000000000, 24.17072847820000092 ) ) ;
#10676=CIRCLE ( 'NONE', #1432, 6.000000000000000000 ) ;
#10679=DIRECTION ( 'NONE',  ( 1.000000000000000000, 0.000000000000000000, 0.000000000000000000 ) ) ;
#10681=CARTESIAN_POINT ( 'NONE',  ( 0.000000000000000000, -107.5000000000000000, 0.000000000000000000 ) ) ;
#10685=ORIENTED_EDGE ( 'NONE', *, *, #27258, .T. ) ;
#10694=FACE_OUTER_BOUND ( 'NONE', #16638, .T. ) ;
#10696=CARTESIAN_POINT ( 'NONE',  ( -29.86363316589999783, -93.00000000000000000, 0.3450520983969999622 ) ) ;
#10700=CARTESIAN_POINT ( 'NONE',  ( -7.834619151519719438, -100.6338045035611515, 14.85527437501940362 ) ) ;
#10702=CARTESIAN_POINT ( 'NONE',  ( -1.283023294879999998, -101.3150694429999987, -16.20107482390000087 ) ) ;
#10703=CARTESIAN_POINT ( 'NONE',  ( 6.114061450890000415, -111.0000000000000000, -13.40104985119999981 ) ) ;
#10708=CARTESIAN_POINT ( 'NONE',  ( 12.02508340220000171, -92.51167569919999778, 27.24521537120000048 ) ) ;
#10713=CARTESIAN_POINT ( 'NONE',  ( -16.34073580590758112, -93.59825774987527325, -21.52464356387743294 ) ) ;
#10722=CARTESIAN_POINT ( 'NONE',  ( -16.46937899769999802, -93.21603264569999681, -21.54563518039999792 ) ) ;
#10723=CARTESIAN_POINT ( 'NONE',  ( -17.05574026919999753, -93.34713166629998682, 21.78488634390000200 ) ) ;
#10726=CARTESIAN_POINT ( 'NONE',  ( 13.23566414709999961, -100.6809449770000100, -9.745096673970000012 ) ) ;
#10729=AXIS2_PLACEMENT_3D ( 'NONE', #22173, #27281, #15895 ) ;
#10730=CARTESIAN_POINT ( 'NONE',  ( 30.00028607799999847, -92.50000000000000000, 5.498439345520000465 ) ) ;
#10733=CIRCLE ( 'NONE', #27074, 15.19391340349999986 ) ;
#10737=CARTESIAN_POINT ( 'NONE',  ( 4.420730772149999765, -92.67327634539999792, -27.51018170170000232 ) ) ;
#10740=B_SPLINE_SURFACE_WITH_KNOTS ( 'NONE', 5, 5, ( 
 ( #3191, #27673, #13293, #24087, #23952, #16718 ),
 ( #15319, #14523, #23426, #28310, #28600, #12997 ),
 ( #10002, #22197, #12846, #18915, #3465, #22059 ),
 ( #27795, #1811, #24239, #1959, #17249, #12331 ),
 ( #26570, #21239, #19572, #28458, #17394, #26426 ),
 ( #8769, #26288, #21760, #6312, #3987, #8495 ) ),
 .UNSPECIFIED., .F., .F., .F.,
 ( 6, 6 ),
 ( 6, 6 ),
 ( 7.179431123200000542, 23.44689954300000068 ),
 ( 0.000000000000000000, 0.5000000000000000000 ),
 .UNSPECIFIED. ) ;
#10743=CARTESIAN_POINT ( 'NONE',  ( -11.85289073049999864, -94.98812769020000246, -21.44326021599999876 ) ) ;
#10747=CARTESIAN_POINT ( 'NONE',  ( 19.60969031579999822, -98.43722211769998864, -0.3265172099129999839 ) ) ;
#10751=ADVANCED_FACE ( 'NONE', ( #19624 ), #7857, .T. ) ;
#10752=ORIENTED_EDGE ( 'NONE', *, *, #91, .F. ) ;
#10754=CARTESIAN_POINT ( 'NONE',  ( 16.54056940490000116, -94.89196973119999257, 16.94454239999999956 ) ) ;
#10758=CARTESIAN_POINT ( 'NONE',  ( 7.286238495500000134, -101.2500498790000023, 13.33737010350000141 ) ) ;
#10759=CARTESIAN_POINT ( 'NONE',  ( -30.39212651620044170, -92.86276748823678417, 2.566209473271955144 ) ) ;
#10763=ORIENTED_EDGE ( 'NONE', *, *, #20681, .F. ) ;
#10764=CARTESIAN_POINT ( 'NONE',  ( 13.42574138988457655, -100.7538407676048848, -9.930469818722173159 ) ) ;
#10767=CARTESIAN_POINT ( 'NONE',  ( 8.831073959190000267, -94.59276583650000703, -22.09757114230000141 ) ) ;
#10770=CARTESIAN_POINT ( 'NONE',  ( -15.25386055589999934, -92.94769410010000854, 25.12374163710000019 ) ) ;
#10771=CARTESIAN_POINT ( 'NONE',  ( -20.34767246214833847, -92.64526570559976903, 19.18952924589508413 ) ) ;
#10772=VERTEX_POINT ( 'NONE', #9126 ) ;
#10775=CARTESIAN_POINT ( 'NONE',  ( 0.5694848120150000081, -99.99711545080000974, -17.16320790510000194 ) ) ;
#10777=CARTESIAN_POINT ( 'NONE',  ( 15.03693308380000104, -101.1848541609999899, 2.726188632040000392 ) ) ;
#10781=VERTEX_POINT ( 'NONE', #13651 ) ;
#10783=CARTESIAN_POINT ( 'NONE',  ( 15.12841431370000045, -101.0956037589999994, 3.574132650939999767 ) ) ;
#10784=CARTESIAN_POINT ( 'NONE',  ( -5.902985309178900408, -97.42330309878559547, 19.71785937141702405 ) ) ;
#10786=ORIENTED_EDGE ( 'NONE', *, *, #10551, .F. ) ;
#10787=CARTESIAN_POINT ( 'NONE',  ( -16.44063509269999912, -92.87228942340000515, 21.55809250360000107 ) ) ;
#10788=CARTESIAN_POINT ( 'NONE',  ( 4.811931075225057697, -92.71525149899693474, -30.11819794593843724 ) ) ;
#10789=CARTESIAN_POINT ( 'NONE',  ( -4.472380792810000116, -95.66919271819999437, 22.06157936329999814 ) ) ;
#10791=CARTESIAN_POINT ( 'NONE',  ( 4.725730692399999988, -92.90721294759998727, -27.95382239220000287 ) ) ;
#10794=CARTESIAN_POINT ( 'NONE',  ( -15.42268960139999834, -101.1889999979999999, 4.259183661159999801 ) ) ;
#10796=ORIENTED_EDGE ( 'NONE', *, *, #14963, .T. ) ;
#10797=AXIS2_PLACEMENT_3D ( 'NONE', #19152, #12010, #8078 ) ;
#10799=AXIS2_PLACEMENT_3D ( 'NONE', #17604, #24596, #20222 ) ;
#10800=CARTESIAN_POINT ( 'NONE',  ( -13.10181604453989124, -100.1517898586368460, -11.11398002738276070 ) ) ;
#10801=ORIENTED_EDGE ( 'NONE', *, *, #129, .F. ) ;
#10803=CIRCLE ( 'NONE', #27144, 18.64285714289999873 ) ;
#10806=CARTESIAN_POINT ( 'NONE',  ( 9.753760903854669095, -93.20709273739691980, -25.68565009221217466 ) ) ;
#10809=CARTESIAN_POINT ( 'NONE',  ( -19.89498170407338407, -92.54383083955177369, -23.11796002674290307 ) ) ;
#10810=VERTEX_POINT ( 'NONE', #28511 ) ;
#10811=CARTESIAN_POINT ( 'NONE',  ( -15.13778281370000123, -101.1716780380000102, 4.291020750220000401 ) ) ;
#10816=CARTESIAN_POINT ( 'NONE',  ( 13.74822071429026771, -100.1585711159249570, -10.29449286259888297 ) ) ;
#10818=CARTESIAN_POINT ( 'NONE',  ( 24.52093283500401455, -93.74885976995108194, -10.40268822211655397 ) ) ;
#10821=CARTESIAN_POINT ( 'NONE',  ( -13.18688177930000016, -93.32822605769999313, -23.58441486170000090 ) ) ;
#10826=CARTESIAN_POINT ( 'NONE',  ( -24.06374496360000137, -94.22763312380000400, -3.197736329870000116 ) ) ;
#10828=CARTESIAN_POINT ( 'NONE',  ( 0.000000000000000000, -101.1889999979999999, 0.000000000000000000 ) ) ;
#10836=B_SPLINE_CURVE_WITH_KNOTS ( 'NONE', 5,
 ( #24229, #19839, #11387, #28720, #8759, #7046 ),
 .UNSPECIFIED., .F., .F.,
 ( 6, 6 ),
 ( 0.000000000000000000, 1.000000000000000000 ),
 .UNSPECIFIED. ) ;
#10841=CARTESIAN_POINT ( 'NONE',  ( -17.60247688846170888, -95.05882272216540230, 15.10979806272066917 ) ) ;
#10842=EDGE_CURVE ( 'NONE', #2729, #14760, #10992, .T. ) ;
#10845=CARTESIAN_POINT ( 'NONE',  ( -12.44240347620000087, -101.3878691800000098, -10.22198205940000015 ) ) ;
#10851=EDGE_LOOP ( 'NONE', ( #28444, #21277, #612, #17736 ) ) ;
#10858=CARTESIAN_POINT ( 'NONE',  ( -19.88469613148559390, -96.02299627876102761, 9.294782919059894510 ) ) ;
#10860=CARTESIAN_POINT ( 'NONE',  ( 22.06554121350000131, -93.81709728810000115, 13.31880052350000021 ) ) ;
#10862=ORIENTED_EDGE ( 'NONE', *, *, #7322, .T. ) ;
#10865=TOROIDAL_SURFACE ( 'NONE', #3042, 5.500000000000000000, 0.5000000000000000000 ) ;
#10867=CARTESIAN_POINT ( 'NONE',  ( 12.44788637039999912, -101.5369810359999860, -10.05268415809999993 ) ) ;
#10868=CARTESIAN_POINT ( 'NONE',  ( -20.30146180590000071, -92.55031878709998239, -20.19289408079999859 ) ) ;
#10869=CARTESIAN_POINT ( 'NONE',  ( 6.114061450880000415, -93.00000000000000000, -13.40104985119999981 ) ) ;
#10872=CARTESIAN_POINT ( 'NONE',  ( 12.57051157029999899, -101.4908759489999994, -9.948597786639998830 ) ) ;
#10874=EDGE_CURVE ( 'NONE', #15494, #13209, #11185, .T. ) ;
#10883=PLANE ( 'NONE',  #25946 ) ;
#10886=CARTESIAN_POINT ( 'NONE',  ( -0.1318277626668340474, -92.71346081467603994, -30.49971527465584842 ) ) ;
#10889=B_SPLINE_CURVE_WITH_KNOTS ( 'NONE', 3,
 ( #1079, #3246, #18245, #25522, #27286, #5558 ),
 .UNSPECIFIED., .F., .F.,
 ( 4, 2, 4 ),
 ( 0.000000000000000000, 0.5000000000000000000, 1.000000000000000000 ),
 .UNSPECIFIED. ) ;
#10891=CARTESIAN_POINT ( 'NONE',  ( -11.38188502134437385, -94.78087563376180924, -20.62155828120727108 ) ) ;
#10894=CARTESIAN_POINT ( 'NONE',  ( 19.67779709110000042, -98.51736893609999868, -0.3242707669709999907 ) ) ;
#10902=CARTESIAN_POINT ( 'NONE',  ( -4.523871465800000990, -98.54854614750000508, -18.92597532359999946 ) ) ;
#10904=CARTESIAN_POINT ( 'NONE',  ( -20.19758353400000317, -95.55441921500001001, 10.16704513559999867 ) ) ;
#10905=CARTESIAN_POINT ( 'NONE',  ( -29.54921749321805180, -92.53260370677851654, 7.556178546955753639 ) ) ;
#10906=CARTESIAN_POINT ( 'NONE',  ( 6.880103916109999496, -101.6484611540000031, 13.88935456040000105 ) ) ;
#10908=SHAPE_REPRESENTATION ( 'Coolant Impeller Vanes', ( #26433 ), #17143 ) ;
#10911=DIRECTION ( 'NONE',  ( 1.000000000000000000, 0.000000000000000000, 0.000000000000000000 ) ) ;
#10913=ORIENTED_EDGE ( 'NONE', *, *, #24174, .T. ) ;
#10916=CARTESIAN_POINT ( 'NONE',  ( -13.45765177410000035, -92.63554508160000012, 27.09946297289999961 ) ) ;
#10918=ORIENTED_EDGE ( 'NONE', *, *, #18879, .T. ) ;
#10921=CARTESIAN_POINT ( 'NONE',  ( 0.5104505476449999746, -100.8455998110000138, -16.03521346039999784 ) ) ;
#10923=CARTESIAN_POINT ( 'NONE',  ( 15.65153732499999961, -101.3256027139999986, 2.837616081620000230 ) ) ;
#10929=CARTESIAN_POINT ( 'NONE',  ( 12.39757656149999931, -101.1889999979999999, -10.11435096289999969 ) ) ;
#10931=CARTESIAN_POINT ( 'NONE',  ( -17.00181101289999930, -93.27295844349998788, 19.70561590980000233 ) ) ;
#10934=AXIS2_PLACEMENT_3D ( 'NONE', #26879, #8784, #8933 ) ;
#10935=CARTESIAN_POINT ( 'NONE',  ( 26.66586667100000341, -92.50000467790000869, 13.56662017419999877 ) ) ;
#10941=DIRECTION ( 'NONE',  ( -0.000000000000000000, 1.000000000000000000, 0.000000000000000000 ) ) ;
#10943=CARTESIAN_POINT ( 'NONE',  ( 8.825526648140000319, -98.73826279789999205, 16.36868468389999620 ) ) ;
#10946=CARTESIAN_POINT ( 'NONE',  ( -20.82481777699772607, -92.81370807121814437, -22.28401471726260041 ) ) ;
#10947=CARTESIAN_POINT ( 'NONE',  ( -15.12459707010000010, -101.1499364180000100, 4.397920892620000188 ) ) ;
#10949=CARTESIAN_POINT ( 'NONE',  ( -7.630334818519999729, -100.8023006570000035, 13.80849637110000039 ) ) ;
#10955=CARTESIAN_POINT ( 'NONE',  ( 24.75663061290020650, -93.31462968082412601, -12.91046299435144817 ) ) ;
#10963=LINE ( 'NONE', #19873, #14071 ) ;
#10965=CARTESIAN_POINT ( 'NONE',  ( -26.67277937040000069, -92.98481302140000082, -0.3354105345299999708 ) ) ;
#10979=CARTESIAN_POINT ( 'NONE',  ( -14.79537251110000007, -100.9197086940000077, 5.022279785309999411 ) ) ;
#10982=CARTESIAN_POINT ( 'NONE',  ( -15.40337430839999833, -101.5317003319999998, 4.643717924509999762 ) ) ;
#10984=CARTESIAN_POINT ( 'NONE',  ( 8.185346967789998374, -101.3150701389999995, 14.03998109830000018 ) ) ;
#10985=CARTESIAN_POINT ( 'NONE',  ( 9.385332722619999402, -98.68450614990000247, 16.47661810339999988 ) ) ;
#10986=ORIENTED_EDGE ( 'NONE', *, *, #27899, .T. ) ;
#10988=CARTESIAN_POINT ( 'NONE',  ( -0.7724858235186301547, -101.6484611540000031, -15.98142581210590762 ) ) ;
#10989=CARTESIAN_POINT ( 'NONE',  ( -13.09441083470000144, -92.84549618469999643, -23.96915825600000005 ) ) ;
#10992=LINE ( 'NONE', #16267, #23331 ) ;
#10993=CARTESIAN_POINT ( 'NONE',  ( -5.884306709680000580, -101.1461869959999973, 15.04985507670000011 ) ) ;
#10995=ORIENTED_EDGE ( 'NONE', *, *, #17035, .T. ) ;
#10999=CARTESIAN_POINT ( 'NONE',  ( 21.07836655800000258, -93.85715932649999615, 13.25903705600000038 ) ) ;
#11003=CARTESIAN_POINT ( 'NONE',  ( -22.29269500190000386, -94.98812477769999418, -8.065858985560000249 ) ) ;
#11005=CARTESIAN_POINT ( 'NONE',  ( 12.29187919760000014, -101.1617736559999940, -9.834676144290000366 ) ) ;
#11006=DIRECTION ( 'NONE',  ( 0.000000000000000000, -1.000000000000000000, 0.000000000000000000 ) ) ;
#11010=CARTESIAN_POINT ( 'NONE',  ( -1.449832362199999780, -100.8733988930000010, -15.65780151839999945 ) ) ;
#11011=EDGE_CURVE ( 'NONE', #10810, #17507, #19141, .T. ) ;
#11021=CARTESIAN_POINT ( 'NONE',  ( -7.105427357599999217E-15, -101.6484611540000031, -1.598721155459999804E-14 ) ) ;
#11024=CARTESIAN_POINT ( 'NONE',  ( 0.1200718050890000055, -91.50000000000000000, -30.49976365090000030 ) ) ;
#11028=CARTESIAN_POINT ( 'NONE',  ( -11.64049356306891347, -94.65527814842015175, -20.66310145454055558 ) ) ;
#11030=EDGE_CURVE ( 'NONE', #23088, #17197, #15887, .T. ) ;
#11031=CARTESIAN_POINT ( 'NONE',  ( 22.04471494010000043, -95.70830610080000156, -4.438274023730000017 ) ) ;
#11039=B_SPLINE_SURFACE_WITH_KNOTS ( 'NONE', 5, 5, ( 
 ( #9657, #14190, #6908, #24682, #16514, #25689 ),
 ( #16649, #28147, #9800, #25543, #23086, #20897 ),
 ( #5581, #14466, #17068, #10346, #7776, #19259 ),
 ( #25830, #5852, #25962, #3672, #10208, #19122 ),
 ( #23359, #1232, #5986, #25411, #23220, #7912 ),
 ( #12269, #23633, #18853, #21449, #16797, #14734 ) ),
 .UNSPECIFIED., .F., .F., .F.,
 ( 6, 6 ),
 ( 6, 6 ),
 ( 7.179431122970000523, 23.44689954309999891 ),
 ( 0.000000000000000000, 0.5000000000000000000 ),
 .UNSPECIFIED. ) ;
#11041=CARTESIAN_POINT ( 'NONE',  ( -11.23277242420000022, -95.05245081340000013, -21.31917440760000204 ) ) ;
#11042=CARTESIAN_POINT ( 'NONE',  ( 1.342713516450000144, -94.57749834670001121, 24.16140173950000047 ) ) ;
#11043=DIRECTION ( 'NONE',  ( 1.000000000000000000, 0.000000000000000000, 0.000000000000000000 ) ) ;
#11044=CARTESIAN_POINT ( 'NONE',  ( -29.45136854416018224, -92.49999999999997158, 7.930057420454290629 ) ) ;
#11047=CIRCLE ( 'NONE', #28750, 18.14285714289999873 ) ;
#11052=CARTESIAN_POINT ( 'NONE',  ( -13.27471559884043728, -92.83865970264245959, 27.45964197909431093 ) ) ;
#11053=ORIENTED_EDGE ( 'NONE', *, *, #5975, .T. ) ;
#11055=CARTESIAN_POINT ( 'NONE',  ( -13.54698799950000065, -92.84291960289999679, 27.17977165490000147 ) ) ;
#11056=CARTESIAN_POINT ( 'NONE',  ( -14.34373124439999891, -102.5000000000000000, -26.25602392650000283 ) ) ;
#11057=VERTEX_POINT ( 'NONE', #15575 ) ;
#11058=CARTESIAN_POINT ( 'NONE',  ( 11.70455088819999823, -92.50000000000000000, 8.942783294160001617 ) ) ;
#11060=CARTESIAN_POINT ( 'NONE',  ( 0.2405919600229999844, -101.0678230150000019, -15.82154074309999991 ) ) ;
#11062=CARTESIAN_POINT ( 'NONE',  ( 15.17121247040000043, -101.1411470150000014, 2.586268237070000087 ) ) ;
#11067=CARTESIAN_POINT ( 'NONE',  ( 28.34932843007601377, -92.75430643202088277, 11.25025375756242951 ) ) ;
#11070=CARTESIAN_POINT ( 'NONE',  ( -2.903043064769999848, -94.98812477769999418, 23.52859639729999941 ) ) ;
#11073=CARTESIAN_POINT ( 'NONE',  ( 20.51117185680000077, -93.49005502510000554, 16.28046590780000002 ) ) ;
#11077=CARTESIAN_POINT ( 'NONE',  ( -6.842500939620000722, -101.1402801299999936, 13.72981480590000025 ) ) ;
#11080=CARTESIAN_POINT ( 'NONE',  ( -12.88540406179054187, -100.4166221067027323, -11.03975155362831551 ) ) ;
#11085=CARTESIAN_POINT ( 'NONE',  ( -6.665307709260000379, -93.00000000000000000, -13.13558364449999871 ) ) ;
#11087=CARTESIAN_POINT ( 'NONE',  ( -7.593123957489999576, -94.98812477769999418, -22.45811603920000010 ) ) ;
#11089=CARTESIAN_POINT ( 'NONE',  ( 14.03681164164373563, -92.52048598158043546, 27.07800181827376207 ) ) ;
#11091=CARTESIAN_POINT ( 'NONE',  ( -14.76791303109999909, -100.9938288390000025, 4.803350814669999913 ) ) ;
#11093=CARTESIAN_POINT ( 'NONE',  ( 16.28649422715901451, -94.66088193484175406, 17.22963786743054371 ) ) ;
#11103=CARTESIAN_POINT ( 'NONE',  ( 25.11232611503765710, -93.38817447853173803, 11.60437395511254266 ) ) ;
#11108=CARTESIAN_POINT ( 'NONE',  ( -18.69985100922852084, -92.84292036730930420, 22.78328761814548997 ) ) ;
#11109=CARTESIAN_POINT ( 'NONE',  ( -27.15805213390000006, -93.30149055180000062, -0.5667321042260000663 ) ) ;
#11114=EDGE_CURVE ( 'NONE', #3774, #28309, #7296, .T. ) ;
#11120=CARTESIAN_POINT ( 'NONE',  ( -13.25045755180000029, -101.1889999979999999, -10.32789304109999939 ) ) ;
#11123=CARTESIAN_POINT ( 'NONE',  ( 6.981684465299999864, -111.0000000000000000, 29.03810821740000137 ) ) ;
#11127=CARTESIAN_POINT ( 'NONE',  ( -24.64364036189999752, -92.50000000000000000, -17.97055897050000084 ) ) ;
#11130=CARTESIAN_POINT ( 'NONE',  ( 24.27280310300000110, -92.97898997910000674, -11.25989722030000095 ) ) ;
#11133=CARTESIAN_POINT ( 'NONE',  ( 14.17788327750000121, -97.64874574789999429, -14.06651099139999950 ) ) ;
#11137=CARTESIAN_POINT ( 'NONE',  ( -12.60239484230000073, -99.94549701829998867, -11.26274910859999956 ) ) ;
#11140=CARTESIAN_POINT ( 'NONE',  ( 11.90927564517308745, -97.32634609770845202, 16.96552214579065776 ) ) ;
#11148=DIRECTION ( 'NONE',  ( 0.4794255386042036715, 0.000000000000000000, 0.8775825618903723147 ) ) ;
#11149=CARTESIAN_POINT ( 'NONE',  ( -5.145566427369999474, -99.82967635509999127, 17.17619540129999933 ) ) ;
#11150=CARTESIAN_POINT ( 'NONE',  ( -17.84952165019772607, -94.52419090328167783, 16.07137172613918707 ) ) ;
#11153=DIRECTION ( 'NONE',  ( 1.000000000000000000, 0.000000000000000000, 0.000000000000000000 ) ) ;
#11155=CARTESIAN_POINT ( 'NONE',  ( -26.02252412820971017, -93.99439547200873335, -2.045450153116517900 ) ) ;
#11156=CARTESIAN_POINT ( 'NONE',  ( 19.64032065480000000, -94.52419443349998573, 13.82578161140000006 ) ) ;
#11161=CARTESIAN_POINT ( 'NONE',  ( -24.72072344461773952, -93.86980009075321618, -6.303046593384079799 ) ) ;
#11163=EDGE_CURVE ( 'NONE', #14989, #11899, #558, .T. ) ;
#11167=CARTESIAN_POINT ( 'NONE',  ( -13.28804895260000052, -94.06807348040000250, -21.53763003719999958 ) ) ;
#11170=CARTESIAN_POINT ( 'NONE',  ( 0.000000000000000000, -101.2530993010000060, 0.000000000000000000 ) ) ;
#11171=CARTESIAN_POINT ( 'NONE',  ( -17.05934341600000081, -99.58396357329999660, 3.231284207160000310 ) ) ;
#11173=CARTESIAN_POINT ( 'NONE',  ( 0.1200718050890000055, -111.0000000000000000, -30.49976365090000030 ) ) ;
#11174=CARTESIAN_POINT ( 'NONE',  ( -5.719111655694421259, -98.21781671762684596, -19.46371341358546658 ) ) ;
#11175=DIRECTION ( 'NONE',  ( 0.000000000000000000, -1.000000000000000000, 0.000000000000000000 ) ) ;
#11178=ORIENTED_EDGE ( 'NONE', *, *, #12743, .F. ) ;
#11179=CARTESIAN_POINT ( 'NONE',  ( -9.671059929650001052, -94.07042739149999022, -23.11466436250000100 ) ) ;
#11181=DIRECTION ( 'NONE',  ( 1.000000000000000000, 0.000000000000000000, 0.000000000000000000 ) ) ;
#11184=B_SPLINE_CURVE_WITH_KNOTS ( 'NONE', 3,
 ( #27410, #18812, #16027, #7741, #11800, #11942 ),
 .UNSPECIFIED., .F., .F.,
 ( 4, 2, 4 ),
 ( 0.000000000000000000, 0.5000000000000000000, 1.000000000000000000 ),
 .UNSPECIFIED. ) ;
#11185=CIRCLE ( 'NONE', #14481, 29.91857981989999971 ) ;
#11191=CARTESIAN_POINT ( 'NONE',  ( -11.77049175740000209, -94.59276292389999696, -20.68200892780000189 ) ) ;
#11193=EDGE_CURVE ( 'NONE', #726, #21723, #17746, .T. ) ;
#11194=CARTESIAN_POINT ( 'NONE',  ( 19.09127226800000088, -98.29702512280000803, -0.7133363862450000648 ) ) ;
#11198=ORIENTED_EDGE ( 'NONE', *, *, #21421, .F. ) ;
#11201=CARTESIAN_POINT ( 'NONE',  ( -11.31661412480000095, -95.23933631519999210, -21.36055902369999870 ) ) ;
#11202=CARTESIAN_POINT ( 'NONE',  ( 7.804759209956171340, -94.00303307110470996, -24.89030770455894270 ) ) ;
#11206=AXIS2_PLACEMENT_3D ( 'NONE', #11056, #2662, #42 ) ;
#11209=AXIS2_PLACEMENT_3D ( 'NONE', #15536, #13351, #11153 ) ;
#11211=AXIS2_PLACEMENT_3D ( 'NONE', #11586, #8970, #26776 ) ;
#11216=CARTESIAN_POINT ( 'NONE',  ( -16.76064802440000179, -92.85978345570001125, 21.58520938940000278 ) ) ;
#11217=DIRECTION ( 'NONE',  ( 1.000000000000000000, 0.000000000000000000, 0.000000000000000000 ) ) ;
#11221=CARTESIAN_POINT ( 'NONE',  ( -12.57512233279243574, -101.1416252791420476, -9.133129954655776928 ) ) ;
#11223=CARTESIAN_POINT ( 'NONE',  ( 0.9302366604389999960, -100.4808658609999981, -16.19480876779999790 ) ) ;
#11224=CARTESIAN_POINT ( 'NONE',  ( 2.876553231629999985, -91.50000000000000000, 5.265495371340000119 ) ) ;
#11225=LINE ( 'NONE', #11822, #18230 ) ;
#11228=DIRECTION ( 'NONE',  ( 0.2162432783070565578, 0.000000000000000000, 0.9763395129702663322 ) ) ;
#11234=CARTESIAN_POINT ( 'NONE',  ( 14.95019707169999990, -101.2530993000000024, 2.710463435110000319 ) ) ;
#11235=B_SPLINE_CURVE_WITH_KNOTS ( 'NONE', 3,
 ( #18402, #16348, #20882, #27290 ),
 .UNSPECIFIED., .F., .F.,
 ( 4, 4 ),
 ( -19.56549066489999689, -15.82800233080000041 ),
 .UNSPECIFIED. ) ;
#11236=CARTESIAN_POINT ( 'NONE',  ( 14.95034095350000136, -97.23151611000000116, 15.27375035569999895 ) ) ;
#11238=CARTESIAN_POINT ( 'NONE',  ( 23.52525244343676647, -92.58347372263170882, -19.41166030436781043 ) ) ;
#11239=CARTESIAN_POINT ( 'NONE',  ( 22.57257117529999846, -92.75885938649999218, 15.68540759639999749 ) ) ;
#11242=CARTESIAN_POINT ( 'NONE',  ( -7.423820152569999387, -100.9678331089999972, 14.37793136710000041 ) ) ;
#11243=VERTEX_POINT ( 'NONE', #28368 ) ;
#11245=ORIENTED_EDGE ( 'NONE', *, *, #17406, .T. ) ;
#11251=DIRECTION ( 'NONE',  ( 0.000000000000000000, 1.000000000000000000, 0.000000000000000000 ) ) ;
#11253=CARTESIAN_POINT ( 'NONE',  ( -15.21246199350000161, -100.9405350259999921, 4.776674228709999248 ) ) ;
#11256=CARTESIAN_POINT ( 'NONE',  ( 13.20594032278986774, -96.16332745752187350, 17.30516087073727505 ) ) ;
#11266=ORIENTED_EDGE ( 'NONE', *, *, #14787, .F. ) ;
#11273=CARTESIAN_POINT ( 'NONE',  ( 0.000000000000000000, -108.5000000000000000, 0.000000000000000000 ) ) ;
#11278=ORIENTED_EDGE ( 'NONE', *, *, #130, .T. ) ;
#11281=CARTESIAN_POINT ( 'NONE',  ( -19.66462998450000299, -97.01506441399999403, -6.707659482730000455 ) ) ;
#11283=CARTESIAN_POINT ( 'NONE',  ( -30.47783378272416854, -92.54687141712493315, 1.162627035193506853 ) ) ;
#11289=CARTESIAN_POINT ( 'NONE',  ( 22.85992316819999814, -94.54719310899999130, -6.820851015779999749 ) ) ;
#11292=CARTESIAN_POINT ( 'NONE',  ( 14.06911839400000019, -98.73889367950000917, -12.22485475130000054 ) ) ;
#11293=ORIENTED_EDGE ( 'NONE', *, *, #4317, .F. ) ;
#11294=AXIS2_PLACEMENT_3D ( 'NONE', #18628, #15840, #1020 ) ;
#11297=CARTESIAN_POINT ( 'NONE',  ( -12.90942923769999950, -100.2522625769999962, -11.08739780120000162 ) ) ;
#11305=ORIENTED_EDGE ( 'NONE', *, *, #10551, .T. ) ;
#11306=EDGE_CURVE ( 'NONE', #22763, #2020, #88, .T. ) ;
#11309=VECTOR ( 'NONE', #12681, 1000.000000000000114 ) ;
#11311=CARTESIAN_POINT ( 'NONE',  ( 12.03509228579999935, -92.84019744260001517, 27.58265792150000095 ) ) ;
#11312=VERTEX_POINT ( 'NONE', #21967 ) ;
#11315=CARTESIAN_POINT ( 'NONE',  ( 20.33590001279999981, -94.16310024840001347, 13.51329393089999975 ) ) ;
#11323=CARTESIAN_POINT ( 'NONE',  ( -23.85440626824976107, -94.57749869815765464, -4.067369308893817426 ) ) ;
#11324=ORIENTED_EDGE ( 'NONE', *, *, #7382, .F. ) ;
#11325=CARTESIAN_POINT ( 'NONE',  ( 6.981684465299999864, -93.00000000000000000, 29.03810821740000137 ) ) ;
#11326=CIRCLE ( 'NONE', #19715, 5.000000000000000888 ) ;
#11327=CARTESIAN_POINT ( 'NONE',  ( 13.88148934900000064, -99.91102932019998661, -9.687780287520000755 ) ) ;
#11336=EDGE_CURVE ( 'NONE', #25460, #3543, #23396, .T. ) ;
#11340=CARTESIAN_POINT ( 'NONE',  ( -24.20176002190990516, -92.56772982775143532, -18.56148008688876416 ) ) ;
#11344=EDGE_CURVE ( 'NONE', #11758, #19059, #20616, .T. ) ;
#11349=CARTESIAN_POINT ( 'NONE',  ( 17.45802118700000349, -99.55619081819999394, 0.9170739917250000373 ) ) ;
#11352=CARTESIAN_POINT ( 'NONE',  ( -2.903039748510000351, -94.98812477769999418, 23.52859306979999943 ) ) ;
#11355=CARTESIAN_POINT ( 'NONE',  ( 3.631617597942636166, -93.11247489620001261, -28.67783563263252589 ) ) ;
#11356=DIRECTION ( 'NONE',  ( 0.000000000000000000, 1.000000000000000000, 0.000000000000000000 ) ) ;
#11364=CARTESIAN_POINT ( 'NONE',  ( -13.31491859036868775, -92.89593097429161617, 27.44017123060003627 ) ) ;
#11368=CARTESIAN_POINT ( 'NONE',  ( -17.05574026919999753, -93.34713166629998682, 21.78488634390000200 ) ) ;
#11372=CARTESIAN_POINT ( 'NONE',  ( -16.22299306009999853, -99.56341898720000927, 6.708263584790000067 ) ) ;
#11374=CARTESIAN_POINT ( 'NONE',  ( 0.6180977789570000214, -100.8746138070000029, -16.59152119279999837 ) ) ;
#11378=ADVANCED_FACE ( 'NONE', ( #19043 ), #3789, .T. ) ;
#11381=CARTESIAN_POINT ( 'NONE',  ( -15.60988350939999947, -92.64731536089999508, 23.37060113569999942 ) ) ;
#11382=DIRECTION ( 'NONE',  ( 0.000000000000000000, -1.000000000000000000, 0.000000000000000000 ) ) ;
#11387=CARTESIAN_POINT ( 'NONE',  ( -18.84946550835717005, -97.93129752234466423, 6.692286737796515617 ) ) ;
#11388=B_SPLINE_CURVE_WITH_KNOTS ( 'NONE', 5,
 ( #14411, #21123, #9601, #18653, #2922, #25212, #14540, #11785, #25489 ),
 .UNSPECIFIED., .F., .F.,
 ( 6, 3, 6 ),
 ( 0.000000000000000000, 0.5000000000000000000, 1.000000000000000000 ),
 .UNSPECIFIED. ) ;
#11389=CARTESIAN_POINT ( 'NONE',  ( 11.31179088046036441, -98.73470581857429806, -14.63453564218954739 ) ) ;
#11390=CARTESIAN_POINT ( 'NONE',  ( -7.341283001269998998, -101.1412505549999992, 14.40471526709999850 ) ) ;
#11396=CARTESIAN_POINT ( 'NONE',  ( 7.560313589829999792, -99.58327329889999646, 15.94543460589999739 ) ) ;
#11397=CARTESIAN_POINT ( 'NONE',  ( 3.166345171159999694, -93.00000000000000000, -25.30265318609999881 ) ) ;
#11398=CARTESIAN_POINT ( 'NONE',  ( -3.841450593410000280, -96.73974214389998849, -20.89652819670000028 ) ) ;
#11400=ORIENTED_EDGE ( 'NONE', *, *, #6076, .T. ) ;
#11401=CARTESIAN_POINT ( 'NONE',  ( -14.79537254420000103, -100.9197086940000077, 5.022279801499999863 ) ) ;
#11408=CARTESIAN_POINT ( 'NONE',  ( 24.71840331404647628, -93.41743724424139828, -12.20012907774811062 ) ) ;
#11409=CARTESIAN_POINT ( 'NONE',  ( 29.52540673129999860, -93.00000000000000000, 7.168153169610000930 ) ) ;
#11412=CARTESIAN_POINT ( 'NONE',  ( 8.085424419389999784, -101.4206919209999853, 14.00535675889999965 ) ) ;
#11425=CARTESIAN_POINT ( 'NONE',  ( -17.51014701730000311, -98.29702512480000109, -7.640698720650000553 ) ) ;
#11427=CARTESIAN_POINT ( 'NONE',  ( -30.47866716000020659, -92.54383083955178790, 1.140710722936425281 ) ) ;
#11428=CARTESIAN_POINT ( 'NONE',  ( -17.00715350810000004, -99.92967601899998442, 3.484608414699999823 ) ) ;
#11429=CARTESIAN_POINT ( 'NONE',  ( -17.00715350810000004, -101.1889999979999999, 3.484608414699999823 ) ) ;
#11433=CARTESIAN_POINT ( 'NONE',  ( 12.77500156440000012, -93.00000000000000000, 27.05403395929999988 ) ) ;
#11436=CARTESIAN_POINT ( 'NONE',  ( -15.18759500087176306, -100.4790389224915401, 5.637615933027189108 ) ) ;
#11437=VERTEX_POINT ( 'NONE', #15501 ) ;
#11439=CARTESIAN_POINT ( 'NONE',  ( -5.119737544835406773, -100.1470170834167419, 17.03205665007207159 ) ) ;
#11441=DIRECTION ( 'NONE',  ( 1.000000000000000000, 0.000000000000000000, 0.000000000000000000 ) ) ;
#11449=CARTESIAN_POINT ( 'NONE',  ( -4.056245258659999742, -98.60488091210000050, 19.31197723180000025 ) ) ;
#11450=CARTESIAN_POINT ( 'NONE',  ( 7.994999523870000679, -92.89940159850000612, 27.27230444749999805 ) ) ;
#11461=B_SPLINE_CURVE_WITH_KNOTS ( 'NONE', 3,
 ( #19583, #17412, #19308, #28054, #17115, #24103, #10525, #21923, #21353, #8357, #1410, #10255, #17259, #10818, #6326, #4140, #24398, #15637, #11408, #16080, #380, #26741, #7070, #10955, #22073, #28746, #18283, #24537, #6776, #27173, #4291, #17844, #27028, #7211, #9378, #13457, #20308 ),
 .UNSPECIFIED., .F., .F.,
 ( 4, 2, 2, 1, 1, 1, 2, 2, 2, 2, 1, 1, 1, 2, 2, 2, 2, 1, 1, 1, 2, 2, 4 ),
 ( 0.000000000000000000, 0.1250000000000197065, 0.1875000000000296707, 0.2187500000000343614, 0.2343750000000362488, 0.2421875000000367484, 0.2460937500000368872, 0.2500000000000370259, 0.3750000000000243694, 0.4375000000000178746, 0.4687500000000144329, 0.4843750000000129896, 0.4921875000000123235, 0.4960937500000122125, 0.5000000000000121014, 0.6250000000000108802, 0.6875000000000104361, 0.7187500000000101030, 0.7343750000000097700, 0.7421875000000094369, 0.7460937500000092149, 0.7500000000000091038, 1.000000000000000000 ),
 .UNSPECIFIED. ) ;
#11462=CARTESIAN_POINT ( 'NONE',  ( 12.32527298249999959, -101.3256027139999986, -10.05536332369999997 ) ) ;
#11463=ADVANCED_FACE ( 'NONE', ( #24116 ), #13556, .F. ) ;
#11464=CARTESIAN_POINT ( 'NONE',  ( -12.47731372630000024, -94.18458606750000683, -20.89673554119999821 ) ) ;
#11477=CARTESIAN_POINT ( 'NONE',  ( 0.000000000000000000, -102.8486084350000027, 0.000000000000000000 ) ) ;
#11480=CARTESIAN_POINT ( 'NONE',  ( 16.13476677959289418, -100.7538407667569658, 4.305120634646285360 ) ) ;
#11492=ORIENTED_EDGE ( 'NONE', *, *, #4237, .F. ) ;
#11494=CARTESIAN_POINT ( 'NONE',  ( 9.385332722619999402, -98.68450614990000247, 16.47661810339999988 ) ) ;
#11498=EDGE_CURVE ( 'NONE', #7420, #5746, #10733, .T. ) ;
#11500=CARTESIAN_POINT ( 'NONE',  ( 7.834729293268852146, -94.01603309712585599, -24.85338230034197693 ) ) ;
#11501=CARTESIAN_POINT ( 'NONE',  ( -28.46472064010000125, -92.56290624670000966, 3.501361395690000045 ) ) ;
#11502=CARTESIAN_POINT ( 'NONE',  ( -20.03691699049999997, -95.66927305889998934, 10.25834442809999913 ) ) ;
#11507=EDGE_CURVE ( 'NONE', #5924, #18376, #7533, .T. ) ;
#11510=CARTESIAN_POINT ( 'NONE',  ( -12.71070678442828772, -92.56772982770620217, 27.72528925393579868 ) ) ;
#11522=CARTESIAN_POINT ( 'NONE',  ( -6.781378104809999030, -111.0000000000000000, 14.49182221120000058 ) ) ;
#11523=TOROIDAL_SURFACE ( 'NONE', #18995, 15.50000000000000000, 0.5000000000000000000 ) ;
#11525=B_SPLINE_CURVE_WITH_KNOTS ( 'NONE', 5,
 ( #21228, #10406, #5905, #10124, #23553, #23687, #21097, #12592, #7702 ),
 .UNSPECIFIED., .F., .F.,
 ( 6, 3, 6 ),
 ( 0.000000000000000000, 0.5000000000000000000, 1.000000000000000000 ),
 .UNSPECIFIED. ) ;
#11529=CARTESIAN_POINT ( 'NONE',  ( 8.140396429159999059, -100.8869814400000138, 13.38618259969999968 ) ) ;
#11541=VERTEX_POINT ( 'NONE', #1623 ) ;
#11542=ADVANCED_FACE ( 'NONE', ( #1485 ), #27984, .T. ) ;
#11543=CARTESIAN_POINT ( 'NONE',  ( 6.888450598059999486, -99.53431388120000634, 15.99365471700000008 ) ) ;
#11546=CARTESIAN_POINT ( 'NONE',  ( 0.000000000000000000, -101.6484611540000031, 0.000000000000000000 ) ) ;
#11548=CARTESIAN_POINT ( 'NONE',  ( 11.86312790959999930, -101.5317765570000006, -10.86703365620000028 ) ) ;
#11550=CARTESIAN_POINT ( 'NONE',  ( 13.81470970028357215, -95.86012411014323220, 17.32825506473149701 ) ) ;
#11554=DIRECTION ( 'NONE',  ( 0.000000000000000000, -1.000000000000000000, 0.000000000000000000 ) ) ;
#11556=VERTEX_POINT ( 'NONE', #14847 ) ;
#11564=CARTESIAN_POINT ( 'NONE',  ( -14.54628291358669046, -94.01603309693408050, -21.62126842404864746 ) ) ;
#11571=CARTESIAN_POINT ( 'NONE',  ( -21.78729678839999906, -95.70830610310001418, -5.566096626759999388 ) ) ;
#11572=ORIENTED_EDGE ( 'NONE', *, *, #327, .T. ) ;
#11573=CARTESIAN_POINT ( 'NONE',  ( 9.457795928940385011, -92.92035259857971141, 28.99786150557102715 ) ) ;
#11574=CIRCLE ( 'NONE', #26264, 18.64285714289999873 ) ;
#11583=CARTESIAN_POINT ( 'NONE',  ( -17.08506256729766193, -97.54019988239669203, 10.37759590189724790 ) ) ;
#11584=ORIENTED_EDGE ( 'NONE', *, *, #13776, .F. ) ;
#11586=CARTESIAN_POINT ( 'NONE',  ( 0.000000000000000000, -92.50000000000000000, 0.000000000000000000 ) ) ;
#11587=CARTESIAN_POINT ( 'NONE',  ( 7.830640929019831553, -101.5867234369360403, 14.00591651322954689 ) ) ;
#11589=CARTESIAN_POINT ( 'NONE',  ( 0.000000000000000000, -92.50000000000000000, 0.000000000000000000 ) ) ;
#11593=CARTESIAN_POINT ( 'NONE',  ( 26.95513443413419452, -92.54687141712491893, -14.27132724549746534 ) ) ;
#11596=CIRCLE ( 'NONE', #15299, 0.4999999999999986122 ) ;
#11598=CARTESIAN_POINT ( 'NONE',  ( 1.312652382290000030, -94.71481430560001513, 24.32357623499999733 ) ) ;
#11599=CARTESIAN_POINT ( 'NONE',  ( 4.103525764680000520, -93.31218863639999483, 25.66466408690000023 ) ) ;
#11609=CARTESIAN_POINT ( 'NONE',  ( 7.584268347236687191, -101.5555611381076204, 14.08825305945834394 ) ) ;
#11617=CARTESIAN_POINT ( 'NONE',  ( -16.89322606969999896, -99.75798417260000406, 3.074878952570000212 ) ) ;
#11620=CARTESIAN_POINT ( 'NONE',  ( 15.14880929390000119, -101.6484611540000031, 3.280789078519999791 ) ) ;
#11622=FACE_OUTER_BOUND ( 'NONE', #14917, .T. ) ;
#11624=EDGE_CURVE ( 'NONE', #24455, #4274, #20566, .T. ) ;
#11628=CARTESIAN_POINT ( 'NONE',  ( 16.22618840215064395, -100.6338045034763979, 4.332579364030344493 ) ) ;
#11639=CIRCLE ( 'NONE', #27015, 29.91857981989999971 ) ;
#11651=CARTESIAN_POINT ( 'NONE',  ( -7.333297298759998917, -94.59276292389999696, -22.63874378639999563 ) ) ;
#11656=DIRECTION ( 'NONE',  ( 1.000000000000000000, 0.000000000000000000, 0.000000000000000000 ) ) ;
#11657=CARTESIAN_POINT ( 'NONE',  ( -13.01302628178067700, -92.66191076874173405, 27.58469122193175949 ) ) ;
#11659=B_SPLINE_CURVE_WITH_KNOTS ( 'NONE', 5,
 ( #4964, #23049, #7610, #22752, #12088, #9901 ),
 .UNSPECIFIED., .F., .F.,
 ( 6, 6 ),
 ( 0.000000000000000000, 1.000000000000000000 ),
 .UNSPECIFIED. ) ;
#11662=DIRECTION ( 'NONE',  ( 0.000000000000000000, 1.000000000000000000, 0.000000000000000000 ) ) ;
#11665=CARTESIAN_POINT ( 'NONE',  ( -18.04416748670000459, -95.71113290489999770, 13.55963794960000079 ) ) ;
#11666=TOROIDAL_SURFACE ( 'NONE', #15867, 29.91857981989999971, 10.00000000000000000 ) ;
#11670=EDGE_CURVE ( 'NONE', #9243, #14226, #15726, .T. ) ;
#11677=CARTESIAN_POINT ( 'NONE',  ( -0.1689899845689999958, -101.2530993010000060, -15.19297360289999865 ) ) ;
#11678=CARTESIAN_POINT ( 'NONE',  ( 10.18609790949999905, -99.75094907060000082, 14.67385898429999891 ) ) ;
#11679=VERTEX_POINT ( 'NONE', #25063 ) ;
#11680=CIRCLE ( 'NONE', #15378, 18.64285714289999873 ) ;
#11684=TOROIDAL_SURFACE ( 'NONE', #25216, 21.14285714289999873, 0.5000000000000000000 ) ;
#11686=CARTESIAN_POINT ( 'NONE',  ( -7.417318425790000447, -100.8455998110000138, 14.22575192579999914 ) ) ;
#11690=CARTESIAN_POINT ( 'NONE',  ( 7.405704750090000843, -101.1273033739999931, 13.62605079230000094 ) ) ;
#11691=ORIENTED_EDGE ( 'NONE', *, *, #16529, .F. ) ;
#11694=CARTESIAN_POINT ( 'NONE',  ( 0.6456114843440000639, -99.57787118740000665, -17.34593263700000421 ) ) ;
#11697=CARTESIAN_POINT ( 'NONE',  ( 11.32586188939999872, -100.9728541479999961, -10.72774646679999933 ) ) ;
#11699=CARTESIAN_POINT ( 'NONE',  ( 15.40147643716055015, -95.08513980200086735, 17.29809606948850131 ) ) ;
#11704=CARTESIAN_POINT ( 'NONE',  ( -16.77201711099999670, -99.85760268239999959, 2.755376769609999776 ) ) ;
#11708=ADVANCED_FACE ( 'NONE', ( #3584 ), #5097, .F. ) ;
#11710=FACE_OUTER_BOUND ( 'NONE', #10851, .T. ) ;
#11713=CARTESIAN_POINT ( 'NONE',  ( 23.56050396080000198, -94.79581469870001342, -2.314010422780000464 ) ) ;
#11718=DIRECTION ( 'NONE',  ( 0.000000000000000000, -1.000000000000000000, 0.000000000000000000 ) ) ;
#11719=CARTESIAN_POINT ( 'NONE',  ( -18.72457341818005006, -96.53847999818908932, -10.28520624310983678 ) ) ;
#11720=CIRCLE ( 'NONE', #21501, 0.7500000000000006661 ) ;
#11721=DIRECTION ( 'NONE',  ( 0.000000000000000000, 1.000000000000000000, 0.000000000000000000 ) ) ;
#11724=LINE ( 'NONE', #7375, #16163 ) ;
#11725=CARTESIAN_POINT ( 'NONE',  ( -22.20135144879999700, -95.98460637919998817, -5.903444897400000002 ) ) ;
#11728=CARTESIAN_POINT ( 'NONE',  ( 9.093840868627895091, -92.81370807120056554, 29.11275331569328273 ) ) ;
#11736=B_SPLINE_SURFACE_WITH_KNOTS ( 'NONE', 5, 5, ( 
 ( #23492, #7640, #19115, #16507, #8040, #25405 ),
 ( #12390, #10200, #3123, #20748, #807, #5433 ),
 ( #14727, #8592, #26091, #3807, #23906, #24194 ),
 ( #5843, #17494, #23624, #3664, #8173, #19251 ),
 ( #10337, #28410, #22014, #10473, #8726, #3943 ),
 ( #8302, #12807, #28556, #6120, #4225, #19667 ) ),
 .UNSPECIFIED., .F., .F., .F.,
 ( 6, 6 ),
 ( 6, 6 ),
 ( 7.179549394140000373, 14.35382494800000153 ),
 ( 0.000000000000000000, 0.5000000000000000000 ),
 .UNSPECIFIED. ) ;
#11737=ORIENTED_EDGE ( 'NONE', *, *, #18475, .T. ) ;
#11742=CARTESIAN_POINT ( 'NONE',  ( 15.67492025179999970, -101.0314399550000104, 2.383182498780000103 ) ) ;
#11743=ORIENTED_EDGE ( 'NONE', *, *, #4581, .F. ) ;
#11744=EDGE_CURVE ( 'NONE', #3132, #21723, #447, .T. ) ;
#11745=TOROIDAL_SURFACE ( 'NONE', #28038, 18.14285714289999873, 0.5000000000000000000 ) ;
#11746=CIRCLE ( 'NONE', #14984, 16.00000000000000000 ) ;
#11751=CARTESIAN_POINT ( 'NONE',  ( -0.4238013828789999882, -95.77248565759998655, 22.35470455460000139 ) ) ;
#11752=CARTESIAN_POINT ( 'NONE',  ( 5.659366841679999816, -92.97642175670000597, 26.32172450590000068 ) ) ;
#11755=CARTESIAN_POINT ( 'NONE',  ( -25.90513195527891099, -94.04667188315717397, -2.194660316649619691 ) ) ;
#11756=CARTESIAN_POINT ( 'NONE',  ( -12.50340864429999854, -94.22763312360000043, -20.80754938939999832 ) ) ;
#11757=CARTESIAN_POINT ( 'NONE',  ( 2.356750984242918623, -93.20709273738651746, 27.37396933629507600 ) ) ;
#11758=VERTEX_POINT ( 'NONE', #12315 ) ;
#11761=CARTESIAN_POINT ( 'NONE',  ( -8.841108207830000509, -95.92024868639998658, -20.36834459239999973 ) ) ;
#11769=ORIENTED_EDGE ( 'NONE', *, *, #25740, .F. ) ;
#11771=CARTESIAN_POINT ( 'NONE',  ( -16.14211878319999727, -101.0779259520000011, 3.133147776259999961 ) ) ;
#11777=CARTESIAN_POINT ( 'NONE',  ( 23.76596721370000154, -92.50425969839999141, -17.55797138329999640 ) ) ;
#11778=ORIENTED_EDGE ( 'NONE', *, *, #327, .F. ) ;
#11779=CARTESIAN_POINT ( 'NONE',  ( 0.3059185938709999553, -111.0000000000000000, 14.72672055670000013 ) ) ;
#11784=CARTESIAN_POINT ( 'NONE',  ( 16.41212907226823248, -100.4010812937642214, 4.355947949365128302 ) ) ;
#11785=CARTESIAN_POINT ( 'NONE',  ( 19.94074090517771225, -94.89420224093041156, 14.19047658555035518 ) ) ;
#11792=LINE ( 'NONE', #3082, #8883 ) ;
#11800=CARTESIAN_POINT ( 'NONE',  ( -18.05095464379880354, -92.86910234287326205, -23.30076470957695634 ) ) ;
#11807=CARTESIAN_POINT ( 'NONE',  ( -3.633282526024673054, -96.53847999809016756, -21.05218219683358072 ) ) ;
#11812=DIRECTION ( 'NONE',  ( 1.000000000000000000, 0.000000000000000000, 0.000000000000000000 ) ) ;
#11816=CARTESIAN_POINT ( 'NONE',  ( -12.59499905819999910, -101.4254868729999970, -9.817004629319999509 ) ) ;
#11819=CARTESIAN_POINT ( 'NONE',  ( -17.16832732159999964, -98.24896744320000153, 8.807259461759999297 ) ) ;
#11822=CARTESIAN_POINT ( 'NONE',  ( 2.876553231629999985, -100.0000000000000000, 5.265495371340000119 ) ) ;
#11829=CARTESIAN_POINT ( 'NONE',  ( 17.39024827180000088, -95.90105875090000609, 14.90673015379999988 ) ) ;
#11831=AXIS2_PLACEMENT_3D ( 'NONE', #3281, #824, #16376 ) ;
#11833=CARTESIAN_POINT ( 'NONE',  ( 16.49890011909999643, -94.79581646409999962, 16.97758076400000249 ) ) ;
#11836=CARTESIAN_POINT ( 'NONE',  ( -7.940795358099999923, -100.3063911739999980, 15.09437935239999895 ) ) ;
#11838=CARTESIAN_POINT ( 'NONE',  ( -10.31966890614535082, -93.93488429366382775, -23.20916244078144075 ) ) ;
#11846=CARTESIAN_POINT ( 'NONE',  ( 11.56323489949999939, -97.41042626769998947, -18.07474074250000129 ) ) ;
#11848=CIRCLE ( 'NONE', #2081, 30.50000000000000000 ) ;
#11851=DIRECTION ( 'NONE',  ( 0.000000000000000000, 1.000000000000000000, 0.000000000000000000 ) ) ;
#11853=CARTESIAN_POINT ( 'NONE',  ( 15.97618948326800314, -94.80901416784320190, 17.25790605317358484 ) ) ;
#11854=EDGE_CURVE ( 'NONE', #22747, #12473, #6464, .T. ) ;
#11855=CARTESIAN_POINT ( 'NONE',  ( -25.37284092810000047, -92.50000000000000000, 2.543411731580000001 ) ) ;
#11858=CARTESIAN_POINT ( 'NONE',  ( -6.665307709260000379, -101.1889999979999999, -13.13558364449999871 ) ) ;
#11862=CARTESIAN_POINT ( 'NONE',  ( 13.85716626522326322, -97.34036579237553610, -15.36281561190910949 ) ) ;
#11869=CARTESIAN_POINT ( 'NONE',  ( 21.75659477429999811, -101.1889999979999999, -13.30039788230000042 ) ) ;
#11870=CARTESIAN_POINT ( 'NONE',  ( -11.32307664130000013, -93.00000000000000000, 9.421136869679999748 ) ) ;
#11874=CARTESIAN_POINT ( 'NONE',  ( -20.20541094980000096, -94.98812148390000232, 12.40015412250000004 ) ) ;
#11876=CARTESIAN_POINT ( 'NONE',  ( -30.44632542846705192, -92.66777315148624439, 1.808678671120149462 ) ) ;
#11878=CARTESIAN_POINT ( 'NONE',  ( 0.4337523258651289626, -101.2637735886937094, -16.29242920662442984 ) ) ;
#11880=CARTESIAN_POINT ( 'NONE',  ( -11.69640386740000082, -101.0875971110000080, -10.03173011250000002 ) ) ;
#11881=B_SPLINE_CURVE_WITH_KNOTS ( 'NONE', 5,
 ( #21207, #5747, #25859, #12156, #14762, #1129, #988, #25440, #16970 ),
 .UNSPECIFIED., .F., .F.,
 ( 6, 3, 6 ),
 ( 0.000000000000000000, 0.5000000000000000000, 1.000000000000000000 ),
 .UNSPECIFIED. ) ;
#11882=CARTESIAN_POINT ( 'NONE',  ( 23.54490914119999800, -94.22485739640001157, -7.400599509700000134 ) ) ;
#11883=ADVANCED_FACE ( 'NONE', ( #14377 ), #3313, .F. ) ;
#11891=FACE_OUTER_BOUND ( 'NONE', #2550, .T. ) ;
#11895=DIRECTION ( 'NONE',  ( -0.8737996304181506746, 0.000000000000000000, 0.4862861358100837861 ) ) ;
#11897=CARTESIAN_POINT ( 'NONE',  ( -13.18661228299999877, -93.00000000000000000, 26.85581268440000002 ) ) ;
#11898=CARTESIAN_POINT ( 'NONE',  ( 1.342731302320000264, -94.57749190790001137, 24.16139931020000020 ) ) ;
#11899=VERTEX_POINT ( 'NONE', #15188 ) ;
#11901=B_SPLINE_CURVE_WITH_KNOTS ( 'NONE', 3,
 ( #18298, #8681, #2161, #2711, #17599, #6524, #26200, #17748, #11564, #27185, #7228, #5028, #12903, #21820, #10713, #19628, #8552, #17455, #26340, #6366, #22816, #20634, #23107, #1125, #1255, #7532, #25436, #5606, #5329, #18736, #9542, #16540, #14219, #18878, #9827, #12292, #27632 ),
 .UNSPECIFIED., .F., .F.,
 ( 4, 2, 2, 1, 1, 1, 2, 2, 2, 2, 1, 1, 1, 2, 2, 2, 2, 1, 1, 1, 2, 2, 4 ),
 ( 0.000000000000000000, 0.1249999999999938105, 0.1874999999999909239, 0.2187499999999897859, 0.2343749999999894529, 0.2421874999999897304, 0.2460937499999898692, 0.2499999999999900080, 0.3750000000000081046, 0.4375000000000174305, 0.4687500000000217604, 0.4843750000000236478, 0.4921875000000245914, 0.4960937500000250355, 0.5000000000000255351, 0.6250000000000371925, 0.6875000000000431877, 0.7187500000000457412, 0.7343750000000467404, 0.7421875000000471845, 0.7460937500000471845, 0.7500000000000471845, 1.000000000000000000 ),
 .UNSPECIFIED. ) ;
#11905=CARTESIAN_POINT ( 'NONE',  ( -2.415535008216042723, -94.65677004888377155, 24.01682572601766807 ) ) ;
#11907=CARTESIAN_POINT ( 'NONE',  ( 26.02259374959999860, -111.0000000000000000, -15.90831903569999994 ) ) ;
#11909=VERTEX_POINT ( 'NONE', #10821 ) ;
#11917=ADVANCED_FACE ( 'NONE', ( #15491 ), #28321, .F. ) ;
#11919=CARTESIAN_POINT ( 'NONE',  ( -15.97429264209999999, -100.8622054559999981, 3.109706331429999970 ) ) ;
#11923=CARTESIAN_POINT ( 'NONE',  ( -14.42556421679999978, -93.00000000000000000, -2.978755036369999942 ) ) ;
#11932=ORIENTED_EDGE ( 'NONE', *, *, #3117, .F. ) ;
#11940=CARTESIAN_POINT ( 'NONE',  ( -5.390284282690000595, -100.8869817940000075, 14.71056662440000018 ) ) ;
#11942=CARTESIAN_POINT ( 'NONE',  ( -18.05096283909999855, -93.00000167610001256, -23.30076369320000040 ) ) ;
#11943=DIRECTION ( 'NONE',  ( 1.000000000000000000, 0.000000000000000000, 0.000000000000000000 ) ) ;
#11947=CARTESIAN_POINT ( 'NONE',  ( 22.85993575921586896, -94.54719627003775884, -6.820847890398427538 ) ) ;
#11948=DIRECTION ( 'NONE',  ( 0.000000000000000000, 1.000000000000000000, 0.000000000000000000 ) ) ;
#11950=ORIENTED_EDGE ( 'NONE', *, *, #26589, .F. ) ;
#11952=CARTESIAN_POINT ( 'NONE',  ( 19.83740677649999640, -97.64874574840000321, 2.314389350519999944 ) ) ;
#11954=CARTESIAN_POINT ( 'NONE',  ( -12.16265938883512376, -92.50000000000000000, 27.97031705946124802 ) ) ;
#11959=ORIENTED_EDGE ( 'NONE', *, *, #25763, .F. ) ;
#11960=CARTESIAN_POINT ( 'NONE',  ( -17.54428790840000119, -94.59276292389999696, 16.07756064530000017 ) ) ;
#11973=CARTESIAN_POINT ( 'NONE',  ( -13.31136913029999924, -101.0685849509999912, -9.042834681369999572 ) ) ;
#11975=B_SPLINE_SURFACE_WITH_KNOTS ( 'NONE', 5, 5, ( 
 ( #34, #22464, #20266, #22612, #335, #19816 ),
 ( #18083, #28694, #26532, #15281, #7020, #4833 ),
 ( #26686, #4389, #13711, #2656, #15437, #13258 ),
 ( #20415, #22165, #8882, #485, #2205, #17795 ),
 ( #6727, #24492, #20567, #16035, #5410, #18527 ),
 ( #27417, #24940, #7615, #14293, #633, #4969 ) ),
 .UNSPECIFIED., .F., .F., .F.,
 ( 6, 6 ),
 ( 6, 6 ),
 ( 7.179431122730000503, 23.44689954309999891 ),
 ( 0.000000000000000000, 0.5000000000000000000 ),
 .UNSPECIFIED. ) ;
#11976=DIRECTION ( 'NONE',  ( 0.000000000000000000, 1.000000000000000000, 0.000000000000000000 ) ) ;
#11977=CARTESIAN_POINT ( 'NONE',  ( -7.630334818519999729, -100.8023006570000035, 13.80849637110000039 ) ) ;
#11980=CARTESIAN_POINT ( 'NONE',  ( 7.474780311509999109, -101.1715078010000042, 13.84506678670000035 ) ) ;
#11981=VERTEX_POINT ( 'NONE', #20170 ) ;
#11986=EDGE_LOOP ( 'NONE', ( #17946, #8738, #10862, #22597 ) ) ;
#11992=B_SPLINE_CURVE_WITH_KNOTS ( 'NONE', 3,
 ( #3370, #16904, #14433, #23190, #25794, #5823, #1471, #14705, #23470, #3510, #14156, #23324 ),
 .UNSPECIFIED., .F., .F.,
 ( 4, 2, 2, 2, 2, 4 ),
 ( 0.000000000000000000, 0.2499999999999840128, 0.3749999999999876210, 0.4374999999999744649, 0.4999999999999613087, 1.000000000000000000 ),
 .UNSPECIFIED. ) ;
#11996=ORIENTED_EDGE ( 'NONE', *, *, #20104, .T. ) ;
#11998=CARTESIAN_POINT ( 'NONE',  ( 6.390838521760000113, -101.2010924020000004, 13.85940160760000062 ) ) ;
#12000=CARTESIAN_POINT ( 'NONE',  ( 7.610177731959999470, -101.4231532209999926, 14.04048934709999941 ) ) ;
#12002=CARTESIAN_POINT ( 'NONE',  ( -11.58382158670000095, -95.11335285699999531, -21.40443484560000087 ) ) ;
#12006=EDGE_CURVE ( 'NONE', #17308, #21862, #18600, .T. ) ;
#12010=DIRECTION ( 'NONE',  ( 0.000000000000000000, -1.000000000000000000, 0.000000000000000000 ) ) ;
#12012=CARTESIAN_POINT ( 'NONE',  ( -5.298192075760000286, -100.9197081840000010, 14.69882727599999939 ) ) ;
#12013=ORIENTED_EDGE ( 'NONE', *, *, #16364, .T. ) ;
#12015=CARTESIAN_POINT ( 'NONE',  ( 0.5547406113394584004, -100.2392017794624053, -17.10134437667061036 ) ) ;
#12020=AXIS2_PLACEMENT_3D ( 'NONE', #16234, #22373, #2419 ) ;
#12022=CARTESIAN_POINT ( 'NONE',  ( 12.88056774689999884, -94.79581469870001342, -19.86310563940000051 ) ) ;
#12028=DIRECTION ( 'NONE',  ( 0.000000000000000000, 1.000000000000000000, 0.000000000000000000 ) ) ;
#12030=EDGE_CURVE ( 'NONE', #7500, #8693, #4219, .T. ) ;
#12033=AXIS2_PLACEMENT_3D ( 'NONE', #17752, #8555, #26634 ) ;
#12035=CARTESIAN_POINT ( 'NONE',  ( -2.607841079019999952, -97.32097376469998551, 21.26526383349999705 ) ) ;
#12036=CARTESIAN_POINT ( 'NONE',  ( 11.26796299709999971, -92.84764728559999014, 27.58759766900000088 ) ) ;
#12040=CARTESIAN_POINT ( 'NONE',  ( -11.16205695805461495, -94.83055549493140290, -21.09956338124505137 ) ) ;
#12045=CARTESIAN_POINT ( 'NONE',  ( 6.153546133999999945, -93.00000450890000536, 28.82528558229999760 ) ) ;
#12055=CARTESIAN_POINT ( 'NONE',  ( -15.86504038540000039, -100.9725757459999897, 3.161101131529999719 ) ) ;
#12059=DIRECTION ( 'NONE',  ( 0.000000000000000000, 1.000000000000000000, 0.000000000000000000 ) ) ;
#12061=CARTESIAN_POINT ( 'NONE',  ( 22.78264860270000014, -94.59276292389999696, -6.873201011689999085 ) ) ;
#12069=CARTESIAN_POINT ( 'NONE',  ( 15.82576138244594333, -101.2021794473940162, 4.092296143312620593 ) ) ;
#12072=EDGE_CURVE ( 'NONE', #22989, #24255, #27414, .T. ) ;
#12076=CARTESIAN_POINT ( 'NONE',  ( 5.621891740541981264, -93.55104906477529880, 26.56729936354081190 ) ) ;
#12080=ORIENTED_EDGE ( 'NONE', *, *, #26072, .F. ) ;
#12082=CARTESIAN_POINT ( 'NONE',  ( -5.774731795730000172, -101.2530993039999885, 14.05532693159999980 ) ) ;
#12088=CARTESIAN_POINT ( 'NONE',  ( -20.34965187303443557, -94.63959659917352951, 12.21935051695949603 ) ) ;
#12090=DIRECTION ( 'NONE',  ( 0.7791198649362079953, 0.000000000000000000, -0.6268749764201669850 ) ) ;
#12094=CARTESIAN_POINT ( 'NONE',  ( 21.22741177940000057, -96.73974214489999213, 0.9047775657389999227 ) ) ;
#12107=ADVANCED_FACE ( 'NONE', ( #22609 ), #3234, .F. ) ;
#12108=EDGE_CURVE ( 'NONE', #18837, #7118, #5664, .T. ) ;
#12110=CYLINDRICAL_SURFACE ( 'NONE', #9533, 15.99999999999999467 ) ;
#12112=CARTESIAN_POINT ( 'NONE',  ( 7.618259826220000086, -101.6474417639999928, 14.07078423930000000 ) ) ;
#12114=CARTESIAN_POINT ( 'NONE',  ( 0.000000000000000000, -102.5000000000000000, 0.000000000000000000 ) ) ;
#12116=CARTESIAN_POINT ( 'NONE',  ( -7.864778453279999582, -100.4808658609999981, 14.18740396090000111 ) ) ;
#12120=CARTESIAN_POINT ( 'NONE',  ( 7.350260020649999504, -101.1292391010000102, 13.65356784849999983 ) ) ;
#12121=ORIENTED_EDGE ( 'NONE', *, *, #1406, .F. ) ;
#12126=CARTESIAN_POINT ( 'NONE',  ( 0.000000000000000000, -101.6484611540000031, 0.000000000000000000 ) ) ;
#12127=CARTESIAN_POINT ( 'NONE',  ( 12.11264993960000069, -99.91547912590000635, -13.29325542860000020 ) ) ;
#12128=ORIENTED_EDGE ( 'NONE', *, *, #23777, .F. ) ;
#12132=CARTESIAN_POINT ( 'NONE',  ( -17.63818201149086207, -92.64884742711599586, 24.88264283798182319 ) ) ;
#12136=CARTESIAN_POINT ( 'NONE',  ( 12.96030886027237905, -98.56104087989207585, 15.02160250790822893 ) ) ;
#12137=CARTESIAN_POINT ( 'NONE',  ( -15.54744790750000050, -100.8070272189999912, 2.643184715480000335 ) ) ;
#12140=CARTESIAN_POINT ( 'NONE',  ( 6.916664799299999444, -101.1716782170000073, 14.13220977900000008 ) ) ;
#12141=CARTESIAN_POINT ( 'NONE',  ( 0.000000000000000000, -101.1889999979999999, 0.000000000000000000 ) ) ;
#12142=CARTESIAN_POINT ( 'NONE',  ( 7.500294343269999331, -101.1699703470000031, 13.83260060669999980 ) ) ;
#12146=CARTESIAN_POINT ( 'NONE',  ( -11.73626313630000162, -94.71481430550001335, -21.34524641919999866 ) ) ;
#12153=DIRECTION ( 'NONE',  ( 1.000000000000000000, 0.000000000000000000, 0.000000000000000000 ) ) ;
#12155=CARTESIAN_POINT ( 'NONE',  ( 8.137534397419999621, -101.2306315539999986, 14.02341335179999859 ) ) ;
#12156=CARTESIAN_POINT ( 'NONE',  ( -16.98428476389999631, -99.78393587620000460, 3.406952114930000164 ) ) ;
#12157=ORIENTED_EDGE ( 'NONE', *, *, #13276, .T. ) ;
#12159=CARTESIAN_POINT ( 'NONE',  ( 0.6026929693157587753, -100.4507315469087843, -16.92988022290758110 ) ) ;
#12168=CARTESIAN_POINT ( 'NONE',  ( -17.54428855099999751, -94.59276292389999696, 16.07755916609999858 ) ) ;
#12169=CARTESIAN_POINT ( 'NONE',  ( 13.48409207689999967, -95.94970068820001075, -18.04862505909999726 ) ) ;
#12170=CARTESIAN_POINT ( 'NONE',  ( -14.94683085001314282, -101.1292394719999379, 4.127768892864509986 ) ) ;
#12172=EDGE_CURVE ( 'NONE', #4529, #26855, #13623, .T. ) ;
#12179=CIRCLE ( 'NONE', #8466, 15.19391340349999986 ) ;
#12181=CARTESIAN_POINT ( 'NONE',  ( -29.71161909530000145, -92.92146929989999649, 6.352307300799999723 ) ) ;
#12184=ORIENTED_EDGE ( 'NONE', *, *, #9105, .F. ) ;
#12190=CYLINDRICAL_SURFACE ( 'NONE', #18320, 18.64285714289998808 ) ;
#12193=CARTESIAN_POINT ( 'NONE',  ( 6.308882621530000456, -101.1889999979999999, -29.19167084780000110 ) ) ;
#12197=CARTESIAN_POINT ( 'NONE',  ( -16.29874522269999915, -100.6375206259999970, 3.070048125000000017 ) ) ;
#12201=ORIENTED_EDGE ( 'NONE', *, *, #22175, .T. ) ;
#12202=CARTESIAN_POINT ( 'NONE',  ( 18.83155579810272684, -99.33527509199842598, 0.2391732240786322572 ) ) ;
#12203=ADVANCED_FACE ( 'NONE', ( #14429 ), #14831, .F. ) ;
#12219=CARTESIAN_POINT ( 'NONE',  ( 12.04737265770000043, -101.1889999979999999, -10.52904611289999970 ) ) ;
#12220=CARTESIAN_POINT ( 'NONE',  ( -17.52027961638587783, -99.14332933491964184, 3.769849805601797499 ) ) ;
#12221=ORIENTED_EDGE ( 'NONE', *, *, #14196, .T. ) ;
#12224=FACE_OUTER_BOUND ( 'NONE', #8803, .T. ) ;
#12225=CARTESIAN_POINT ( 'NONE',  ( -5.963512921169999537, -101.1292389529999980, 14.31440776300000017 ) ) ;
#12233=EDGE_CURVE ( 'NONE', #8616, #25599, #17446, .T. ) ;
#12235=FACE_OUTER_BOUND ( 'NONE', #20270, .T. ) ;
#12238=AXIS2_PLACEMENT_3D ( 'NONE', #20620, #9529, #27320 ) ;
#12239=CARTESIAN_POINT ( 'NONE',  ( 14.36320985907368453, -97.53591929634409041, -14.01783439808674991 ) ) ;
#12245=LINE ( 'NONE', #12649, #25023 ) ;
#12246=CARTESIAN_POINT ( 'NONE',  ( 20.55132429533163219, -97.41291607309865697, 1.353383486903313671 ) ) ;
#12249=CIRCLE ( 'NONE', #15969, 6.000000000000000000 ) ;
#12254=VECTOR ( 'NONE', #12819, 1000.000000000000000 ) ;
#12257=CARTESIAN_POINT ( 'NONE',  ( -13.15133982419999903, -100.9197086960000007, -8.436149064220000326 ) ) ;
#12259=B_SPLINE_CURVE_WITH_KNOTS ( 'NONE', 3,
 ( #20284, #13578, #8619, #17523, #26411, #2530, #6599, #9197, #17673, #22045, #4547, #6894, #2094, #7041, #15907, #26556, #4409, #13280, #2225, #11067, #56, #26853, #8904, #26707, #6745, #15610, #24511, #22331, #2376, #27148 ),
 .UNSPECIFIED., .F., .F.,
 ( 4, 1, 1, 1, 1, 2, 2, 1, 1, 1, 1, 2, 2, 2, 1, 1, 1, 1, 2, 2, 4 ),
 ( 0.000000000000000000, 0.1250000000000360545, 0.1875000000000534572, 0.2187500000000621725, 0.2343750000000665579, 0.2421875000000698330, 0.2500000000000731082, 0.3750000000000863198, 0.4375000000000920375, 0.4687500000000958122, 0.4843750000000985878, 0.4921875000000990319, 0.5000000000000994760, 0.6250000000001237899, 0.6875000000001372236, 0.7187500000001429967, 0.7343750000001472156, 0.7421875000001466605, 0.7460937500001444400, 0.7500000000001422196, 1.000000000000000000 ),
 .UNSPECIFIED. ) ;
#12261=CARTESIAN_POINT ( 'NONE',  ( -7.755678108949999761, -100.8746138070000029, 14.68026149039999950 ) ) ;
#12265=CARTESIAN_POINT ( 'NONE',  ( 7.372139244490000465, -101.1290456289999895, 13.64202221559999906 ) ) ;
#12267=EDGE_CURVE ( 'NONE', #20422, #7753, #19886, .T. ) ;
#12269=CARTESIAN_POINT ( 'NONE',  ( -22.29269736170000016, -94.98812656900000206, -8.065862048359999648 ) ) ;
#12275=LINE ( 'NONE', #21187, #26585 ) ;
#12285=CARTESIAN_POINT ( 'NONE',  ( 13.83663993448646323, -97.24405583930904129, -15.54750970113168229 ) ) ;
#12286=CIRCLE ( 'NONE', #15053, 18.14285714289999873 ) ;
#12291=DIRECTION ( 'NONE',  ( 1.000000000000000000, 0.000000000000000000, 0.000000000000000000 ) ) ;
#12292=CARTESIAN_POINT ( 'NONE',  ( -22.49587410578730839, -93.00000237470423770, -19.82286531042224098 ) ) ;
#12293=ORIENTED_EDGE ( 'NONE', *, *, #13439, .F. ) ;
#12294=CIRCLE ( 'NONE', #23484, 20.64285714289999873 ) ;
#12302=CARTESIAN_POINT ( 'NONE',  ( 0.5649143243405088111, -100.9616911410344926, -16.52536945643391775 ) ) ;
#12304=CARTESIAN_POINT ( 'NONE',  ( 13.69010830728659478, -92.58347372262932140, 27.25492602878164305 ) ) ;
#12314=ORIENTED_EDGE ( 'NONE', *, *, #15909, .F. ) ;
#12315=CARTESIAN_POINT ( 'NONE',  ( -11.25326567110000120, -94.84395216780001192, -20.59896464009999661 ) ) ;
#12316=AXIS2_PLACEMENT_3D ( 'NONE', #11058, #45, #6285 ) ;
#12321=CARTESIAN_POINT ( 'NONE',  ( -29.43780281349999939, -92.91851489729999969, 4.711604253540000009 ) ) ;
#12324=CIRCLE ( 'NONE', #4897, 18.14285714289999518 ) ;
#12328=CARTESIAN_POINT ( 'NONE',  ( -5.873418876839999747, -101.1889999979999999, 15.15334698740000086 ) ) ;
#12331=CARTESIAN_POINT ( 'NONE',  ( 25.81290055409999695, -93.01584738559999721, -5.657397443709999862 ) ) ;
#12334=CARTESIAN_POINT ( 'NONE',  ( -15.35765514150000044, -101.3349956970000108, 4.566393778230000144 ) ) ;
#12335=CARTESIAN_POINT ( 'NONE',  ( -16.34872446949999869, -100.7006823539999942, 3.091720520159999985 ) ) ;
#12338=ORIENTED_EDGE ( 'NONE', *, *, #18745, .T. ) ;
#12348=CARTESIAN_POINT ( 'NONE',  ( 6.757998639866319657, -100.5550990438330956, 15.44352938470917991 ) ) ;
#12350=EDGE_CURVE ( 'NONE', #10205, #19075, #1382, .T. ) ;
#12354=CARTESIAN_POINT ( 'NONE',  ( -5.547446579819999890, -101.0848057460000007, 14.37961489299999940 ) ) ;
#12356=ORIENTED_EDGE ( 'NONE', *, *, #6404, .T. ) ;
#12357=CARTESIAN_POINT ( 'NONE',  ( 0.000000000000000000, -102.5000000000000000, 0.000000000000000000 ) ) ;
#12358=CARTESIAN_POINT ( 'NONE',  ( -28.95818204711633115, -93.00000166546705316, -1.362778528346119566 ) ) ;
#12359=ADVANCED_FACE ( 'NONE', ( #10575 ), #25009, .T. ) ;
#12363=CARTESIAN_POINT ( 'NONE',  ( 16.76176042277295863, -99.62767017971319206, 4.428935492921096895 ) ) ;
#12366=CARTESIAN_POINT ( 'NONE',  ( -20.59660110919999809, -95.94970068810000896, -9.129820831349999111 ) ) ;
#12367=CARTESIAN_POINT ( 'NONE',  ( 16.79023019859999977, -99.83167544280000527, 4.266711010680000804 ) ) ;
#12368=CARTESIAN_POINT ( 'NONE',  ( 23.96865075879999907, -92.76843000840000286, -18.60167795649999789 ) ) ;
#12373=LINE ( 'NONE', #10181, #20181 ) ;
#12377=CARTESIAN_POINT ( 'NONE',  ( -6.665307709260000379, -92.50000000000000000, -13.13558364449999871 ) ) ;
#12388=CARTESIAN_POINT ( 'NONE',  ( 9.385332722619999402, -98.68450614990000247, 16.47661810339999988 ) ) ;
#12390=CARTESIAN_POINT ( 'NONE',  ( -17.06978221569999832, -93.00000000760000773, -23.47580390800000316 ) ) ;
#12391=CARTESIAN_POINT ( 'NONE',  ( 3.778421007439999979, -92.49999846069999876, 28.62986538160000194 ) ) ;
#12393=DIRECTION ( 'NONE',  ( 0.000000000000000000, 1.000000000000000000, 0.000000000000000000 ) ) ;
#12395=CARTESIAN_POINT ( 'NONE',  ( 12.82719021566207473, -101.4304678898291172, -9.842949757285465395 ) ) ;
#12396=CARTESIAN_POINT ( 'NONE',  ( 16.62464038829999780, -111.0000000000000000, 13.20435077039999960 ) ) ;
#12403=CARTESIAN_POINT ( 'NONE',  ( -17.06205513267597240, -92.82334897402063234, 25.28114489634798900 ) ) ;
#12405=DIRECTION ( 'NONE',  ( 1.000000000000000000, 0.000000000000000000, 0.000000000000000000 ) ) ;
#12408=CARTESIAN_POINT ( 'NONE',  ( 15.86628499849999940, -101.4334236450000049, 2.533787873950000158 ) ) ;
#12411=CARTESIAN_POINT ( 'NONE',  ( 6.525449878219999889, -99.97545561319999763, 15.58947632439999964 ) ) ;
#12412=CARTESIAN_POINT ( 'NONE',  ( 15.01376502369999955, -101.1030539030000028, 3.591278379049999803 ) ) ;
#12413=EDGE_CURVE ( 'NONE', #14792, #11909, #21268, .T. ) ;
#12414=CARTESIAN_POINT ( 'NONE',  ( -11.57961683250000107, -94.58575303309999072, -20.85094915950000072 ) ) ;
#12416=CARTESIAN_POINT ( 'NONE',  ( 6.161525631346291831, -92.49999999999998579, -29.87131533446021692 ) ) ;
#12417=CARTESIAN_POINT ( 'NONE',  ( -8.015006079049999954, -99.64579499010000063, 15.35521677919999917 ) ) ;
#12418=CARTESIAN_POINT ( 'NONE',  ( 8.320075280630000236, -93.86380869120000625, -23.56309038849999737 ) ) ;
#12419=CIRCLE ( 'NONE', #3599, 5.500000000000000000 ) ;
#12423=DIRECTION ( 'NONE',  ( 0.000000000000000000, 1.000000000000000000, 0.000000000000000000 ) ) ;
#12426=CARTESIAN_POINT ( 'NONE',  ( -5.582121642149999730, -100.8816835080000089, 14.77497840909999915 ) ) ;
#12429=DIRECTION ( 'NONE',  ( 1.000000000000000000, 0.000000000000000000, 0.000000000000000000 ) ) ;
#12430=CARTESIAN_POINT ( 'NONE',  ( 0.1502068069240189152, -101.5526869445977667, -16.07314774595968743 ) ) ;
#12435=CARTESIAN_POINT ( 'NONE',  ( 15.45219090089999980, -100.9364576079999978, 3.957211818329999797 ) ) ;
#12442=TOROIDAL_SURFACE ( 'NONE', #28722, 29.91857981989999971, 10.00000000000000000 ) ;
#12448=VECTOR ( 'NONE', #13727, 1000.000000000000000 ) ;
#12452=ORIENTED_EDGE ( 'NONE', *, *, #6148, .F. ) ;
#12461=CARTESIAN_POINT ( 'NONE',  ( -16.33619708059999809, -111.0000000000000000, 3.920288885250000188 ) ) ;
#12462=CARTESIAN_POINT ( 'NONE',  ( -15.15090857039999861, -101.1124885629999994, 3.392036723980000001 ) ) ;
#12471=CARTESIAN_POINT ( 'NONE',  ( 0.000000000000000000, -92.50000000000000000, 29.91857981989999971 ) ) ;
#12473=VERTEX_POINT ( 'NONE', #27909 ) ;
#12485=VERTEX_POINT ( 'NONE', #10519 ) ;
#12486=B_SPLINE_CURVE_WITH_KNOTS ( 'NONE', 3,
 ( #23848, #4170, #26034, #28216, #12613, #8250, #21525, #14941, #19340, #3888 ),
 .UNSPECIFIED., .F., .F.,
 ( 4, 2, 2, 2, 4 ),
 ( 0.000000000000000000, 0.2500000000000000000, 0.5000000000000000000, 0.7500000000000000000, 1.000000000000000000 ),
 .UNSPECIFIED. ) ;
#12490=ORIENTED_EDGE ( 'NONE', *, *, #21359, .F. ) ;
#12491=CARTESIAN_POINT ( 'NONE',  ( -3.528528669317067656, -97.24405583809684117, -20.51163445666866636 ) ) ;
#12493=AXIS2_PLACEMENT_3D ( 'NONE', #20429, #17957, #6887 ) ;
#12495=CARTESIAN_POINT ( 'NONE',  ( 7.579179873580000226, -101.3235621230000021, 13.98627925510000125 ) ) ;
#12496=CARTESIAN_POINT ( 'NONE',  ( -17.76804213369999985, -93.83763213849999829, 19.50200951540000105 ) ) ;
#12497=ORIENTED_EDGE ( 'NONE', *, *, #2956, .T. ) ;
#12501=CARTESIAN_POINT ( 'NONE',  ( 18.39461646259999839, -98.93445099689999722, 3.291678619879999879 ) ) ;
#12503=EDGE_CURVE ( 'NONE', #13839, #26488, #9204, .T. ) ;
#12504=CARTESIAN_POINT ( 'NONE',  ( 23.83720300980000317, -93.60790942699999562, -8.962666302020000586 ) ) ;
#12506=AXIS2_PLACEMENT_3D ( 'NONE', #17797, #36, #10911 ) ;
#12511=CARTESIAN_POINT ( 'NONE',  ( -15.36947826900000003, -101.0685828069999985, 4.769131590209999771 ) ) ;
#12516=DIRECTION ( 'NONE',  ( 0.000000000000000000, -1.000000000000000000, 0.000000000000000000 ) ) ;
#12518=VECTOR ( 'NONE', #27235, 1000.000000000000000 ) ;
#12523=CARTESIAN_POINT ( 'NONE',  ( 7.635702898730000854, -101.6454117330000031, 14.06304778130000166 ) ) ;
#12525=B_SPLINE_CURVE_WITH_KNOTS ( 'NONE', 3,
 ( #24559, #19883, #17719, #26603, #6645, #8953, #17864, #15507, #4598, #24417, #13475, #22381, #22675, #7234, #26903, #5034, #2719, #551, #20483, #2867, #24713, #20789, #11728, #9398, #16243, #13773, #18304, #15955, #11573, #7538 ),
 .UNSPECIFIED., .F., .F.,
 ( 4, 1, 1, 1, 1, 2, 2, 1, 1, 1, 1, 2, 2, 2, 1, 1, 1, 1, 2, 2, 4 ),
 ( 0.000000000000000000, 0.1249999999999861222, 0.1874999999999780731, 0.2187499999999731881, 0.2343749999999721334, 0.2421874999999739375, 0.2499999999999757416, 0.3749999999999756861, 0.4374999999999746869, 0.4687499999999725775, 0.4843749999999715228, 0.4921874999999713007, 0.4999999999999710232, 0.6249999999999793499, 0.6874999999999844569, 0.7187499999999875655, 0.7343749999999872324, 0.7421874999999861222, 0.7460937499999883427, 0.7499999999999905631, 1.000000000000000000 ),
 .UNSPECIFIED. ) ;
#12526=CARTESIAN_POINT ( 'NONE',  ( -13.02193338449999871, -101.6484611580000035, -9.297634755529999850 ) ) ;
#12527=CARTESIAN_POINT ( 'NONE',  ( -8.138356485639999249, -99.77922884479998800, 15.08989400399999958 ) ) ;
#12528=CARTESIAN_POINT ( 'NONE',  ( -2.749191855459999889, -99.88544659679999427, -17.64021669569999773 ) ) ;
#12530=CARTESIAN_POINT ( 'NONE',  ( 11.70394544829403216, -98.37417905365539639, -16.31992250965110003 ) ) ;
#12532=CARTESIAN_POINT ( 'NONE',  ( 13.30228833790079612, -100.9229461902416887, -9.872452464501236591 ) ) ;
#12545=CARTESIAN_POINT ( 'NONE',  ( 0.05051043905469999873, -101.1284992150000051, -15.40552557020000002 ) ) ;
#12552=ADVANCED_FACE ( 'NONE', ( #26515 ), #12442, .F. ) ;
#12553=B_SPLINE_CURVE_WITH_KNOTS ( 'NONE', 3,
 ( #8231, #17127, #18907, #21505, #3732, #27788, #26015, #18767, #14786, #27663 ),
 .UNSPECIFIED., .F., .F.,
 ( 4, 2, 2, 2, 4 ),
 ( 0.000000000000000000, 0.2500000000000000000, 0.5000000000000000000, 0.7500000000000000000, 1.000000000000000000 ),
 .UNSPECIFIED. ) ;
#12554=CARTESIAN_POINT ( 'NONE',  ( 6.072376808220000477, -100.9137139110000021, 14.40534646189999890 ) ) ;
#12555=CARTESIAN_POINT ( 'NONE',  ( 15.63748056140000209, -101.6484611540000031, 3.386620984279999913 ) ) ;
#12561=CARTESIAN_POINT ( 'NONE',  ( 8.649323485130000932, -94.16309976680000204, -22.83302821760000256 ) ) ;
#12565=CARTESIAN_POINT ( 'NONE',  ( -13.26856174610000139, -93.91547326100000248, -20.89962974999999901 ) ) ;
#12566=CARTESIAN_POINT ( 'NONE',  ( -6.781378104809999030, -101.6484611540000031, 14.49182221120000058 ) ) ;
#12570=EDGE_LOOP ( 'NONE', ( #23900, #10918, #2093, #6376, #17173, #10995, #13389 ) ) ;
#12571=CARTESIAN_POINT ( 'NONE',  ( -0.8744470429980000237, -101.1848541600000004, -15.25816383929999986 ) ) ;
#12572=CARTESIAN_POINT ( 'NONE',  ( 7.286238495500000134, -101.2500498790000023, 13.33737010350000141 ) ) ;
#12573=CARTESIAN_POINT ( 'NONE',  ( 13.13193815604943460, -92.93978723899418526, 27.52821129672017264 ) ) ;
#12583=ORIENTED_EDGE ( 'NONE', *, *, #28496, .T. ) ;
#12584=B_SPLINE_CURVE_WITH_KNOTS ( 'NONE', 5,
 ( #24786, #26377, #15582, #15427, #6405, #22157, #2059, #17640, #17787 ),
 .UNSPECIFIED., .F., .F.,
 ( 6, 3, 6 ),
 ( 0.000000000000000000, 0.5000000000000000000, 1.000000000000000000 ),
 .UNSPECIFIED. ) ;
#12591=CARTESIAN_POINT ( 'NONE',  ( -29.69641156999999865, -92.84292833370000153, 6.354845228289999426 ) ) ;
#12592=CARTESIAN_POINT ( 'NONE',  ( 9.397459420459995272, -94.89420224095998435, -22.59846300103535199 ) ) ;
#12594=ORIENTED_EDGE ( 'NONE', *, *, #3588, .F. ) ;
#12595=CARTESIAN_POINT ( 'NONE',  ( -17.90995366394907862, -97.42330309962233059, -10.14262162657689359 ) ) ;
#12596=FACE_OUTER_BOUND ( 'NONE', #26214, .T. ) ;
#12597=VERTEX_POINT ( 'NONE', #13694 ) ;
#12598=CIRCLE ( 'NONE', #24740, 15.19391340349999986 ) ;
#12601=ORIENTED_EDGE ( 'NONE', *, *, #27187, .F. ) ;
#12602=AXIS2_PLACEMENT_3D ( 'NONE', #17842, #26738, #15635 ) ;
#12604=EDGE_CURVE ( 'NONE', #26971, #12597, #2155, .T. ) ;
#12612=CARTESIAN_POINT ( 'NONE',  ( -12.36343567480000161, -101.1716782170000073, -9.731652660190000859 ) ) ;
#12613=CARTESIAN_POINT ( 'NONE',  ( 22.01067795732654275, -93.33134965528456917, 15.58958953133906000 ) ) ;
#12614=CARTESIAN_POINT ( 'NONE',  ( -7.679489405794825529, -100.9609609849295424, 14.64415966093239874 ) ) ;
#12617=AXIS2_PLACEMENT_3D ( 'NONE', #3565, #12423, #838 ) ;
#12621=ORIENTED_EDGE ( 'NONE', *, *, #1592, .F. ) ;
#12623=CARTESIAN_POINT ( 'NONE',  ( 6.671273368871432297, -100.8738282931630863, 15.20505492520185875 ) ) ;
#12624=CARTESIAN_POINT ( 'NONE',  ( 11.77387480661665187, -101.1586404113069335, -10.29001710982078777 ) ) ;
#12625=EDGE_LOOP ( 'NONE', ( #2604, #18256, #1047, #27676 ) ) ;
#12629=CARTESIAN_POINT ( 'NONE',  ( -23.77081188420000046, -111.0000000000000000, -19.11016751280000037 ) ) ;
#12633=FACE_OUTER_BOUND ( 'NONE', #17814, .T. ) ;
#12634=CARTESIAN_POINT ( 'NONE',  ( -30.34790777679999962, -93.00000000000000000, 3.042119914239999723 ) ) ;
#12635=CARTESIAN_POINT ( 'NONE',  ( 20.98778206287693493, -96.61062616032549499, -3.223209917027987093 ) ) ;
#12637=CARTESIAN_POINT ( 'NONE',  ( -18.17993916029999824, -94.51629284240000572, 17.35042103430000182 ) ) ;
#12638=ORIENTED_EDGE ( 'NONE', *, *, #8477, .F. ) ;
#12639=CARTESIAN_POINT ( 'NONE',  ( -16.85779618499999799, -97.58045781630001159, -10.78314124750000147 ) ) ;
#12641=CARTESIAN_POINT ( 'NONE',  ( 12.82866288339999983, -100.7707614970000094, -9.316536369119999605 ) ) ;
#12643=CARTESIAN_POINT ( 'NONE',  ( 23.73696482120000084, -93.59856727309998803, -8.983699850290001621 ) ) ;
#12649=CARTESIAN_POINT ( 'NONE',  ( 11.86655840719999944, -101.1889999979999999, -11.10431293650000129 ) ) ;
#12651=CARTESIAN_POINT ( 'NONE',  ( -1.013078509969999973E-15, -101.6484611540000031, -5.329070518200000398E-15 ) ) ;
#12665=CARTESIAN_POINT ( 'NONE',  ( -12.98104160269999952, -101.4254868690000109, -9.301111302380000723 ) ) ;
#12668=CARTESIAN_POINT ( 'NONE',  ( -8.046121148190000127, -99.85455315880000171, 15.13041121020000013 ) ) ;
#12675=CARTESIAN_POINT ( 'NONE',  ( 12.51632808644059836, -101.6297509123139235, -9.990436032579999903 ) ) ;
#12678=CARTESIAN_POINT ( 'NONE',  ( 8.920182828499999772, -94.54719592040000009, -22.12534720020000023 ) ) ;
#12680=B_SPLINE_CURVE_WITH_KNOTS ( 'NONE', 3,
 ( #16503, #14723, #25676, #14587, #27731, #23346 ),
 .UNSPECIFIED., .F., .F.,
 ( 4, 2, 4 ),
 ( 0.000000000000000000, 0.5000000000000000000, 1.000000000000000000 ),
 .UNSPECIFIED. ) ;
#12681=DIRECTION ( 'NONE',  ( 0.3790931394101558771, -0.6121731929912518355, 0.6939253370752848094 ) ) ;
#12684=CARTESIAN_POINT ( 'NONE',  ( -17.55208023420000174, -93.64386272749999307, 18.16437695980000200 ) ) ;
#12685=DIRECTION ( 'NONE',  ( 0.7748485350940619298, 0.000000000000000000, -0.6321469351840490747 ) ) ;
#12687=CARTESIAN_POINT ( 'NONE',  ( 12.61209325099999923, -111.0000000000000000, -11.02259514940000074 ) ) ;
#12692=EDGE_LOOP ( 'NONE', ( #5271, #17128, #27257, #7724 ) ) ;
#12693=CARTESIAN_POINT ( 'NONE',  ( 6.968069840630000122, -100.0482783049999966, 15.72019133129999879 ) ) ;
#12694=CARTESIAN_POINT ( 'NONE',  ( 15.36147648729999915, -101.1716782170000073, 3.403622381159999932 ) ) ;
#12696=CARTESIAN_POINT ( 'NONE',  ( -7.879410208250000380, -99.92967571559999840, 15.46934584979999983 ) ) ;
#12702=TOROIDAL_SURFACE ( 'NONE', #16915, 5.500000000000000000, 0.5000000000000000000 ) ;
#12703=CARTESIAN_POINT ( 'NONE',  ( 4.742489832159999530, -92.98926436760000058, -27.98920360839999688 ) ) ;
#12705=DIRECTION ( 'NONE',  ( 0.000000000000000000, 1.000000000000000000, 0.000000000000000000 ) ) ;
#12706=CARTESIAN_POINT ( 'NONE',  ( -6.768220873529999793, -101.4254868729999970, 14.46370517449999937 ) ) ;
#12708=FACE_OUTER_BOUND ( 'NONE', #2108, .T. ) ;
#12709=CARTESIAN_POINT ( 'NONE',  ( -12.56985916528515190, -100.9570234915280338, -10.74835527338169427 ) ) ;
#12710=ORIENTED_EDGE ( 'NONE', *, *, #4298, .T. ) ;
#12711=EDGE_CURVE ( 'NONE', #21689, #21931, #18936, .T. ) ;
#12717=CARTESIAN_POINT ( 'NONE',  ( -13.18688177930000016, -93.32822605769999313, -23.58441486170000090 ) ) ;
#12719=CARTESIAN_POINT ( 'NONE',  ( 16.34567793506732869, -94.63270597576601517, 17.22370556663485175 ) ) ;
#12723=CIRCLE ( 'NONE', #4856, 11.00000000000000000 ) ;
#12733=CARTESIAN_POINT ( 'NONE',  ( -29.38881566890000130, -92.76004107139999633, 4.720288864379999616 ) ) ;
#12737=EDGE_LOOP ( 'NONE', ( #2670, #24778, #23696, #26638, #17979, #7519, #27415 ) ) ;
#12738=CARTESIAN_POINT ( 'NONE',  ( -18.87800995732253995, -96.89152198193129095, -9.790682212865581491 ) ) ;
#12741=CIRCLE ( 'NONE', #1182, 0.5000000000000009992 ) ;
#12743=EDGE_CURVE ( 'NONE', #1488, #28309, #8724, .T. ) ;
#12744=EDGE_LOOP ( 'NONE', ( #3533, #23499, #4000, #22488 ) ) ;
#12747=CARTESIAN_POINT ( 'NONE',  ( -15.32098868920000001, -101.1716782350000017, 3.581867792729999778 ) ) ;
#12748=DIRECTION ( 'NONE',  ( 1.000000000000000000, 0.000000000000000000, 0.000000000000000000 ) ) ;
#12749=CARTESIAN_POINT ( 'NONE',  ( 11.12836528380000090, -101.0356131030000029, -10.75380786670000077 ) ) ;
#12752=CARTESIAN_POINT ( 'NONE',  ( -12.55296505889999992, -100.8088109309999965, -10.78431163630000000 ) ) ;
#12756=CARTESIAN_POINT ( 'NONE',  ( -0.9692006007005103951, -101.5902664364219277, -16.01432838750588061 ) ) ;
#12762=CARTESIAN_POINT ( 'NONE',  ( 6.667714868184677179, -101.2021794473701988, 14.92458339438100801 ) ) ;
#12764=ORIENTED_EDGE ( 'NONE', *, *, #23078, .F. ) ;
#12774=CARTESIAN_POINT ( 'NONE',  ( -3.371331056789452774, -97.34036579176134296, -20.41252770651184179 ) ) ;
#12779=CARTESIAN_POINT ( 'NONE',  ( -22.02936738240000025, -92.83702889919999279, -20.06351774230000373 ) ) ;
#12781=EDGE_LOOP ( 'NONE', ( #14819, #2659, #25720, #21355 ) ) ;
#12782=CARTESIAN_POINT ( 'NONE',  ( -13.27621816679999966, -99.83167544280000527, -11.12918164819999944 ) ) ;
#12783=CARTESIAN_POINT ( 'NONE',  ( 12.16870387880000060, -101.1030539030000028, -9.499108720959998919 ) ) ;
#12785=CARTESIAN_POINT ( 'NONE',  ( 23.81109335309999864, -94.64125147549999895, -7.489946264089999417 ) ) ;
#12787=CARTESIAN_POINT ( 'NONE',  ( 29.84209778924876844, -92.58608763743339409, 6.300736884733585619 ) ) ;
#12792=CARTESIAN_POINT ( 'NONE',  ( 6.153525452890544756, -92.86910576385621141, 28.82527858285896016 ) ) ;
#12794=CARTESIAN_POINT ( 'NONE',  ( 0.1199839491673418412, -92.96960399592218494, -30.49976399678630301 ) ) ;
#12796=ORIENTED_EDGE ( 'NONE', *, *, #16712, .F. ) ;
#12797=ADVANCED_FACE ( 'NONE', ( #24001 ), #17452, .F. ) ;
#12799=DIRECTION ( 'NONE',  ( 1.000000000000000000, 0.000000000000000000, 0.000000000000000000 ) ) ;
#12805=EDGE_CURVE ( 'NONE', #4037, #19516, #3897, .T. ) ;
#12806=CARTESIAN_POINT ( 'NONE',  ( -12.99806807920000118, -101.2995922080000071, -9.195720578049998650 ) ) ;
#12807=CARTESIAN_POINT ( 'NONE',  ( -13.16778098350000015, -93.19477590270000178, -23.58326777899999982 ) ) ;
#12808=CARTESIAN_POINT ( 'NONE',  ( -7.983017350639999954, -99.94751438429999268, 15.18573513309999790 ) ) ;
#12809=CARTESIAN_POINT ( 'NONE',  ( -3.055530165179999980, -94.70873790529999781, 23.49572270359999848 ) ) ;
#12814=CARTESIAN_POINT ( 'NONE',  ( 13.63841234616398879, -100.4010812937911510, -10.11563007918305601 ) ) ;
#12819=DIRECTION ( 'NONE',  ( 0.000000000000000000, 1.000000000000000000, 0.000000000000000000 ) ) ;
#12825=ADVANCED_FACE ( 'NONE', ( #28648 ), #18504, .T. ) ;
#12832=CARTESIAN_POINT ( 'NONE',  ( 6.775066376809999902, -101.3878691800000098, 14.60824414760000067 ) ) ;
#12833=CARTESIAN_POINT ( 'NONE',  ( 14.96872597019999951, -101.0403179300000005, 3.906879788429999500 ) ) ;
#12834=EDGE_CURVE ( 'NONE', #22453, #842, #12553, .T. ) ;
#12839=CARTESIAN_POINT ( 'NONE',  ( 8.467196410959999753, -93.92589062430000979, -23.69480735049999964 ) ) ;
#12844=CARTESIAN_POINT ( 'NONE',  ( -12.83467265744653929, -100.4872618010412992, -11.01232127950116890 ) ) ;
#12846=CARTESIAN_POINT ( 'NONE',  ( 26.24918299980000214, -92.87437365140000622, -7.909057152789999989 ) ) ;
#12848=CARTESIAN_POINT ( 'NONE',  ( 12.82422237299999956, -94.98812477769999418, -19.93894812050000098 ) ) ;
#12851=CARTESIAN_POINT ( 'NONE',  ( -19.78043542534729227, -92.52498922770500656, -23.21615846764749236 ) ) ;
#12853=CARTESIAN_POINT ( 'NONE',  ( -6.439729480049999566, -101.2530993010000060, 13.76171823350000167 ) ) ;
#12856=CARTESIAN_POINT ( 'NONE',  ( 13.75485398520459057, -100.1406256088168760, -10.30979386037251189 ) ) ;
#12869=DIRECTION ( 'NONE',  ( 0.4794255386042040601, 0.000000000000000000, 0.8775825618903722036 ) ) ;
#12871=CARTESIAN_POINT ( 'NONE',  ( -15.02595431881585242, -98.99956644457965638, -10.95841658774190108 ) ) ;
#12874=ORIENTED_EDGE ( 'NONE', *, *, #6069, .F. ) ;
#12884=ORIENTED_EDGE ( 'NONE', *, *, #21421, .T. ) ;
#12886=CARTESIAN_POINT ( 'NONE',  ( -11.89877799829999994, -101.0147083550000104, -10.00853575740000068 ) ) ;
#12889=CARTESIAN_POINT ( 'NONE',  ( -7.860694240047618742, -100.5550990450661573, 14.91249917024564198 ) ) ;
#12896=EDGE_CURVE ( 'NONE', #17152, #2628, #11525, .T. ) ;
#12900=CARTESIAN_POINT ( 'NONE',  ( 12.02686724500000004, -92.54157628459999785, 27.32173438410000088 ) ) ;
#12903=CARTESIAN_POINT ( 'NONE',  ( -15.11912402641494424, -93.86130746169172312, -21.61442877420574149 ) ) ;
#12914=CARTESIAN_POINT ( 'NONE',  ( -18.88944331899999796, -93.00000000000000000, -23.13319212550000259 ) ) ;
#12915=CARTESIAN_POINT ( 'NONE',  ( -21.97175844099999864, -92.62399497440000573, -19.94807775750000189 ) ) ;
#12918=CARTESIAN_POINT ( 'NONE',  ( -15.09406086359999932, -98.83667233820000320, -10.95640931279999997 ) ) ;
#12919=CARTESIAN_POINT ( 'NONE',  ( 12.62715338020000111, -101.2063419769999939, -9.804727914620000817 ) ) ;
#12922=CARTESIAN_POINT ( 'NONE',  ( 29.85855671192240379, -92.56772982766284485, 6.222565568561500449 ) ) ;
#12925=ADVANCED_FACE ( 'NONE', ( #14657 ), #20368, .F. ) ;
#12927=FACE_OUTER_BOUND ( 'NONE', #25349, .T. ) ;
#12929=CARTESIAN_POINT ( 'NONE',  ( 12.04737265770000043, -101.6484611540000031, -10.52904611289999970 ) ) ;
#12946=CARTESIAN_POINT ( 'NONE',  ( -12.61650973899999961, -101.1516803200000112, -8.702315162139999671 ) ) ;
#12957=CARTESIAN_POINT ( 'NONE',  ( 13.48463565429420896, -100.6644468680852924, -9.970219641038934100 ) ) ;
#12960=CARTESIAN_POINT ( 'NONE',  ( -16.79027416539999962, -100.2529091920000042, 3.234199557169999739 ) ) ;
#12964=CARTESIAN_POINT ( 'NONE',  ( -17.60151059589999889, -93.41955571290000648, 19.34924659089999821 ) ) ;
#12971=CARTESIAN_POINT ( 'NONE',  ( 0.2107703687019999994, -101.2927714249999980, -16.05360085099999878 ) ) ;
#12973=CARTESIAN_POINT ( 'NONE',  ( 15.28252213929999925, -101.1292389529999980, 2.628739817060000039 ) ) ;
#12979=CARTESIAN_POINT ( 'NONE',  ( 6.601639229639999940, -100.7430069139999915, 15.11370351929999956 ) ) ;
#12980=CARTESIAN_POINT ( 'NONE',  ( 14.80905440220000102, -101.2358105800000061, 3.500992360309999718 ) ) ;
#12981=CARTESIAN_POINT ( 'NONE',  ( -5.892551212131841076, -97.41291607174348144, 19.73490353248802265 ) ) ;
#12982=EDGE_LOOP ( 'NONE', ( #24520, #17142, #17236, #23583 ) ) ;
#12983=CARTESIAN_POINT ( 'NONE',  ( -13.30284256589999892, -92.50000025620001054, 26.72171909750000296 ) ) ;
#12984=CARTESIAN_POINT ( 'NONE',  ( 5.191020918613762802, -92.62800705126865353, -30.05509293616334787 ) ) ;
#12985=B_SPLINE_CURVE_WITH_KNOTS ( 'NONE', 3,
 ( #3833, #6151, #26272, #15303, #4110, #3695, #8069, #3974, #16959, #26123, #12981, #10784, #8201, #28586, #26409, #17088, #12696 ),
 .UNSPECIFIED., .F., .F.,
 ( 4, 2, 2, 1, 1, 1, 1, 1, 2, 2, 4 ),
 ( 0.000000000000000000, 0.2500000000001315059, 0.3750000000001976752, 0.4375000000002307043, 0.4687500000002471912, 0.4843750000002554623, 0.4921875000002595701, 0.4960937500002607914, 0.4980468750002605693, 0.5000000000002603473, 1.000000000000000000 ),
 .UNSPECIFIED. ) ;
#12988=CARTESIAN_POINT ( 'NONE',  ( 6.586633760479999822, -93.48569568790000517, -26.38833621560000253 ) ) ;
#12994=CARTESIAN_POINT ( 'NONE',  ( -12.95358181834116351, -100.3266728694473073, -11.07102962069259000 ) ) ;
#12997=CARTESIAN_POINT ( 'NONE',  ( 27.07127711109999879, -92.49999846069999876, -10.05443248829999980 ) ) ;
#13001=FACE_OUTER_BOUND ( 'NONE', #25290, .T. ) ;
#13006=CARTESIAN_POINT ( 'NONE',  ( -14.73065703810000038, -101.1848546039999945, 4.068069544640000146 ) ) ;
#13007=CARTESIAN_POINT ( 'NONE',  ( 16.31233561804996057, -94.64857743460261474, 17.22706169121702047 ) ) ;
#13009=CARTESIAN_POINT ( 'NONE',  ( 26.51307495810083381, -92.55389105864081500, 13.35502057535796894 ) ) ;
#13010=CYLINDRICAL_SURFACE ( 'NONE', #4055, 5.000000000000001776 ) ;
#13014=VERTEX_POINT ( 'NONE', #17854 ) ;
#13021=CARTESIAN_POINT ( 'NONE',  ( -25.12376022900000194, -94.06807348059999185, -3.039477672979999934 ) ) ;
#13032=B_SPLINE_CURVE_WITH_KNOTS ( 'NONE', 3,
 ( #2176, #4496, #22431, #19929, #3, #26805, #13370, #4202, #19642, #22274, #2322, #11174, #17471, #9004, #20235, #306, #9145 ),
 .UNSPECIFIED., .F., .F.,
 ( 4, 2, 2, 1, 1, 1, 1, 1, 2, 2, 4 ),
 ( 0.000000000000000000, 0.2500000000000727751, 0.3750000000001091349, 0.4375000000001275646, 0.4687500000001377787, 0.4843750000001418865, 0.4921875000001446621, 0.4960937500001461054, 0.4980468750001466050, 0.5000000000001471046, 1.000000000000000000 ),
 .UNSPECIFIED. ) ;
#13041=CARTESIAN_POINT ( 'NONE',  ( -13.46646228700000059, -101.3150700380000018, -9.098096927170001180 ) ) ;
#13042=ORIENTED_EDGE ( 'NONE', *, *, #15583, .F. ) ;
#13045=CARTESIAN_POINT ( 'NONE',  ( -12.28682837150000040, -101.1417990620000040, -9.866547330559999551 ) ) ;
#13047=CARTESIAN_POINT ( 'NONE',  ( -7.647449374585493231, -101.0147714268888848, 14.61310169654407254 ) ) ;
#13053=CIRCLE ( 'NONE', #11206, 9.999999999999996447 ) ;
#13059=CARTESIAN_POINT ( 'NONE',  ( -20.43932202180000246, -94.59276292389999696, 12.18704577789999988 ) ) ;
#13061=CARTESIAN_POINT ( 'NONE',  ( 24.22266071560000000, -93.30149109789999784, 12.29404703189999815 ) ) ;
#13068=CARTESIAN_POINT ( 'NONE',  ( -29.47185689770189398, -92.86910576385491822, -0.4149841894467364845 ) ) ;
#13075=CARTESIAN_POINT ( 'NONE',  ( 12.69294339169999830, -100.9137139110000021, -9.125620792290000338 ) ) ;
#13082=ORIENTED_EDGE ( 'NONE', *, *, #3508, .F. ) ;
#13084=CARTESIAN_POINT ( 'NONE',  ( -29.91144828099999842, -92.50000000000000000, -0.6532076026720000650 ) ) ;
#13086=CARTESIAN_POINT ( 'NONE',  ( -14.42556421679999978, -101.1889999979999999, -2.978755036369999942 ) ) ;
#13088=CARTESIAN_POINT ( 'NONE',  ( 19.91489911684789504, -97.53591929688253970, 2.489632866012725820 ) ) ;
#13092=ORIENTED_EDGE ( 'NONE', *, *, #13137, .T. ) ;
#13093=CARTESIAN_POINT ( 'NONE',  ( 22.33318586679999740, -95.76596938049999608, -4.313430884220000650 ) ) ;
#13097=ORIENTED_EDGE ( 'NONE', *, *, #7224, .T. ) ;
#13099=DIRECTION ( 'NONE',  ( 1.000000000000000000, 0.000000000000000000, 0.000000000000000000 ) ) ;
#13104=CARTESIAN_POINT ( 'NONE',  ( -4.535184989290000246, -98.41760973750001540, -18.76514591000000109 ) ) ;
#13105=CARTESIAN_POINT ( 'NONE',  ( -29.21843812340000213, -92.50000000000000000, 6.434616699369999360 ) ) ;
#13106=CARTESIAN_POINT ( 'NONE',  ( -20.22328760799999969, -94.79579754960001026, 12.30739653150000024 ) ) ;
#13107=CARTESIAN_POINT ( 'NONE',  ( -29.74292299291512620, -92.82709422631626239, 6.753409419028412408 ) ) ;
#13108=CARTESIAN_POINT ( 'NONE',  ( 11.92827614917728418, -99.33527508908198911, -14.57398112561237191 ) ) ;
#13117=CARTESIAN_POINT ( 'NONE',  ( -18.02343650629999772, -94.04288410259999864, 18.38798360810000077 ) ) ;
#13119=ORIENTED_EDGE ( 'NONE', *, *, #8694, .T. ) ;
#13121=CIRCLE ( 'NONE', #10797, 0.7499999999999997780 ) ;
#13122=CARTESIAN_POINT ( 'NONE',  ( 0.4502802160170000234, -100.9678331089999972, -16.17514339299999904 ) ) ;
#13131=CARTESIAN_POINT ( 'NONE',  ( 3.787197165510000296, -93.00000000000000000, -30.26395773239999798 ) ) ;
#13133=CARTESIAN_POINT ( 'NONE',  ( -4.400377801179999437, -95.75647260670000094, 22.05748086060000190 ) ) ;
#13135=CARTESIAN_POINT ( 'NONE',  ( 9.397448849349999023, -94.89419905519999077, -22.59845534099999753 ) ) ;
#13136=CARTESIAN_POINT ( 'NONE',  ( -6.665307709260000379, -111.0000000000000000, -13.13558364449999871 ) ) ;
#13137=EDGE_CURVE ( 'NONE', #4936, #7956, #3190, .T. ) ;
#13140=CARTESIAN_POINT ( 'NONE',  ( 0.000000000000000000, -111.0000000000000000, 0.000000000000000000 ) ) ;
#13143=EDGE_CURVE ( 'NONE', #11541, #22767, #27399, .T. ) ;
#13144=CIRCLE ( 'NONE', #14985, 13.13304743849999845 ) ;
#13145=CARTESIAN_POINT ( 'NONE',  ( -12.58496709408010972, -100.9229461901620937, -10.77194485367771826 ) ) ;
#13150=EDGE_CURVE ( 'NONE', #7636, #19075, #27481, .T. ) ;
#13151=CARTESIAN_POINT ( 'NONE',  ( -1.241004412070000118, -101.0848057460000007, -15.36253221559999993 ) ) ;
#13155=CARTESIAN_POINT ( 'NONE',  ( -14.89765609740000052, -101.1045759049999901, 4.404014004990000508 ) ) ;
#13157=CARTESIAN_POINT ( 'NONE',  ( 16.24020105036429484, -94.68293928641202228, 17.23415085847014083 ) ) ;
#13158=DIRECTION ( 'NONE',  ( 0.000000000000000000, 1.000000000000000000, 0.000000000000000000 ) ) ;
#13161=B_SPLINE_CURVE_WITH_KNOTS ( 'NONE', 3,
 ( #4013, #19739, #17564, #26315, #3736, #12738, #19328, #15065, #23976, #24265, #28070, #12595, #21787, #25884, #26024, #12871, #6491 ),
 .UNSPECIFIED., .F., .F.,
 ( 4, 2, 2, 1, 1, 1, 1, 1, 2, 2, 4 ),
 ( 0.000000000000000000, 0.2499999999999857336, 0.3749999999999782396, 0.4374999999999752420, 0.4687499999999737987, 0.4843749999999718558, 0.4921874999999703570, 0.4960937499999696909, 0.4980468749999701905, 0.4999999999999706901, 1.000000000000000000 ),
 .UNSPECIFIED. ) ;
#13163=FACE_OUTER_BOUND ( 'NONE', #22244, .T. ) ;
#13165=DIRECTION ( 'NONE',  ( 0.000000000000000000, -1.000000000000000000, 0.000000000000000000 ) ) ;
#13166=CARTESIAN_POINT ( 'NONE',  ( 24.95011738624632613, -93.41743724467393406, 11.71896984693396604 ) ) ;
#13168=DIRECTION ( 'NONE',  ( -0.000000000000000000, 1.000000000000000000, 0.000000000000000000 ) ) ;
#13172=CARTESIAN_POINT ( 'NONE',  ( -23.85439607509999860, -94.57749572790000059, -4.067360661330000404 ) ) ;
#13177=CARTESIAN_POINT ( 'NONE',  ( 16.20958609349999691, -100.4071172650000108, 4.379827211240000295 ) ) ;
#13181=CARTESIAN_POINT ( 'NONE',  ( 11.70455088819999823, -93.00000000000000000, 8.942783294160001617 ) ) ;
#13185=CARTESIAN_POINT ( 'NONE',  ( 0.6601778629024529499, -99.57060688035245732, -17.35471282991112574 ) ) ;
#13191=CARTESIAN_POINT ( 'NONE',  ( -17.05590440810569675, -97.60610394651996558, 10.26113453133471154 ) ) ;
#13195=CARTESIAN_POINT ( 'NONE',  ( -11.91096112960000042, -101.1700440390000040, -9.606277335259999717 ) ) ;
#13199=B_SPLINE_CURVE_WITH_KNOTS ( 'NONE', 3,
 ( #6703, #12794, #9016, #21995, #19651, #21702, #1751, #10593, #1899, #19511, #19939, #15258, #24179, #28395, #2043, #10886, #26227, #17335, #8431, #15117, #12, #19796, #28675, #6254, #8708, #24029, #4064, #8859, #28543, #17625, #26511, #4365, #22883 ),
 .UNSPECIFIED., .F., .F.,
 ( 4, 2, 1, 1, 2, 2, 1, 1, 1, 2, 2, 2, 1, 1, 2, 2, 1, 1, 2, 2, 4 ),
 ( 0.000000000000000000, 0.06250000000002318978, 0.09375000000002295386, 0.1093750000000323352, 0.1171875000000370259, 0.1250000000000417166, 0.1875000000000381362, 0.2187500000000363598, 0.2343750000000414946, 0.2421875000000440759, 0.2500000000000466294, 0.3750000000000206501, 0.4375000000000118794, 0.4687500000000074385, 0.4843750000000081601, 0.5000000000000087708, 0.6250000000000012212, 0.6874999999999975575, 0.7187499999999973355, 0.7499999999999971134, 1.000000000000000000 ),
 .UNSPECIFIED. ) ;
#13204=DIRECTION ( 'NONE',  ( 0.000000000000000000, 1.000000000000000000, 0.000000000000000000 ) ) ;
#13206=DIRECTION ( 'NONE',  ( -0.7320471826101231372, 0.000000000000000000, 0.6812539338841141490 ) ) ;
#13208=CARTESIAN_POINT ( 'NONE',  ( 12.03625741000000104, -92.92010097569999516, 27.59856934729999978 ) ) ;
#13209=VERTEX_POINT ( 'NONE', #21987 ) ;
#13212=TOROIDAL_SURFACE ( 'NONE', #3486, 15.50000000000000000, 0.5000000000000000000 ) ;
#13214=CARTESIAN_POINT ( 'NONE',  ( 24.09844107120000345, -93.07154584180000256, 12.17654209520000030 ) ) ;
#13215=CARTESIAN_POINT ( 'NONE',  ( -15.21246488650000117, -100.9405327639999967, 4.776672761669999545 ) ) ;
#13219=AXIS2_PLACEMENT_3D ( 'NONE', #18152, #701, #2722 ) ;
#13220=CARTESIAN_POINT ( 'NONE',  ( 12.39757656149999931, -101.6484611540000031, -10.11435096289999969 ) ) ;
#13225=CARTESIAN_POINT ( 'NONE',  ( 12.97071070920000047, -101.3090757639999993, -9.810351643989998038 ) ) ;
#13231=CARTESIAN_POINT ( 'NONE',  ( -6.296318341739999269, -102.8486084350000027, -11.52533341650000054 ) ) ;
#13235=CARTESIAN_POINT ( 'NONE',  ( 1.723886190540000030, -92.49999926799999628, -29.27157131740000295 ) ) ;
#13237=DIRECTION ( 'NONE',  ( 0.000000000000000000, 1.000000000000000000, 0.000000000000000000 ) ) ;
#13244=CARTESIAN_POINT ( 'NONE',  ( 19.14326094509999976, -98.26007807750001177, -0.6345988924250000052 ) ) ;
#13246=EDGE_LOOP ( 'NONE', ( #13608, #11996, #4989, #435 ) ) ;
#13247=LINE ( 'NONE', #20255, #27508 ) ;
#13249=EDGE_LOOP ( 'NONE', ( #8079, #8564, #987, #6454 ) ) ;
#13252=DIRECTION ( 'NONE',  ( 0.000000000000000000, -1.000000000000000000, 0.000000000000000000 ) ) ;
#13254=DIRECTION ( 'NONE',  ( 0.000000000000000000, 1.000000000000000000, 0.000000000000000000 ) ) ;
#13258=CARTESIAN_POINT ( 'NONE',  ( 10.49047732170000025, -92.65509162889999573, -25.64082967920000300 ) ) ;
#13264=CARTESIAN_POINT ( 'NONE',  ( -17.96353918029999974, -93.86098520749999352, 18.31830939139999970 ) ) ;
#13268=CARTESIAN_POINT ( 'NONE',  ( 0.7855938671740000379, -100.2511768809999921, -16.66646386170000227 ) ) ;
#13273=EDGE_CURVE ( 'NONE', #139, #23006, #7836, .T. ) ;
#13274=LINE ( 'NONE', #24365, #12448 ) ;
#13276=EDGE_CURVE ( 'NONE', #15187, #23314, #8284, .T. ) ;
#13280=CARTESIAN_POINT ( 'NONE',  ( 28.25594642106975130, -92.69183043804710564, 11.48302245628102192 ) ) ;
#13290=CARTESIAN_POINT ( 'NONE',  ( -13.12737311083959568, -100.1240332945601779, -11.11848609902146201 ) ) ;
#13291=ORIENTED_EDGE ( 'NONE', *, *, #21202, .F. ) ;
#13293=CARTESIAN_POINT ( 'NONE',  ( 26.79489351000000141, -92.68584525839999344, -12.41053404230000190 ) ) ;
#13294=CARTESIAN_POINT ( 'NONE',  ( 8.708727887559998493, -98.58239820560001476, 16.48836518959999964 ) ) ;
#13296=CARTESIAN_POINT ( 'NONE',  ( -0.5455003419149999644, -98.53908914310000000, -18.73905742539999864 ) ) ;
#13297=CARTESIAN_POINT ( 'NONE',  ( 14.28478035945855140, -92.50000000000000000, 26.94835746195996862 ) ) ;
#13299=CARTESIAN_POINT ( 'NONE',  ( 11.45697295529999948, -101.0535396030000044, -10.57669106610000220 ) ) ;
#13301=DIRECTION ( 'NONE',  ( 1.000000000000000000, 0.000000000000000000, 0.000000000000000000 ) ) ;
#13305=DIRECTION ( 'NONE',  ( 0.000000000000000000, -1.000000000000000000, 0.000000000000000000 ) ) ;
#13306=CARTESIAN_POINT ( 'NONE',  ( 27.32142465356705330, -93.09721478964854668, 9.756329643219576297 ) ) ;
#13308=ADVANCED_FACE ( 'NONE', ( #2323 ), #18051, .T. ) ;
#13311=CARTESIAN_POINT ( 'NONE',  ( 7.889779489369998622, -101.3196660750000149, 13.95717439989999953 ) ) ;
#13316=CARTESIAN_POINT ( 'NONE',  ( -24.00581540240000322, -94.71481161159999829, -4.132755290490000455 ) ) ;
#13319=VERTEX_POINT ( 'NONE', #9006 ) ;
#13320=CARTESIAN_POINT ( 'NONE',  ( -6.285925807789999986, -101.6484611540000031, 14.71350185169999847 ) ) ;
#13328=CARTESIAN_POINT ( 'NONE',  ( 24.20411630889999799, -92.55031878719999838, -15.29912012159999968 ) ) ;
#13330=CARTESIAN_POINT ( 'NONE',  ( 17.60755106127235692, -95.57586274903817980, 14.14554066879750671 ) ) ;
#13331=CARTESIAN_POINT ( 'NONE',  ( 14.08191940870000103, -97.83383802260000550, -14.15749693589999758 ) ) ;
#13335=CARTESIAN_POINT ( 'NONE',  ( -12.00964495180000036, -100.4731125450000064, -10.87550195419999888 ) ) ;
#13336=CARTESIAN_POINT ( 'NONE',  ( 0.000000000000000000, -92.50000000000000000, 0.000000000000000000 ) ) ;
#13340=ADVANCED_FACE ( 'NONE', ( #4799 ), #25534, .F. ) ;
#13344=ORIENTED_EDGE ( 'NONE', *, *, #13819, .F. ) ;
#13345=CIRCLE ( 'NONE', #25021, 0.4999999999999991118 ) ;
#13347=TOROIDAL_SURFACE ( 'NONE', #15205, 21.14285714289999873, 0.5000000000000000000 ) ;
#13351=DIRECTION ( 'NONE',  ( 0.000000000000000000, 1.000000000000000000, 0.000000000000000000 ) ) ;
#13355=CARTESIAN_POINT ( 'NONE',  ( 21.86954465750000054, -93.60791045439999891, 13.04854595950000018 ) ) ;
#13356=DIRECTION ( 'NONE',  ( 1.000000000000000000, 0.000000000000000000, 0.000000000000000000 ) ) ;
#13358=CARTESIAN_POINT ( 'NONE',  ( 16.58537890990000108, -94.98812477769999418, 16.93952572510000110 ) ) ;
#13363=CARTESIAN_POINT ( 'NONE',  ( -18.79536340909999836, -92.66001714109999909, -20.78146695779999931 ) ) ;
#13364=FACE_OUTER_BOUND ( 'NONE', #23017, .T. ) ;
#13366=CARTESIAN_POINT ( 'NONE',  ( -1.228311966399999955, -101.1461874320000049, -16.11255545180000226 ) ) ;
#13370=CARTESIAN_POINT ( 'NONE',  ( -5.069308693793000309, -98.61679376083424131, -19.10643818412435024 ) ) ;
#13379=CARTESIAN_POINT ( 'NONE',  ( -23.81726931088821786, -92.83865970263468625, -19.05223594286923117 ) ) ;
#13381=CARTESIAN_POINT ( 'NONE',  ( 22.60879290213893711, -95.55433702443635013, -0.3969505341440314194 ) ) ;
#13388=CARTESIAN_POINT ( 'NONE',  ( 15.50925568500000118, -100.9197081840000010, 1.894556133100000039 ) ) ;
#13389=ORIENTED_EDGE ( 'NONE', *, *, #23278, .T. ) ;
#13394=CARTESIAN_POINT ( 'NONE',  ( 13.43278536909999943, -96.09419472199999745, 17.29930431160000026 ) ) ;
#13396=EDGE_CURVE ( 'NONE', #3543, #21689, #10130, .T. ) ;
#13398=CARTESIAN_POINT ( 'NONE',  ( 9.374849361280000792, -94.98812477599999227, -22.63660904189999812 ) ) ;
#13400=CARTESIAN_POINT ( 'NONE',  ( -16.97872427700000131, -99.83167715590001023, 3.440838554449999531 ) ) ;
#13401=CARTESIAN_POINT ( 'NONE',  ( -29.74393970790053388, -92.83160374581187568, 6.748930471038662837 ) ) ;
#13403=ORIENTED_EDGE ( 'NONE', *, *, #21286, .F. ) ;
#13408=CARTESIAN_POINT ( 'NONE',  ( -12.80006882320263450, -92.59055325462904307, 27.68408069405598226 ) ) ;
#13414=ORIENTED_EDGE ( 'NONE', *, *, #13776, .T. ) ;
#13416=CARTESIAN_POINT ( 'NONE',  ( -23.32456840009999866, -92.51542729400000553, -18.96923773310000172 ) ) ;
#13417=CARTESIAN_POINT ( 'NONE',  ( 0.6800711189380000965, -100.1459902240000019, -16.94139632559999953 ) ) ;
#13424=ORIENTED_EDGE ( 'NONE', *, *, #5792, .T. ) ;
#13431=CARTESIAN_POINT ( 'NONE',  ( 23.27561534246691011, -92.52048598158071968, -19.71030172176314821 ) ) ;
#13434=CARTESIAN_POINT ( 'NONE',  ( -6.842114547430000471, -101.1030539030000028, 13.83820396960000032 ) ) ;
#13439=EDGE_CURVE ( 'NONE', #2729, #9504, #5525, .T. ) ;
#13440=CARTESIAN_POINT ( 'NONE',  ( 6.944463756510000252, -99.57787269160000676, 15.90826982280000124 ) ) ;
#13442=CARTESIAN_POINT ( 'NONE',  ( -7.441474119920000518, -94.70873613630000420, -22.49466058249999989 ) ) ;
#13443=AXIS2_PLACEMENT_3D ( 'NONE', #6824, #15687, #13356 ) ;
#13444=CARTESIAN_POINT ( 'NONE',  ( -20.00661640924422713, -92.56492639285779944, -23.02161043673221030 ) ) ;
#13447=CARTESIAN_POINT ( 'NONE',  ( -14.86197080470000209, -100.8869818489999943, 4.957595453540000641 ) ) ;
#13449=CARTESIAN_POINT ( 'NONE',  ( -13.46646228700000059, -101.3150700380000018, -9.098096927170001180 ) ) ;
#13450=EDGE_CURVE ( 'NONE', #15112, #1700, #26445, .T. ) ;
#13457=CARTESIAN_POINT ( 'NONE',  ( 24.33166760675546314, -93.00000237470422348, -17.52085307207648412 ) ) ;
#13458=CARTESIAN_POINT ( 'NONE',  ( 28.86890114233755966, -93.00000237470419506, 8.099190551483227196 ) ) ;
#13463=DIRECTION ( 'NONE',  ( 0.000000000000000000, -1.000000000000000000, 0.000000000000000000 ) ) ;
#13465=CARTESIAN_POINT ( 'NONE',  ( -23.50862730440000092, -94.59276292120000562, -3.692480652049999978 ) ) ;
#13468=AXIS2_PLACEMENT_3D ( 'NONE', #16582, #20970, #27534 ) ;
#13470=ORIENTED_EDGE ( 'NONE', *, *, #14230, .T. ) ;
#13475=CARTESIAN_POINT ( 'NONE',  ( 8.182334915651470197, -92.59033770621367410, 29.38229076648032034 ) ) ;
#13481=EDGE_CURVE ( 'NONE', #8693, #28264, #19459, .T. ) ;
#13483=CARTESIAN_POINT ( 'NONE',  ( 8.188637977920000921, -100.9197082849999987, 13.30686163390000054 ) ) ;
#13484=CARTESIAN_POINT ( 'NONE',  ( -16.10081869210645422, -99.27453212434828345, 7.470651185126897076 ) ) ;
#13487=CARTESIAN_POINT ( 'NONE',  ( -5.873418876839999747, -101.3150700380000018, 15.15334698740000086 ) ) ;
#13488=CARTESIAN_POINT ( 'NONE',  ( -12.94893854829999924, -100.3063911739999980, -11.10051843049999931 ) ) ;
#13490=AXIS2_PLACEMENT_3D ( 'NONE', #22891, #18658, #16018 ) ;
#13491=CARTESIAN_POINT ( 'NONE',  ( 10.65740927894239753, -97.98442063578340822, 16.78772980300869833 ) ) ;
#13492=ORIENTED_EDGE ( 'NONE', *, *, #18563, .F. ) ;
#13495=ORIENTED_EDGE ( 'NONE', *, *, #1537, .F. ) ;
#13498=CARTESIAN_POINT ( 'NONE',  ( -18.05296197569739647, -94.57749224628196316, 16.11416072503950048 ) ) ;
#13502=CARTESIAN_POINT ( 'NONE',  ( 21.75610509370000045, -93.65023659739999573, 12.77706960399999936 ) ) ;
#13503=CARTESIAN_POINT ( 'NONE',  ( -15.03194159329999913, -100.8816813800000034, 4.847769557329999479 ) ) ;
#13506=CARTESIAN_POINT ( 'NONE',  ( 16.42966103859999905, -94.59276292389999696, 17.21499949629999904 ) ) ;
#13509=EDGE_CURVE ( 'NONE', #16619, #8693, #11047, .T. ) ;
#13511=CARTESIAN_POINT ( 'NONE',  ( 0.000000000000000000, -101.6484611540000031, 0.000000000000000000 ) ) ;
#13513=CARTESIAN_POINT ( 'NONE',  ( -14.04043131989999971, -93.59856727309998803, -21.14276827349999976 ) ) ;
#13514=CARTESIAN_POINT ( 'NONE',  ( -23.55554542814485686, -94.54719627017709627, -3.773182801408312415 ) ) ;
#13518=CARTESIAN_POINT ( 'NONE',  ( -5.963907253145354304, -101.5019029710834673, 14.96613752057661806 ) ) ;
#13521=DIRECTION ( 'NONE',  ( 0.000000000000000000, 1.000000000000000000, 0.000000000000000000 ) ) ;
#13522=DIRECTION ( 'NONE',  ( 0.3186522097941134612, 0.000000000000000000, 0.9478717050283378409 ) ) ;
#13526=CARTESIAN_POINT ( 'NONE',  ( -7.441474466189999859, -94.70873790539999959, -22.49465953780000049 ) ) ;
#13528=CARTESIAN_POINT ( 'NONE',  ( -24.14169972247601237, -92.59055325465111252, -18.63943186536354091 ) ) ;
#13531=AXIS2_PLACEMENT_3D ( 'NONE', #19432, #3852, #1678 ) ;
#13532=CARTESIAN_POINT ( 'NONE',  ( -14.59972664311643697, -101.2126522312630925, 4.393265484499556450 ) ) ;
#13535=ADVANCED_FACE ( 'NONE', ( #14120 ), #407, .F. ) ;
#13540=EDGE_LOOP ( 'NONE', ( #23630, #1676, #21926, #24645 ) ) ;
#13541=FACE_OUTER_BOUND ( 'NONE', #23558, .T. ) ;
#13544=CYLINDRICAL_SURFACE ( 'NONE', #17, 0.7999999999999997113 ) ;
#13546=CARTESIAN_POINT ( 'NONE',  ( 16.46460143819999900, -94.70873611929999925, 17.03825138000000194 ) ) ;
#13549=CARTESIAN_POINT ( 'NONE',  ( 5.341700292228932057, -93.31462968041127226, -27.40505522819004369 ) ) ;
#13552=DIRECTION ( 'NONE',  ( -0.7436828042389490578, 0.000000000000000000, 0.6685326369589542628 ) ) ;
#13556=TOROIDAL_SURFACE ( 'NONE', #7074, 18.14285714289999873, 0.5000000000000000000 ) ;
#13557=FACE_OUTER_BOUND ( 'NONE', #22556, .T. ) ;
#13562=DIRECTION ( 'NONE',  ( -0.2162432783070589171, 0.000000000000000000, -0.9763395129702657771 ) ) ;
#13563=CARTESIAN_POINT ( 'NONE',  ( -16.50487832609999828, -92.86540159979999487, 21.47928501360000197 ) ) ;
#13564=FACE_OUTER_BOUND ( 'NONE', #3283, .T. ) ;
#13566=CARTESIAN_POINT ( 'NONE',  ( -3.215510237749999778, -94.59276292389999696, 23.57860181210000405 ) ) ;
#13567=CARTESIAN_POINT ( 'NONE',  ( 0.6844652716010000137, -99.85455315880000171, -17.12311058819999943 ) ) ;
#13572=EDGE_CURVE ( 'NONE', #1013, #17518, #16688, .T. ) ;
#13578=CARTESIAN_POINT ( 'NONE',  ( 27.75131065520946905, -92.50000000000000000, 12.65403630604174445 ) ) ;
#13579=CARTESIAN_POINT ( 'NONE',  ( 27.05591625959999647, -111.0000000000000000, 12.64646362319999895 ) ) ;
#13580=CARTESIAN_POINT ( 'NONE',  ( 14.78884388380000026, -96.96081173790000207, 14.87954162810000014 ) ) ;
#13581=ORIENTED_EDGE ( 'NONE', *, *, #25839, .F. ) ;
#13582=CARTESIAN_POINT ( 'NONE',  ( 23.42046525251764422, -92.54938211474758702, -19.53815701032223728 ) ) ;
#13583=CARTESIAN_POINT ( 'NONE',  ( 20.51721167730000062, -93.01584738759999027, 16.65400869639999826 ) ) ;
#13584=B_SPLINE_SURFACE_WITH_KNOTS ( 'NONE', 5, 5, ( 
 ( #6412, #15277, #4231, #13106, #22018, #25826 ),
 ( #10904, #8729, #11502, #9032, #16031, #17938 ),
 ( #22753, #19959, #15882, #24936, #7165, #9324 ),
 ( #22608, #7016, #17791, #9174, #2651, #4965 ),
 ( #629, #18079, #4522, #2351, #20410, #13850 ),
 ( #6721, #18228, #26528, #15432, #13400, #2796 ) ),
 .UNSPECIFIED., .F., .F., .F.,
 ( 6, 6 ),
 ( 6, 6 ),
 ( 21.64530111450000049, 36.61382091400000149 ),
 ( 0.000000000000000000, 0.5000000000000000000 ),
 .UNSPECIFIED. ) ;
#13586=CARTESIAN_POINT ( 'NONE',  ( -7.197000385329999972, -101.3878691800000098, 14.40505143829999923 ) ) ;
#13593=CARTESIAN_POINT ( 'NONE',  ( -0.6930209439279999550, -101.1411470200000053, -15.37361599470000151 ) ) ;
#13599=ORIENTED_EDGE ( 'NONE', *, *, #5122, .T. ) ;
#13600=CARTESIAN_POINT ( 'NONE',  ( -21.30003612899999865, -93.00000000000000000, -21.83021898440000186 ) ) ;
#13601=CARTESIAN_POINT ( 'NONE',  ( 12.74020478277715185, -96.39729796470680867, 17.27646218270080425 ) ) ;
#13602=DIRECTION ( 'NONE',  ( 0.000000000000000000, 1.000000000000000000, 0.000000000000000000 ) ) ;
#13607=CARTESIAN_POINT ( 'NONE',  ( 24.76102720923304901, -93.45279863481047755, 11.84977757016969591 ) ) ;
#13608=ORIENTED_EDGE ( 'NONE', *, *, #19452, .T. ) ;
#13609=CARTESIAN_POINT ( 'NONE',  ( -29.75227628095127841, -92.87422005961224158, 6.712099127441182311 ) ) ;
#13615=VECTOR ( 'NONE', #11721, 1000.000000000000000 ) ;
#13619=CARTESIAN_POINT ( 'NONE',  ( 14.28941763439999946, -92.50000000000000000, -3.575252188409999921 ) ) ;
#13621=CARTESIAN_POINT ( 'NONE',  ( 16.76553128029999939, -99.61736775859999682, 4.445700604479999818 ) ) ;
#13623=B_SPLINE_CURVE_WITH_KNOTS ( 'NONE', 3,
 ( #15883, #20411, #25506, #12635, #7872, #25790 ),
 .UNSPECIFIED., .F., .F.,
 ( 4, 2, 4 ),
 ( 0.000000000000000000, 0.5000000000000000000, 1.000000000000000000 ),
 .UNSPECIFIED. ) ;
#13626=CARTESIAN_POINT ( 'NONE',  ( -17.86977837739999941, -98.51736893809999174, -8.245718314579999486 ) ) ;
#13627=ORIENTED_EDGE ( 'NONE', *, *, #27357, .F. ) ;
#13637=CARTESIAN_POINT ( 'NONE',  ( -17.53021419299614081, -96.09436528054369830, 13.05496988638304146 ) ) ;
#13640=CARTESIAN_POINT ( 'NONE',  ( -3.132411190821024149, -98.07566646228944762, 20.23086237361857442 ) ) ;
#13641=CARTESIAN_POINT ( 'NONE',  ( -12.87349974830000043, -99.74726900420000675, -11.33951603419999898 ) ) ;
#13646=CARTESIAN_POINT ( 'NONE',  ( 26.66370566908554096, -92.65976904079786891, -14.80868499793449722 ) ) ;
#13651=CARTESIAN_POINT ( 'NONE',  ( 6.962669195700001090, -93.00000450890000536, -28.64060852350000275 ) ) ;
#13653=CARTESIAN_POINT ( 'NONE',  ( -0.5784133371710000748, -95.70830610519999482, 22.47961678780000128 ) ) ;
#13654=CARTESIAN_POINT ( 'NONE',  ( 11.26661192880000151, -92.54721911629999909, 27.31814187710000041 ) ) ;
#13656=ORIENTED_EDGE ( 'NONE', *, *, #24509, .T. ) ;
#13661=CARTESIAN_POINT ( 'NONE',  ( 20.37436807119999926, -94.16701182180001695, 13.61303751910000059 ) ) ;
#13667=CARTESIAN_POINT ( 'NONE',  ( 12.41906884210000150, -101.3138676899999950, -9.951096275919999457 ) ) ;
#13668=CARTESIAN_POINT ( 'NONE',  ( -13.31557542770000069, -94.15497152580000773, -21.58932584709999958 ) ) ;
#13672=CARTESIAN_POINT ( 'NONE',  ( -16.77203540500000045, -99.85754733859999988, 2.755720534169999958 ) ) ;
#13683=CARTESIAN_POINT ( 'NONE',  ( 16.26822356142537629, -100.5798851022435940, 4.341841719661410970 ) ) ;
#13689=CARTESIAN_POINT ( 'NONE',  ( -14.63416202187712933, -101.1297513861017450, 4.643748334617020745 ) ) ;
#13693=DIRECTION ( 'NONE',  ( 0.000000000000000000, 1.000000000000000000, 0.000000000000000000 ) ) ;
#13694=CARTESIAN_POINT ( 'NONE',  ( 12.80450217360000131, -93.00000000000000000, 27.55316291459999789 ) ) ;
#13701=DIRECTION ( 'NONE',  ( 0.000000000000000000, -1.000000000000000000, 0.000000000000000000 ) ) ;
#13703=CARTESIAN_POINT ( 'NONE',  ( 16.42966247209999864, -94.59276292389999696, 17.21499781270000184 ) ) ;
#13704=CARTESIAN_POINT ( 'NONE',  ( 3.432129155885089489, -93.09721478922745064, -28.80740708133247452 ) ) ;
#13711=CARTESIAN_POINT ( 'NONE',  ( 10.18254802899999945, -92.87437365140000622, -25.45365413509999897 ) ) ;
#13713=CARTESIAN_POINT ( 'NONE',  ( -12.28514971879595663, -92.50630337894784816, 27.91669684123871775 ) ) ;
#13714=ORIENTED_EDGE ( 'NONE', *, *, #12030, .F. ) ;
#13715=VECTOR ( 'NONE', #13204, 1000.000000000000000 ) ;
#13719=EDGE_LOOP ( 'NONE', ( #27937, #3631, #14736, #3569 ) ) ;
#13720=CARTESIAN_POINT ( 'NONE',  ( -17.69156363009999922, -96.95584349610000174, 11.12533346610000073 ) ) ;
#13721=CIRCLE ( 'NONE', #28150, 0.7500000000000006661 ) ;
#13727=DIRECTION ( 'NONE',  ( 0.000000000000000000, 1.000000000000000000, 0.000000000000000000 ) ) ;
#13731=DIRECTION ( 'NONE',  ( 1.000000000000000000, 0.000000000000000000, 0.000000000000000000 ) ) ;
#13732=AXIS2_PLACEMENT_3D ( 'NONE', #9924, #14310, #3256 ) ;
#13736=CARTESIAN_POINT ( 'NONE',  ( 23.76344434241608283, -92.71346081468576017, -19.11932852845460573 ) ) ;
#13737=CARTESIAN_POINT ( 'NONE',  ( 22.54710945800000133, -93.01085527750001347, 15.53951536520000154 ) ) ;
#13739=CARTESIAN_POINT ( 'NONE',  ( -7.338479256380000315, -100.8772072149999985, 13.99320739510000067 ) ) ;
#13741=CARTESIAN_POINT ( 'NONE',  ( -12.48888858376851907, -101.5829753080983977, -10.08195492097721058 ) ) ;
#13745=CARTESIAN_POINT ( 'NONE',  ( 7.437117725900000309, -99.39747163819998832, 16.00091516599999864 ) ) ;
#13748=FACE_OUTER_BOUND ( 'NONE', #19962, .T. ) ;
#13750=CARTESIAN_POINT ( 'NONE',  ( 11.63343413870000020, -100.9405348700000076, -10.90407401050000047 ) ) ;
#13757=CARTESIAN_POINT ( 'NONE',  ( 6.867289776849999861, -93.00000000000000000, 29.52484619129999643 ) ) ;
#13758=CYLINDRICAL_SURFACE ( 'NONE', #12238, 16.00000000000000000 ) ;
#13761=EDGE_CURVE ( 'NONE', #23006, #19757, #20414, .T. ) ;
#13764=FACE_OUTER_BOUND ( 'NONE', #15150, .T. ) ;
#13765=CARTESIAN_POINT ( 'NONE',  ( -18.75664408842720121, -92.68584073461859418, 22.80736226812994261 ) ) ;
#13766=CARTESIAN_POINT ( 'NONE',  ( 21.02256860540000005, -93.91547409650000588, 13.07290323880000038 ) ) ;
#13771=CARTESIAN_POINT ( 'NONE',  ( -15.33123009060000008, -99.55619081909999579, -8.401006626490000073 ) ) ;
#13773=CARTESIAN_POINT ( 'NONE',  ( 9.134356845928596869, -92.82529299096876230, 29.10006078398899021 ) ) ;
#13775=DIRECTION ( 'NONE',  ( 1.000000000000000000, 0.000000000000000000, 0.000000000000000000 ) ) ;
#13776=EDGE_CURVE ( 'NONE', #22228, #18774, #16346, .T. ) ;
#13782=CARTESIAN_POINT ( 'NONE',  ( 13.81099964959999937, -99.92967428129999519, -10.51862844640000105 ) ) ;
#13785=CARTESIAN_POINT ( 'NONE',  ( -3.463941484895344480, -98.37417905842463028, 19.78189371439013300 ) ) ;
#13786=CARTESIAN_POINT ( 'NONE',  ( 7.724131721144110507, -101.6290295230935499, 14.02868979977465358 ) ) ;
#13790=ORIENTED_EDGE ( 'NONE', *, *, #10305, .F. ) ;
#13791=CARTESIAN_POINT ( 'NONE',  ( 26.82487458483781850, -92.59033770622828285, -14.51536147898519857 ) ) ;
#13794=DIRECTION ( 'NONE',  ( -0.7529607911047507818, 0.000000000000000000, 0.6580653820547832655 ) ) ;
#13796=CARTESIAN_POINT ( 'NONE',  ( 11.27094287870000144, -92.51078253369999516, 27.07599673740000057 ) ) ;
#13799=ORIENTED_EDGE ( 'NONE', *, *, #14850, .T. ) ;
#13801=CARTESIAN_POINT ( 'NONE',  ( -17.85148316769999965, -92.81180222680001179, -20.73234325470000172 ) ) ;
#13805=CARTESIAN_POINT ( 'NONE',  ( -11.32307664120000013, -101.1889999979999999, 9.421136869679999748 ) ) ;
#13807=CARTESIAN_POINT ( 'NONE',  ( 7.412091288878791318, -101.1586403914945151, 13.76842333336193924 ) ) ;
#13810=CARTESIAN_POINT ( 'NONE',  ( -11.71096586250000016, -94.52293239719999463, -20.87032883819999896 ) ) ;
#13812=ORIENTED_EDGE ( 'NONE', *, *, #15649, .F. ) ;
#13815=CARTESIAN_POINT ( 'NONE',  ( 13.77380425289999977, -99.99711545080000974, -10.25584394120000020 ) ) ;
#13819=EDGE_CURVE ( 'NONE', #8764, #22228, #19753, .T. ) ;
#13820=CARTESIAN_POINT ( 'NONE',  ( 0.8834120860809999698, -100.8023006570000035, -15.75170354469999978 ) ) ;
#13824=CARTESIAN_POINT ( 'NONE',  ( -11.84764024939999949, -93.03217248389999838, -23.86222728849999797 ) ) ;
#13825=CARTESIAN_POINT ( 'NONE',  ( 23.56065605869999757, -94.89197151660000884, -2.367189373290000010 ) ) ;
#13827=CARTESIAN_POINT ( 'NONE',  ( 15.82012184412321787, -101.2111896145381280, 4.085987896871170477 ) ) ;
#13831=CARTESIAN_POINT ( 'NONE',  ( -14.64568814080000081, -101.2530993010000060, 4.044604232330000215 ) ) ;
#13839=VERTEX_POINT ( 'NONE', #22395 ) ;
#13848=CARTESIAN_POINT ( 'NONE',  ( 8.373915991510450851, -94.27895761501838479, -24.15545878555541748 ) ) ;
#13850=CARTESIAN_POINT ( 'NONE',  ( -18.00122845199999944, -98.93440624740000544, 5.015517834929999808 ) ) ;
#13853=EDGE_LOOP ( 'NONE', ( #28248, #4188, #1393, #11178 ) ) ;
#13858=EDGE_LOOP ( 'NONE', ( #2303, #16872, #28784, #17131 ) ) ;
#13862=EDGE_LOOP ( 'NONE', ( #9121, #14163, #8259, #7645 ) ) ;
#13863=EDGE_CURVE ( 'NONE', #14760, #25977, #22279, .T. ) ;
#13865=CARTESIAN_POINT ( 'NONE',  ( -17.50501298330000211, -97.01468531680001206, 11.19299372800000114 ) ) ;
#13871=AXIS2_PLACEMENT_3D ( 'NONE', #17813, #26703, #28711 ) ;
#13875=CARTESIAN_POINT ( 'NONE',  ( 12.41281216700000023, -98.24303092559999584, 14.67252853509999966 ) ) ;
#13876=ORIENTED_EDGE ( 'NONE', *, *, #10145, .T. ) ;
#13877=CARTESIAN_POINT ( 'NONE',  ( 23.00372540730000281, -92.50000000000000000, -20.02694728079999820 ) ) ;
#13878=FACE_OUTER_BOUND ( 'NONE', #6262, .T. ) ;
#13881=CARTESIAN_POINT ( 'NONE',  ( -7.374356127060000432, -100.8685038539999965, 13.89626452919999977 ) ) ;
#13883=CARTESIAN_POINT ( 'NONE',  ( 3.976803427850000183, -92.99999854809999533, 28.21756021889999744 ) ) ;
#13887=CARTESIAN_POINT ( 'NONE',  ( 7.629218925470000023, -101.5342894280000081, 14.06592359269999903 ) ) ;
#13890=CARTESIAN_POINT ( 'NONE',  ( 8.882943487429999507, -98.83600327540000308, 16.35256359799999970 ) ) ;
#13892=CARTESIAN_POINT ( 'NONE',  ( 0.5588920821209999446, -99.64579499010000063, -17.31215308460000202 ) ) ;
#13894=CARTESIAN_POINT ( 'NONE',  ( 11.86104588439999930, -101.2306315440000049, -11.05401200120000027 ) ) ;
#13896=B_SPLINE_CURVE_WITH_KNOTS ( 'NONE', 3,
 ( #27679, #27944, #7718, #14117, #16870, #25759, #25479, #14529, #9874, #7980 ),
 .UNSPECIFIED., .F., .F.,
 ( 4, 2, 2, 2, 4 ),
 ( 0.000000000000000000, 0.2500000000000000000, 0.5000000000000000000, 0.7500000000000000000, 1.000000000000000000 ),
 .UNSPECIFIED. ) ;
#13897=CARTESIAN_POINT ( 'NONE',  ( 12.79340726668418959, -96.37047651198221843, 17.28024789624581814 ) ) ;
#13905=AXIS2_PLACEMENT_3D ( 'NONE', #17732, #274, #4466 ) ;
#13907=CARTESIAN_POINT ( 'NONE',  ( 7.030727077140000780, -101.5369810359999860, 14.37272453779999992 ) ) ;
#13909=CARTESIAN_POINT ( 'NONE',  ( 8.099920077730001111, -100.8733989549999990, 13.47813240850000049 ) ) ;
#13916=FACE_OUTER_BOUND ( 'NONE', #3480, .T. ) ;
#13918=VERTEX_POINT ( 'NONE', #15668 ) ;
#13921=CARTESIAN_POINT ( 'NONE',  ( -15.31473116159999925, -99.60591459030000294, -8.206551967759999400 ) ) ;
#13922=ORIENTED_EDGE ( 'NONE', *, *, #25889, .T. ) ;
#13923=CARTESIAN_POINT ( 'NONE',  ( -30.49520906449999913, -92.50000000000000000, 0.5405775709410000074 ) ) ;
#13930=CARTESIAN_POINT ( 'NONE',  ( 23.25682987829999959, -94.57749572790000059, -6.685469233060000072 ) ) ;
#13932=DIRECTION ( 'NONE',  ( 0.000000000000000000, -1.000000000000000000, 0.000000000000000000 ) ) ;
#13937=CARTESIAN_POINT ( 'NONE',  ( -12.56556452559999926, -99.92384627689999377, -11.31794108169999902 ) ) ;
#13938=CARTESIAN_POINT ( 'NONE',  ( -12.29363612059999866, -101.2530993000000024, -8.928690578620001261 ) ) ;
#13939=CARTESIAN_POINT ( 'NONE',  ( 15.54119309900000090, -100.8869817940000075, 1.981729577500000339 ) ) ;
#13942=CARTESIAN_POINT ( 'NONE',  ( 26.94827291246611622, -92.54893169919635909, -14.28427949690044052 ) ) ;
#13948=CARTESIAN_POINT ( 'NONE',  ( -3.732180049640000163, -98.24302442990000372, 18.85290869059999963 ) ) ;
#13949=CARTESIAN_POINT ( 'NONE',  ( 10.50529330130000005, -92.86738811510001312, 27.55314313410000082 ) ) ;
#13952=CARTESIAN_POINT ( 'NONE',  ( -22.83021220420000219, -92.50000647099999185, -19.05479008140000374 ) ) ;
#13954=ORIENTED_EDGE ( 'NONE', *, *, #13396, .F. ) ;
#13955=DIRECTION ( 'NONE',  ( 0.6285074900730002190, 0.000000000000000000, -0.7778035323410003032 ) ) ;
#13957=CARTESIAN_POINT ( 'NONE',  ( -11.25325031930000108, -94.84397446139999488, -20.59894429220000234 ) ) ;
#13966=CARTESIAN_POINT ( 'NONE',  ( -30.49520906449999913, -92.50000000000000000, 0.5405775709410000074 ) ) ;
#13968=DIRECTION ( 'NONE',  ( 0.9773425350887455787, 0.000000000000000000, 0.2116638115179453050 ) ) ;
#13970=CARTESIAN_POINT ( 'NONE',  ( 23.65724685329999843, -92.50000647099999185, -18.01772143370000023 ) ) ;
#13972=CARTESIAN_POINT ( 'NONE',  ( -9.594728507420001051, -93.84506351590000861, -23.13300608200000141 ) ) ;
#13975=CARTESIAN_POINT ( 'NONE',  ( 16.80289107651169189, -99.96200787837224766, 4.259014394836682982 ) ) ;
#13986=EDGE_CURVE ( 'NONE', #24255, #20007, #18098, .T. ) ;
#13989=DIRECTION ( 'NONE',  ( 0.000000000000000000, 1.000000000000000000, 0.000000000000000000 ) ) ;
#13997=CARTESIAN_POINT ( 'NONE',  ( 2.407211674977468352, -93.02765837720274078, -29.45082399442910770 ) ) ;
#13999=CARTESIAN_POINT ( 'NONE',  ( -13.13595842799045066, -101.5839620086842672, -9.219410581145925931 ) ) ;
#14000=CARTESIAN_POINT ( 'NONE',  ( -5.417927868154690074, -95.55433702422656950, -21.95361345762339411 ) ) ;
#14006=ORIENTED_EDGE ( 'NONE', *, *, #5122, .F. ) ;
#14008=CARTESIAN_POINT ( 'NONE',  ( -12.61948338259999858, -101.6484611540000031, -9.836088610590000059 ) ) ;
#14012=CARTESIAN_POINT ( 'NONE',  ( -3.055530165179999980, -94.70873790529999781, 23.49572270359999848 ) ) ;
#14014=DIRECTION ( 'NONE',  ( 0.000000000000000000, 1.000000000000000000, 0.000000000000000000 ) ) ;
#14019=EDGE_LOOP ( 'NONE', ( #7805, #7705, #17043, #4510 ) ) ;
#14023=CARTESIAN_POINT ( 'NONE',  ( 17.53803339859999966, -96.16784812509999369, 14.96109425939999937 ) ) ;
#14031=LINE ( 'NONE', #10064, #5607 ) ;
#14033=CARTESIAN_POINT ( 'NONE',  ( -10.66266547438723578, -93.83956660848620857, -23.27634539248033008 ) ) ;
#14036=CARTESIAN_POINT ( 'NONE',  ( 7.620081227840000082, -101.5353651350000064, 14.07009485169999863 ) ) ;
#14037=VERTEX_POINT ( 'NONE', #14235 ) ;
#14040=CARTESIAN_POINT ( 'NONE',  ( 11.97116049530000126, -98.43722211939999056, -15.53505339789999873 ) ) ;
#14043=FACE_OUTER_BOUND ( 'NONE', #28116, .T. ) ;
#14045=CARTESIAN_POINT ( 'NONE',  ( 13.35125805077294281, -96.09071899285407881, 17.31197431996907810 ) ) ;
#14047=DIRECTION ( 'NONE',  ( 1.000000000000000000, 0.000000000000000000, 0.000000000000000000 ) ) ;
#14051=AXIS2_PLACEMENT_3D ( 'NONE', #9488, #2213, #6735 ) ;
#14054=CARTESIAN_POINT ( 'NONE',  ( 6.638042613879999720, -101.0956037589999994, 14.05630584859999921 ) ) ;
#14055=CARTESIAN_POINT ( 'NONE',  ( 14.01548305848342935, -98.16872836011999937, -13.77740321380717248 ) ) ;
#14059=CYLINDRICAL_SURFACE ( 'NONE', #1083, 20.64285714289999163 ) ;
#14067=ORIENTED_EDGE ( 'NONE', *, *, #9868, .T. ) ;
#14068=CARTESIAN_POINT ( 'NONE',  ( 8.097647218569999694, -101.1461874760000086, 13.98396581760000146 ) ) ;
#14071=VECTOR ( 'NONE', #28753, 1000.000000000000000 ) ;
#14072=CARTESIAN_POINT ( 'NONE',  ( -4.636291350829999812E-13, -101.6484611540000031, 1.074695887839999887E-13 ) ) ;
#14073=ORIENTED_EDGE ( 'NONE', *, *, #25266, .F. ) ;
#14074=CARTESIAN_POINT ( 'NONE',  ( 0.4613846910555384762, -101.2145573445051241, -16.33011699766660030 ) ) ;
#14079=CARTESIAN_POINT ( 'NONE',  ( -4.790709198910000133, -98.40794110039999509, -18.33800208579999946 ) ) ;
#14080=CARTESIAN_POINT ( 'NONE',  ( 14.26399793470000077, -97.58045781620000980, -14.03566137740000208 ) ) ;
#14087=CARTESIAN_POINT ( 'NONE',  ( 16.08037952269999948, -101.3150705500000157, 2.354224216990000063 ) ) ;
#14088=ORIENTED_EDGE ( 'NONE', *, *, #11030, .F. ) ;
#14089=AXIS2_PLACEMENT_3D ( 'NONE', #2329, #8857, #11181 ) ;
#14096=CARTESIAN_POINT ( 'NONE',  ( -0.7643172187030000675, -95.76596938490000355, 22.73307493400000112 ) ) ;
#14098=CARTESIAN_POINT ( 'NONE',  ( 2.785942070970000461, -93.82249895229999481, 24.67684871370000010 ) ) ;
#14099=EDGE_LOOP ( 'NONE', ( #14477, #2644, #24943, #11950 ) ) ;
#14102=CARTESIAN_POINT ( 'NONE',  ( -28.84886582594137749, -93.09721478952320695, 3.064172615184945769 ) ) ;
#14103=CARTESIAN_POINT ( 'NONE',  ( 3.787197165510000296, -91.50000000000000000, -30.26395773239999798 ) ) ;
#14108=DIRECTION ( 'NONE',  ( 0.000000000000000000, -1.000000000000000000, 0.000000000000000000 ) ) ;
#14112=DIRECTION ( 'NONE',  ( 0.000000000000000000, -1.000000000000000000, 0.000000000000000000 ) ) ;
#14113=ORIENTED_EDGE ( 'NONE', *, *, #7012, .F. ) ;
#14115=CARTESIAN_POINT ( 'NONE',  ( -16.79027416539999962, -100.2529091920000042, 3.234199557169999739 ) ) ;
#14117=CARTESIAN_POINT ( 'NONE',  ( -6.105915352247367700, -101.1416252791428434, 14.29215036881257994 ) ) ;
#14120=FACE_OUTER_BOUND ( 'NONE', #6632, .T. ) ;
#14122=CARTESIAN_POINT ( 'NONE',  ( -7.920105797075711607, -100.1585711159093535, 15.24014698975379112 ) ) ;
#14128=CARTESIAN_POINT ( 'NONE',  ( 15.87518046294259655, -101.1248211537865700, 4.142658035507630565 ) ) ;
#14137=VERTEX_POINT ( 'NONE', #3305 ) ;
#14139=CARTESIAN_POINT ( 'NONE',  ( 22.95301417039999592, -94.52293512109999085, -6.773259939029999899 ) ) ;
#14147=CIRCLE ( 'NONE', #28106, 30.50000000000000000 ) ;
#14148=FACE_OUTER_BOUND ( 'NONE', #1940, .T. ) ;
#14151=CARTESIAN_POINT ( 'NONE',  ( -2.004269379255393613, -97.53591929645209291, -19.96958644832030316 ) ) ;
#14156=CARTESIAN_POINT ( 'NONE',  ( 15.99006255310108493, -101.4218099524899657, 2.411354960305282180 ) ) ;
#14158=CARTESIAN_POINT ( 'NONE',  ( -12.03627366839999802, -92.50000000000000000, 28.02459841239999960 ) ) ;
#14161=CARTESIAN_POINT ( 'NONE',  ( -12.13775690249999961, -101.1411470200000053, -9.460613307739999200 ) ) ;
#14163=ORIENTED_EDGE ( 'NONE', *, *, #14568, .F. ) ;
#14164=ADVANCED_FACE ( 'NONE', ( #28188 ), #20912, .F. ) ;
#14165=CARTESIAN_POINT ( 'NONE',  ( -17.36676170379999817, -98.30606121530000507, 8.776474676399999453 ) ) ;
#14167=CARTESIAN_POINT ( 'NONE',  ( -0.1779554536940000098, -111.0000000000000000, -15.99901033990000165 ) ) ;
#14171=CIRCLE ( 'NONE', #15524, 30.50000000000000000 ) ;
#14183=CARTESIAN_POINT ( 'NONE',  ( -11.85289063449999958, -94.98812477599999227, -21.44324726029999795 ) ) ;
#14185=CIRCLE ( 'NONE', #4880, 0.8000000000000000444 ) ;
#14187=CARTESIAN_POINT ( 'NONE',  ( 7.491713480479999632, -101.1706547440000037, 13.83665357419999964 ) ) ;
#14190=CARTESIAN_POINT ( 'NONE',  ( -29.47186158120000243, -92.84292488370000740, -0.4149714379639999895 ) ) ;
#14193=ORIENTED_EDGE ( 'NONE', *, *, #11193, .F. ) ;
#14196=EDGE_CURVE ( 'NONE', #20007, #14226, #16699, .T. ) ;
#14202=CARTESIAN_POINT ( 'NONE',  ( 11.90208458877192932, -101.5703832412493455, -10.78058033292013640 ) ) ;
#14207=ORIENTED_EDGE ( 'NONE', *, *, #25763, .T. ) ;
#14209=CARTESIAN_POINT ( 'NONE',  ( 6.789115400040000026, -101.1417990620000040, 14.22050701429999897 ) ) ;
#14212=CARTESIAN_POINT ( 'NONE',  ( 7.462391103660000802, -101.2375126459999848, 13.25959037569999843 ) ) ;
#14213=CARTESIAN_POINT ( 'NONE',  ( -11.17107965319999963, -94.77693780670000478, -20.89252829639999831 ) ) ;
#14215=CARTESIAN_POINT ( 'NONE',  ( 11.70455088819999823, -101.1889999979999999, 8.942783294160001617 ) ) ;
#14219=CARTESIAN_POINT ( 'NONE',  ( -20.57686592631715072, -93.08494709825977509, -20.57755909579458375 ) ) ;
#14221=ORIENTED_EDGE ( 'NONE', *, *, #14963, .F. ) ;
#14223=CARTESIAN_POINT ( 'NONE',  ( -15.54410891719999910, -99.75094652210000845, -8.801109042589999376 ) ) ;
#14226=VERTEX_POINT ( 'NONE', #19438 ) ;
#14227=CARTESIAN_POINT ( 'NONE',  ( 0.5404583983271005199, -100.1994045927584693, -17.13382711562018201 ) ) ;
#14230=EDGE_CURVE ( 'NONE', #13209, #11679, #17052, .T. ) ;
#14233=CARTESIAN_POINT ( 'NONE',  ( 0.000000000000000000, -111.0000000000000000, 0.000000000000000000 ) ) ;
#14234=CARTESIAN_POINT ( 'NONE',  ( 23.86725312652073683, -92.82709422631835139, -18.98958227918895147 ) ) ;
#14235=CARTESIAN_POINT ( 'NONE',  ( -1.283023294879999998, -101.3150694429999987, -16.20107482390000087 ) ) ;
#14238=DIRECTION ( 'NONE',  ( 1.000000000000000000, 0.000000000000000000, 0.000000000000000000 ) ) ;
#14243=CARTESIAN_POINT ( 'NONE',  ( -3.641088133819999850, -98.26007808079999961, 18.80451095879999812 ) ) ;
#14244=CARTESIAN_POINT ( 'NONE',  ( 10.51100516569999854, -92.56539259249998963, 27.27496703559999958 ) ) ;
#14246=CARTESIAN_POINT ( 'NONE',  ( -28.69446774251560939, -93.12686943463702960, 2.652929931884275838 ) ) ;
#14249=EDGE_LOOP ( 'NONE', ( #20400, #15038, #2900, #2017 ) ) ;
#14256=ORIENTED_EDGE ( 'NONE', *, *, #1002, .F. ) ;
#14258=EDGE_CURVE ( 'NONE', #1054, #23896, #14286, .T. ) ;
#14259=CARTESIAN_POINT ( 'NONE',  ( -16.51010518360000034, -100.0706250509999933, 2.778373719329999769 ) ) ;
#14265=CARTESIAN_POINT ( 'NONE',  ( -7.918607114148264792, -100.1240332945198759, 15.27233837034834529 ) ) ;
#14268=CARTESIAN_POINT ( 'NONE',  ( 0.000000000000000000, -90.50000000000000000, 0.000000000000000000 ) ) ;
#14270=CARTESIAN_POINT ( 'NONE',  ( 15.91717527196672854, -101.0610180774675371, 4.179821879114435035 ) ) ;
#14275=CARTESIAN_POINT ( 'NONE',  ( 9.630000870221753217, -93.08383529948000046, 27.46986062684589669 ) ) ;
#14282=CARTESIAN_POINT ( 'NONE',  ( -6.158276018989999656, -101.3256027080000052, 14.66656444329999864 ) ) ;
#14286=B_SPLINE_CURVE_WITH_KNOTS ( 'NONE', 5,
 ( #21218, #25869, #16981, #14646, #23674, #10108, #16840, #25729, #15332 ),
 .UNSPECIFIED., .F., .F.,
 ( 6, 3, 6 ),
 ( 0.000000000000000000, 0.5000000000000000000, 1.000000000000000000 ),
 .UNSPECIFIED. ) ;
#14287=CARTESIAN_POINT ( 'NONE',  ( 0.000000000000000000, -92.50000000000000000, 29.91857981989999971 ) ) ;
#14293=CARTESIAN_POINT ( 'NONE',  ( 12.94734957360000038, -94.70873790539999959, -19.84316983170000270 ) ) ;
#14298=CARTESIAN_POINT ( 'NONE',  ( 13.78600338218322818, -95.55433702442398669, -17.92376068152854529 ) ) ;
#14300=ORIENTED_EDGE ( 'NONE', *, *, #21606, .T. ) ;
#14301=EDGE_CURVE ( 'NONE', #1715, #17343, #5059, .T. ) ;
#14302=DIRECTION ( 'NONE',  ( 0.4396719266362648648, 0.000000000000000000, -0.8981584475625418174 ) ) ;
#14307=CONICAL_SURFACE ( 'NONE', #6379, 13.13304743849999667, 0.9119902906770002149 ) ;
#14310=DIRECTION ( 'NONE',  ( 0.000000000000000000, -1.000000000000000000, 0.000000000000000000 ) ) ;
#14315=ORIENTED_EDGE ( 'NONE', *, *, #13439, .T. ) ;
#14316=CARTESIAN_POINT ( 'NONE',  ( -13.16239993169999956, -100.8816835080000089, -8.729908192910000864 ) ) ;
#14319=CARTESIAN_POINT ( 'NONE',  ( 6.153538985549999119, -93.00000450890000536, 28.82528036289999918 ) ) ;
#14322=CARTESIAN_POINT ( 'NONE',  ( 7.307353180730000730, -101.1411471079999984, 13.54367522859999973 ) ) ;
#14326=FACE_OUTER_BOUND ( 'NONE', #24191, .T. ) ;
#14328=CARTESIAN_POINT ( 'NONE',  ( 11.54254854999999935, -98.24302442830000359, -15.36655156750000017 ) ) ;
#14335=AXIS2_PLACEMENT_3D ( 'NONE', #28221, #23298, #21530 ) ;
#14340=ORIENTED_EDGE ( 'NONE', *, *, #589, .F. ) ;
#14341=CARTESIAN_POINT ( 'NONE',  ( 6.615597047280000531, -101.2530993010000060, 13.67879707989999893 ) ) ;
#14342=CARTESIAN_POINT ( 'NONE',  ( 12.82422237299999956, -94.98812477769999418, -19.93894812050000098 ) ) ;
#14343=CARTESIAN_POINT ( 'NONE',  ( 7.521915565509999624, -101.1193270250000040, 13.57310074129999933 ) ) ;
#14345=CARTESIAN_POINT ( 'NONE',  ( -11.76876610979999960, -94.80026829410000744, -21.40432538299999976 ) ) ;
#14362=CARTESIAN_POINT ( 'NONE',  ( 0.5870844549389877542, -100.3617719035924978, -17.00173476966439878 ) ) ;
#14363=CARTESIAN_POINT ( 'NONE',  ( 6.615597047280000531, -101.2530993010000060, 13.67879707989999893 ) ) ;
#14369=DIRECTION ( 'NONE',  ( 1.000000000000000000, 0.000000000000000000, 0.000000000000000000 ) ) ;
#14370=CARTESIAN_POINT ( 'NONE',  ( 14.09492607880000037, -96.58372172939999700, -15.97495134070000056 ) ) ;
#14377=FACE_OUTER_BOUND ( 'NONE', #12570, .T. ) ;
#14381=DIRECTION ( 'NONE',  ( 0.000000000000000000, 1.000000000000000000, 0.000000000000000000 ) ) ;
#14382=CARTESIAN_POINT ( 'NONE',  ( -28.44519471329999760, -92.55031878709998239, 3.282258450510000092 ) ) ;
#14386=EDGE_CURVE ( 'NONE', #13209, #17197, #20904, .T. ) ;
#14388=CIRCLE ( 'NONE', #26958, 1.000000000000000444 ) ;
#14389=CARTESIAN_POINT ( 'NONE',  ( -28.91764959275750257, -93.08494709829881231, 3.257743348587014420 ) ) ;
#14397=DIRECTION ( 'NONE',  ( 0.3799696139668880535, 0.000000000000000000, -0.9249989688977248159 ) ) ;
#14398=CARTESIAN_POINT ( 'NONE',  ( -15.56430586970000007, -100.7823373549999957, 2.734376720570000252 ) ) ;
#14407=AXIS2_PLACEMENT_3D ( 'NONE', #24882, #4918, #13794 ) ;
#14409=DIRECTION ( 'NONE',  ( 1.000000000000000000, 0.000000000000000000, 0.000000000000000000 ) ) ;
#14411=CARTESIAN_POINT ( 'NONE',  ( 19.57843399940000140, -94.59276292389999696, 13.52682119470000011 ) ) ;
#14412=ORIENTED_EDGE ( 'NONE', *, *, #18953, .T. ) ;
#14414=EDGE_CURVE ( 'NONE', #19113, #21973, #6258, .T. ) ;
#14419=ORIENTED_EDGE ( 'NONE', *, *, #26187, .F. ) ;
#14429=FACE_OUTER_BOUND ( 'NONE', #13540, .T. ) ;
#14430=CARTESIAN_POINT ( 'NONE',  ( -13.55845375110000006, -93.00000046469999404, 27.19007892950000027 ) ) ;
#14433=CARTESIAN_POINT ( 'NONE',  ( 15.76736775957732206, -101.6407018583229274, 2.752252931809222147 ) ) ;
#14439=ORIENTED_EDGE ( 'NONE', *, *, #27562, .F. ) ;
#14448=ORIENTED_EDGE ( 'NONE', *, *, #16156, .T. ) ;
#14452=CARTESIAN_POINT ( 'NONE',  ( 27.05591625959999647, -93.00000000000000000, 12.64646362319999895 ) ) ;
#14456=CARTESIAN_POINT ( 'NONE',  ( -13.14229091329999832, -100.8869817940000075, -8.528547626079999944 ) ) ;
#14461=CARTESIAN_POINT ( 'NONE',  ( -13.55845375110000006, -93.00000046469999404, 27.19007892950000027 ) ) ;
#14462=CARTESIAN_POINT ( 'NONE',  ( 7.218659600080000516, -101.2530993709999905, 13.36960380829999906 ) ) ;
#14466=CARTESIAN_POINT ( 'NONE',  ( -27.05658671429999984, -93.01085527740001169, -4.217795407459999701 ) ) ;
#14467=CARTESIAN_POINT ( 'NONE',  ( 10.55213757090000115, -95.76596938280000870, -20.15016797799999893 ) ) ;
#14471=CARTESIAN_POINT ( 'NONE',  ( -18.11129459295214517, -92.54383083955173106, 24.54040303195527173 ) ) ;
#14475=CARTESIAN_POINT ( 'NONE',  ( 13.82853744383082351, -98.09459741723881621, 15.06191675743312608 ) ) ;
#14477=ORIENTED_EDGE ( 'NONE', *, *, #22923, .F. ) ;
#14478=CARTESIAN_POINT ( 'NONE',  ( 6.715091161579999302, -101.1180794200000008, 13.99142704490000177 ) ) ;
#14481=AXIS2_PLACEMENT_3D ( 'NONE', #5358, #18765, #25180 ) ;
#14483=CARTESIAN_POINT ( 'NONE',  ( -11.47583862359999962, -94.67274582490000512, -20.72942797039999974 ) ) ;
#14489=DIRECTION ( 'NONE',  ( 0.000000000000000000, 1.000000000000000000, 0.000000000000000000 ) ) ;
#14490=DIRECTION ( 'NONE',  ( 0.000000000000000000, -1.000000000000000000, 0.000000000000000000 ) ) ;
#14493=CARTESIAN_POINT ( 'NONE',  ( 0.5331203104650162894, -101.0610180774177138, -16.44819632410123589 ) ) ;
#14495=CARTESIAN_POINT ( 'NONE',  ( 6.038481244350000665, -100.8023006570000035, 14.57509264930000015 ) ) ;
#14496=CARTESIAN_POINT ( 'NONE',  ( 13.58333658430973756, -92.61393927545320537, 27.30833405384957757 ) ) ;
#14497=AXIS2_PLACEMENT_3D ( 'NONE', #19644, #23888, #26359 ) ;
#14498=CARTESIAN_POINT ( 'NONE',  ( 15.67714813079999736, -101.1412505549999992, 3.951871014550000005 ) ) ;
#14504=CARTESIAN_POINT ( 'NONE',  ( -0.2819570041572871943, -95.90275867845988955, 23.35952539960409169 ) ) ;
#14510=ORIENTED_EDGE ( 'NONE', *, *, #7639, .T. ) ;
#14514=B_SPLINE_CURVE_WITH_KNOTS ( 'NONE', 3,
 ( #24271, #13185, #28770, #26605, #18007, #552 ),
 .UNSPECIFIED., .F., .F.,
 ( 4, 2, 4 ),
 ( 0.000000000000000000, 0.5000000000000000000, 1.000000000000000000 ),
 .UNSPECIFIED. ) ;
#14519=ORIENTED_EDGE ( 'NONE', *, *, #8628, .T. ) ;
#14523=CARTESIAN_POINT ( 'NONE',  ( 26.62478236560000155, -92.85282594270000800, -10.14810411050000027 ) ) ;
#14526=CARTESIAN_POINT ( 'NONE',  ( -14.90965166979999879, -101.1292387920000095, 4.262398319349999909 ) ) ;
#14527=CARTESIAN_POINT ( 'NONE',  ( -16.50888742379999741, -100.1721652129999995, 2.973064930670000106 ) ) ;
#14529=CARTESIAN_POINT ( 'NONE',  ( -6.275498632237177077, -101.4628082233731732, 14.68909490417829211 ) ) ;
#14530=ORIENTED_EDGE ( 'NONE', *, *, #3378, .T. ) ;
#14540=CARTESIAN_POINT ( 'NONE',  ( 19.89027988503224265, -94.80026864431334843, 14.17835479305916202 ) ) ;
#14545=CARTESIAN_POINT ( 'NONE',  ( 7.146599689825861468, -99.96200787832681556, 15.79248128130144835 ) ) ;
#14548=CARTESIAN_POINT ( 'NONE',  ( -18.30346299744424954, -98.29032200027317856, 5.174493964400173951 ) ) ;
#14551=CARTESIAN_POINT ( 'NONE',  ( 28.34114226579999851, -92.53610955750001210, 8.350028085840000003 ) ) ;
#14552=CARTESIAN_POINT ( 'NONE',  ( -6.091317750690000032, -101.3957169669999985, 14.78042619649999878 ) ) ;
#14562=CARTESIAN_POINT ( 'NONE',  ( -18.81329003759999807, -96.93384555689999615, -9.961933200989999904 ) ) ;
#14568=EDGE_CURVE ( 'NONE', #9504, #4936, #2768, .T. ) ;
#14577=ADVANCED_FACE ( 'NONE', ( #13557 ), #11975, .F. ) ;
#14579=AXIS2_PLACEMENT_3D ( 'NONE', #23005, #877, #5367 ) ;
#14585=CIRCLE ( 'NONE', #6694, 4.999999999999999112 ) ;
#14587=CARTESIAN_POINT ( 'NONE',  ( 6.998258279363821721, -92.73901256244006674, -28.68106635605278498 ) ) ;
#14589=CARTESIAN_POINT ( 'NONE',  ( -13.01247235640000000, -101.5369810359999860, -9.310661355180000598 ) ) ;
#14591=CARTESIAN_POINT ( 'NONE',  ( -7.888947276530000607, -100.3517545579999961, 14.77732780220000031 ) ) ;
#14592=CARTESIAN_POINT ( 'NONE',  ( -0.2283560652399999891, -93.01584738779999384, 26.42460660340000089 ) ) ;
#14595=CARTESIAN_POINT ( 'NONE',  ( 7.273173879219999804, -101.1845941320000009, 13.44072509259999926 ) ) ;
#14597=DIRECTION ( 'NONE',  ( 0.4794255386042041156, 0.000000000000000000, 0.8775825618903722036 ) ) ;
#14598=DIRECTION ( 'NONE',  ( 1.000000000000000000, 0.000000000000000000, 0.000000000000000000 ) ) ;
#14603=CARTESIAN_POINT ( 'NONE',  ( 12.02399834240000054, -101.4254868729999970, -10.50861765550000015 ) ) ;
#14606=CARTESIAN_POINT ( 'NONE',  ( -18.15215127219713764, -92.53708507728566701, 24.51021966657489060 ) ) ;
#14609=AXIS2_PLACEMENT_3D ( 'NONE', #23332, #14977, #24175 ) ;
#14610=CARTESIAN_POINT ( 'NONE',  ( 14.28941763439999946, -93.00000000000000000, -3.575252188409999921 ) ) ;
#14612=ADVANCED_FACE ( 'NONE', ( #18821 ), #23189, .F. ) ;
#14613=CARTESIAN_POINT ( 'NONE',  ( -0.1699704075889999777, -101.1848541609999899, -15.28111812279999882 ) ) ;
#14615=CARTESIAN_POINT ( 'NONE',  ( 15.41249585359999941, -101.0535396030000044, 2.362963133130000060 ) ) ;
#14619=CARTESIAN_POINT ( 'NONE',  ( 6.555554406829999792, -100.6809449770000100, 15.07230642660000086 ) ) ;
#14621=CARTESIAN_POINT ( 'NONE',  ( -11.43284111409999859, -94.65020208389999823, -20.93784837230000306 ) ) ;
#14625=CARTESIAN_POINT ( 'NONE',  ( -7.879418878250000091, -99.92967428129999519, 15.46932493210000104 ) ) ;
#14627=CARTESIAN_POINT ( 'NONE',  ( 8.080976620399999533, -94.09272382160000348, -24.58537356260000095 ) ) ;
#14631=ORIENTED_EDGE ( 'NONE', *, *, #14301, .F. ) ;
#14632=VECTOR ( 'NONE', #17975, 1000.000000000000000 ) ;
#14638=CARTESIAN_POINT ( 'NONE',  ( 0.4072779472236851550, -101.3038909013372262, -16.26179699871198636 ) ) ;
#14640=CARTESIAN_POINT ( 'NONE',  ( -13.12430501772102254, -92.94830743985350807, -23.71755625844523863 ) ) ;
#14646=CARTESIAN_POINT ( 'NONE',  ( 11.43994069400000058, -100.8816835080000089, -10.88980376029999952 ) ) ;
#14648=CARTESIAN_POINT ( 'NONE',  ( 16.83483077069999823, -99.92967571559999840, 4.239603657359999112 ) ) ;
#14653=ORIENTED_EDGE ( 'NONE', *, *, #26485, .T. ) ;
#14657=FACE_OUTER_BOUND ( 'NONE', #1312, .T. ) ;
#14663=ORIENTED_EDGE ( 'NONE', *, *, #20609, .T. ) ;
#14666=ADVANCED_FACE ( 'NONE', ( #5949 ), #7102, .T. ) ;
#14669=CARTESIAN_POINT ( 'NONE',  ( -15.40337430839999833, -101.5317003319999998, 4.643717924509999762 ) ) ;
#14670=CARTESIAN_POINT ( 'NONE',  ( -16.72188147059999963, -99.89426761010000178, 2.874729616160000223 ) ) ;
#14674=CARTESIAN_POINT ( 'NONE',  ( 20.42065948455764257, -98.07566645793311011, -1.447915294044073375 ) ) ;
#14677=CARTESIAN_POINT ( 'NONE',  ( -11.77049175740000209, -94.59276292389999696, -20.68200892780000189 ) ) ;
#14687=CARTESIAN_POINT ( 'NONE',  ( -18.46601579710593555, -98.10212143905430082, 5.492879491436290174 ) ) ;
#14689=CARTESIAN_POINT ( 'NONE',  ( 27.34475978920000117, -92.65997674700000175, 9.666848034470000073 ) ) ;
#14693=CARTESIAN_POINT ( 'NONE',  ( 12.69294339169999830, -100.9137139110000021, -9.125620792290000338 ) ) ;
#14696=ORIENTED_EDGE ( 'NONE', *, *, #17406, .F. ) ;
#14699=EDGE_CURVE ( 'NONE', #2955, #14037, #19765, .T. ) ;
#14700=CARTESIAN_POINT ( 'NONE',  ( 8.171241461239999770E-14, -101.6484611540000031, -6.927791673659999887E-14 ) ) ;
#14703=EDGE_CURVE ( 'NONE', #9479, #7740, #7966, .T. ) ;
#14705=CARTESIAN_POINT ( 'NONE',  ( 15.84942546552125009, -101.5703832412493597, 2.583842542799739128 ) ) ;
#14706=CARTESIAN_POINT ( 'NONE',  ( -20.16709992299999854, -93.01085577540001736, 18.52401656639999672 ) ) ;
#14707=CARTESIAN_POINT ( 'NONE',  ( 24.17069834520000171, -93.81709628040000837, -8.947401651030000735 ) ) ;
#14713=DIRECTION ( 'NONE',  ( 0.000000000000000000, 1.000000000000000000, 0.000000000000000000 ) ) ;
#14714=CARTESIAN_POINT ( 'NONE',  ( 0.000000000000000000, -107.1975888269999899, 0.000000000000000000 ) ) ;
#14715=CARTESIAN_POINT ( 'NONE',  ( -23.77081188420000046, -93.00000000000000000, -19.11016751280000037 ) ) ;
#14720=ORIENTED_EDGE ( 'NONE', *, *, #941, .T. ) ;
#14723=CARTESIAN_POINT ( 'NONE',  ( 7.206351956654603264, -92.50000267097107098, -28.91782128996979750 ) ) ;
#14725=CARTESIAN_POINT ( 'NONE',  ( -12.94585355969999974, -101.6484611540000031, -9.402386697529999893 ) ) ;
#14727=CARTESIAN_POINT ( 'NONE',  ( -16.08621294430000148, -93.02865658550000205, -23.59017073649999929 ) ) ;
#14728=CARTESIAN_POINT ( 'NONE',  ( -1.381300513170000022, -100.8816824760000088, -15.73378836020000016 ) ) ;
#14730=CARTESIAN_POINT ( 'NONE',  ( 11.67392084060484869, -98.28141829054760592, -16.48995336470006734 ) ) ;
#14731=ORIENTED_EDGE ( 'NONE', *, *, #3160, .F. ) ;
#14733=CARTESIAN_POINT ( 'NONE',  ( 13.05823860876455633, -101.2111896145002419, -9.821097530008616516 ) ) ;
#14734=CARTESIAN_POINT ( 'NONE',  ( -22.27192494970000070, -94.59276479679999738, -8.381614403809997782 ) ) ;
#14736=ORIENTED_EDGE ( 'NONE', *, *, #20948, .T. ) ;
#14740=CARTESIAN_POINT ( 'NONE',  ( -18.07483010357461595, -92.55017404142755311, 24.56726588061794203 ) ) ;
#14744=CARTESIAN_POINT ( 'NONE',  ( 26.78710329588840366, -92.73901256241863678, -12.41089373421818465 ) ) ;
#14747=ORIENTED_EDGE ( 'NONE', *, *, #15642, .F. ) ;
#14748=CARTESIAN_POINT ( 'NONE',  ( 6.364863104659999493, -100.8772072149999985, 14.46207622220000033 ) ) ;
#14749=CARTESIAN_POINT ( 'NONE',  ( -13.91416830965637885, -92.72284173551921072, -24.03918013284343402 ) ) ;
#14750=B_SPLINE_CURVE_WITH_KNOTS ( 'NONE', 5,
 ( #4230, #15881, #8876, #26978, #11042, #22017, #6864, #9173, #2064 ),
 .UNSPECIFIED., .F., .F.,
 ( 6, 3, 6 ),
 ( 0.000000000000000000, 0.5000000000000000000, 1.000000000000000000 ),
 .UNSPECIFIED. ) ;
#14752=CARTESIAN_POINT ( 'NONE',  ( 4.403302820470730516, -92.82334897395796247, -30.18047277449198162 ) ) ;
#14753=CARTESIAN_POINT ( 'NONE',  ( -6.858700158590000484, -97.53592492849999473, 18.86158608849999752 ) ) ;
#14754=CARTESIAN_POINT ( 'NONE',  ( 8.578180688210000682, -94.24983875559999547, -23.91258280499999955 ) ) ;
#14755=DIRECTION ( 'NONE',  ( 0.000000000000000000, 1.000000000000000000, 0.000000000000000000 ) ) ;
#14760=VERTEX_POINT ( 'NONE', #11325 ) ;
#14762=CARTESIAN_POINT ( 'NONE',  ( -16.99615325119999909, -99.69348474340000621, 3.341833029000000010 ) ) ;
#14764=ORIENTED_EDGE ( 'NONE', *, *, #19493, .T. ) ;
#14766=CARTESIAN_POINT ( 'NONE',  ( -0.9248989260280000568, -101.3957169669999985, -15.95962757919999753 ) ) ;
#14771=DIRECTION ( 'NONE',  ( 1.000000000000000000, 0.000000000000000000, 0.000000000000000000 ) ) ;
#14785=CARTESIAN_POINT ( 'NONE',  ( -29.21843977289999827, -92.50000942380000879, 6.434612924249999644 ) ) ;
#14786=CARTESIAN_POINT ( 'NONE',  ( -0.7205257404357856554, -101.5555610555564812, -15.98376809946171129 ) ) ;
#14787=EDGE_CURVE ( 'NONE', #25061, #3132, #5087, .T. ) ;
#14791=DIRECTION ( 'NONE',  ( 0.4794255386042040601, 0.000000000000000000, 0.8775825618903720926 ) ) ;
#14792=VERTEX_POINT ( 'NONE', #17907 ) ;
#14795=AXIS2_PLACEMENT_3D ( 'NONE', #11620, #18492, #13968 ) ;
#14802=ORIENTED_EDGE ( 'NONE', *, *, #25132, .T. ) ;
#14805=CARTESIAN_POINT ( 'NONE',  ( -12.46510431380000128, -101.3138676899999950, -9.893369620240001439 ) ) ;
#14807=CARTESIAN_POINT ( 'NONE',  ( -7.339513061798150773, -101.3846248973262618, 14.44658188679844102 ) ) ;
#14809=FACE_OUTER_BOUND ( 'NONE', #15425, .T. ) ;
#14810=CYLINDRICAL_SURFACE ( 'NONE', #14335, 0.8000000000000005995 ) ;
#14812=ORIENTED_EDGE ( 'NONE', *, *, #7253, .F. ) ;
#14819=ORIENTED_EDGE ( 'NONE', *, *, #295, .T. ) ;
#14820=CARTESIAN_POINT ( 'NONE',  ( 26.25071228570000059, -93.07694010310001431, 10.86079363670000042 ) ) ;
#14831=TOROIDAL_SURFACE ( 'NONE', #6942, 15.50000000000000000, 0.5000000000000000000 ) ;
#14833=CARTESIAN_POINT ( 'NONE',  ( -16.89577420600000224, -97.73638926269998706, -10.62153989119999942 ) ) ;
#14834=CARTESIAN_POINT ( 'NONE',  ( 12.22678147189999898, -101.0956037589999994, -9.599435331940000538 ) ) ;
#14836=CARTESIAN_POINT ( 'NONE',  ( 24.69157579510000033, -92.76550115769998683, -13.71735200580000047 ) ) ;
#14843=B_SPLINE_CURVE_WITH_KNOTS ( 'NONE', 5,
 ( #25862, #27906, #7947, #7684, #1403, #14495, #10246, #23395, #5753, #7543, #14363, #5474 ),
 .UNSPECIFIED., .F., .F.,
 ( 6, 3, 3, 6 ),
 ( 0.000000000000000000, 0.4964111757630880195, 0.7833083924342724158, 1.000000000000000000 ),
 .UNSPECIFIED. ) ;
#14847=CARTESIAN_POINT ( 'NONE',  ( -7.879410208250000380, -99.92967571559999840, 15.46934584979999983 ) ) ;
#14848=EDGE_CURVE ( 'NONE', #5829, #13319, #4622, .T. ) ;
#14850=EDGE_CURVE ( 'NONE', #3921, #13319, #2472, .T. ) ;
#14854=CARTESIAN_POINT ( 'NONE',  ( 11.70455088819999823, -93.00000000000000000, 8.942783294160001617 ) ) ;
#14859=CARTESIAN_POINT ( 'NONE',  ( 12.00742146600000204, -96.90532602029999509, 17.10694051450000330 ) ) ;
#14860=CARTESIAN_POINT ( 'NONE',  ( -8.303419408699999948, -99.91102932029998840, 14.75134094139999874 ) ) ;
#14861=CARTESIAN_POINT ( 'NONE',  ( -2.934900197419999746, -94.89197151660000884, 23.49669041109999768 ) ) ;
#14864=CARTESIAN_POINT ( 'NONE',  ( 12.83479102393274296, -101.4241070620153806, -9.841145288938006885 ) ) ;
#14877=CARTESIAN_POINT ( 'NONE',  ( 0.1178905558060000108, -101.2358105800000061, -15.21680457949999976 ) ) ;
#14883=EDGE_CURVE ( 'NONE', #4936, #7139, #3196, .T. ) ;
#14884=CARTESIAN_POINT ( 'NONE',  ( 6.820352230450000164, -100.2522625769999962, 15.59059167250000044 ) ) ;
#14885=CARTESIAN_POINT ( 'NONE',  ( -15.60709619170274998, -92.58000264305866267, -24.03322618717208314 ) ) ;
#14888=CARTESIAN_POINT ( 'NONE',  ( 5.634073923585436461, -92.54893169919640172, -29.97511075432250749 ) ) ;
#14892=CARTESIAN_POINT ( 'NONE',  ( 6.395435569720000046, -92.99570653130000153, -26.06839265949999884 ) ) ;
#14895=DIRECTION ( 'NONE',  ( 0.000000000000000000, 1.000000000000000000, 0.000000000000000000 ) ) ;
#14896=CARTESIAN_POINT ( 'NONE',  ( -6.659687227720000102, -101.1292389600000092, 14.00371911340000075 ) ) ;
#14901=CARTESIAN_POINT ( 'NONE',  ( -1.164566756239999945, -101.0314399550000104, -15.81222527010000078 ) ) ;
#14903=CARTESIAN_POINT ( 'NONE',  ( -13.14595447578818010, -93.06132686323303460, -23.62747619079523531 ) ) ;
#14905=CARTESIAN_POINT ( 'NONE',  ( 16.39013412538344383, -94.61155572397261437, 17.21914651918165973 ) ) ;
#14909=DIRECTION ( 'NONE',  ( -0.8791797166759636184, 0.000000000000000000, -0.4764903207679798691 ) ) ;
#14910=DIRECTION ( 'NONE',  ( 0.000000000000000000, 1.000000000000000000, 0.000000000000000000 ) ) ;
#14913=ADVANCED_FACE ( 'NONE', ( #25200 ), #17668, .F. ) ;
#14915=AXIS2_PLACEMENT_3D ( 'NONE', #27608, #3269, #7647 ) ;
#14917=EDGE_LOOP ( 'NONE', ( #26352, #15095, #10649, #25047 ) ) ;
#14924=CARTESIAN_POINT ( 'NONE',  ( -28.98513075869999867, -93.04780269100000112, 3.123877206889999592 ) ) ;
#14927=ORIENTED_EDGE ( 'NONE', *, *, #20939, .F. ) ;
#14935=CARTESIAN_POINT ( 'NONE',  ( -15.58072764279999944, -101.4054056550000098, 3.556023071709999872 ) ) ;
#14940=CARTESIAN_POINT ( 'NONE',  ( -12.57055767900000021, -101.5369810359999860, -9.898859202520000622 ) ) ;
#14941=CARTESIAN_POINT ( 'NONE',  ( 18.00137301776900856, -94.36683344921111427, 16.74636862984975139 ) ) ;
#14943=ORIENTED_EDGE ( 'NONE', *, *, #17606, .F. ) ;
#14950=EDGE_CURVE ( 'NONE', #16297, #6421, #9758, .T. ) ;
#14952=CARTESIAN_POINT ( 'NONE',  ( 7.033065480937148450, -100.0863963177764617, 15.73315454065260255 ) ) ;
#14957=CARTESIAN_POINT ( 'NONE',  ( 29.11677851939999684, -92.50000942380000879, 6.880019978119999990 ) ) ;
#14961=CARTESIAN_POINT ( 'NONE',  ( 12.08982211680000063, -101.2010924020000004, -9.314613846919998608 ) ) ;
#14963=EDGE_CURVE ( 'NONE', #23549, #14989, #11596, .T. ) ;
#14969=CARTESIAN_POINT ( 'NONE',  ( -20.51958746069999862, -95.60035679230000483, -9.357022945640000700 ) ) ;
#14970=CARTESIAN_POINT ( 'NONE',  ( 12.52961185140000033, -101.3852859389999992, -9.939768331349998931 ) ) ;
#14971=CARTESIAN_POINT ( 'NONE',  ( -2.876553231629999985, -108.5000000000000000, -5.265495371340000119 ) ) ;
#14972=CARTESIAN_POINT ( 'NONE',  ( 23.41224063439999981, -93.87552273890000265, -8.246875224729999232 ) ) ;
#14974=CARTESIAN_POINT ( 'NONE',  ( 29.84440213756046845, -92.58347372263781949, 6.289810756387969271 ) ) ;
#14975=LINE ( 'NONE', #28389, #27573 ) ;
#14977=DIRECTION ( 'NONE',  ( -0.2796552172570731520, 0.000000000000000000, -0.9601004944592516077 ) ) ;
#14978=EDGE_CURVE ( 'NONE', #22416, #24004, #3784, .T. ) ;
#14979=DIRECTION ( 'NONE',  ( 0.4794255386042040601, 0.000000000000000000, 0.8775825618903722036 ) ) ;
#14980=CARTESIAN_POINT ( 'NONE',  ( 18.29259584288750773, -98.99956642725410916, 3.353674926929683497 ) ) ;
#14983=CARTESIAN_POINT ( 'NONE',  ( 0.000000000000000000, -102.8486084350000027, 0.000000000000000000 ) ) ;
#14984=AXIS2_PLACEMENT_3D ( 'NONE', #27755, #7794, #16665 ) ;
#14985=AXIS2_PLACEMENT_3D ( 'NONE', #325, #19664, #13099 ) ;
#14986=ORIENTED_EDGE ( 'NONE', *, *, #15467, .T. ) ;
#14989=VERTEX_POINT ( 'NONE', #8502 ) ;
#14993=CARTESIAN_POINT ( 'NONE',  ( -12.41793182790000039, -101.2530993039999885, -8.757551688899999576 ) ) ;
#14994=CARTESIAN_POINT ( 'NONE',  ( 3.940393887960000008, -92.70565333729999224, 28.26336050760000163 ) ) ;
#14997=CARTESIAN_POINT ( 'NONE',  ( -29.72951945062797918, -92.77521214513809866, 6.812272564689533461 ) ) ;
#15000=CARTESIAN_POINT ( 'NONE',  ( 13.23050100943412133, -101.0147714270161288, -9.847845762695030203 ) ) ;
#15009=CARTESIAN_POINT ( 'NONE',  ( -17.68470881210000201, -94.03347263330000771, 17.09197474180000142 ) ) ;
#15010=CARTESIAN_POINT ( 'NONE',  ( -20.63373432448497269, -93.20343033882606676, 16.19767797687812916 ) ) ;
#15013=CARTESIAN_POINT ( 'NONE',  ( -0.07581514835600000612, -101.1292389600000092, -15.50644495179999893 ) ) ;
#15019=CARTESIAN_POINT ( 'NONE',  ( 6.592724576960000249, -99.70407914540000149, 15.88227091829999971 ) ) ;
#15020=CARTESIAN_POINT ( 'NONE',  ( 15.63748056140000209, -101.5369810359999860, 3.386620984279999913 ) ) ;
#15023=CARTESIAN_POINT ( 'NONE',  ( 4.907579521315320825, -92.69183043809221090, -30.10272373264253787 ) ) ;
#15028=CARTESIAN_POINT ( 'NONE',  ( 4.747154956369999290, -93.07693985719998864, -28.00930810119999848 ) ) ;
#15030=CARTESIAN_POINT ( 'NONE',  ( -1.303833584549999980, -101.1364147039999892, -15.29041300709999796 ) ) ;
#15031=CARTESIAN_POINT ( 'NONE',  ( -6.833925942180000490, -101.4254868729999970, 14.43295880549999843 ) ) ;
#15032=ORIENTED_EDGE ( 'NONE', *, *, #941, .F. ) ;
#15034=CARTESIAN_POINT ( 'NONE',  ( -12.46005120850608705, -101.3038909013870921, -10.45748730976263374 ) ) ;
#15038=ORIENTED_EDGE ( 'NONE', *, *, #81, .T. ) ;
#15040=CARTESIAN_POINT ( 'NONE',  ( -0.7205257403800000571, -101.6484611540000031, -15.98376809950000066 ) ) ;
#15043=CARTESIAN_POINT ( 'NONE',  ( 14.62247892739999955, -90.50000000000000000, 26.76626813769999913 ) ) ;
#15045=CARTESIAN_POINT ( 'NONE',  ( 12.88056670439999962, -94.79581646409999962, -19.86310537439999990 ) ) ;
#15047=EDGE_CURVE ( 'NONE', #20359, #22101, #1862, .T. ) ;
#15053=AXIS2_PLACEMENT_3D ( 'NONE', #18239, #27134, #4973 ) ;
#15060=VECTOR ( 'NONE', #4753, 1000.000000000000114 ) ;
#15062=CARTESIAN_POINT ( 'NONE',  ( -27.19238942870000031, -93.48569568790000517, -0.5495358801190000086 ) ) ;
#15065=CARTESIAN_POINT ( 'NONE',  ( -18.23664321284092082, -97.24405583968645317, -10.03008010378985482 ) ) ;
#15066=DIRECTION ( 'NONE',  ( -0.09713222731193690840, 0.000000000000000000, -0.9952714857853720565 ) ) ;
#15071=ADVANCED_FACE ( 'NONE', ( #26297 ), #18975, .T. ) ;
#15078=CARTESIAN_POINT ( 'NONE',  ( 11.44042105559999989, -101.2530993000000024, -9.998588429619998053 ) ) ;
#15082=CARTESIAN_POINT ( 'NONE',  ( -11.93759739729999936, -100.7707614970000094, -10.43389714689999970 ) ) ;
#15084=CARTESIAN_POINT ( 'NONE',  ( -15.55828293390000105, -111.0000000000000000, 3.733608462140000306 ) ) ;
#15086=FACE_BOUND ( 'NONE', #16765, .T. ) ;
#15088=VERTEX_POINT ( 'NONE', #13600 ) ;
#15090=CARTESIAN_POINT ( 'NONE',  ( 6.663412416092679535, -100.9364580247760301, 15.15463700478743014 ) ) ;
#15092=EDGE_LOOP ( 'NONE', ( #26621, #27335, #17658, #667 ) ) ;
#15094=CARTESIAN_POINT ( 'NONE',  ( -20.15691507911455105, -95.46331366771129012, 10.39344740093203612 ) ) ;
#15095=ORIENTED_EDGE ( 'NONE', *, *, #23777, .T. ) ;
#15102=CARTESIAN_POINT ( 'NONE',  ( -29.79635530287253786, -92.50000267096076811, -0.5908530661228191816 ) ) ;
#15103=CARTESIAN_POINT ( 'NONE',  ( -20.35840514350000063, -92.54807930229999613, -20.35479784810000226 ) ) ;
#15106=CARTESIAN_POINT ( 'NONE',  ( -22.25450292370000227, -94.89196973819998959, -8.089822570579999095 ) ) ;
#15107=CARTESIAN_POINT ( 'NONE',  ( 12.12202371060000061, -101.1402801299999936, -9.401285809570000040 ) ) ;
#15110=CARTESIAN_POINT ( 'NONE',  ( 29.78875618293655592, -92.66191076884391009, 6.548591290742901805 ) ) ;
#15112=VERTEX_POINT ( 'NONE', #20610 ) ;
#15114=FACE_OUTER_BOUND ( 'NONE', #20169, .T. ) ;
#15115=CARTESIAN_POINT ( 'NONE',  ( -23.78934072751362550, -92.89593097426853774, -19.08709831229086618 ) ) ;
#15117=CARTESIAN_POINT ( 'NONE',  ( -0.3895212963913376458, -92.61393927543522864, -30.49754768368999081 ) ) ;
#15122=CARTESIAN_POINT ( 'NONE',  ( -11.64049821129999884, -94.65528426899999204, -20.66308976129999664 ) ) ;
#15125=CARTESIAN_POINT ( 'NONE',  ( 20.85398878019999813, -96.96081042859999854, -2.285143478920000248 ) ) ;
#15126=ORIENTED_EDGE ( 'NONE', *, *, #6296, .F. ) ;
#15128=B_SPLINE_CURVE_WITH_KNOTS ( 'NONE', 3,
 ( #4906, #22241, #13786, #2733, #11587, #20495, #567, #27208, #16112, #9411, #10984 ),
 .UNSPECIFIED., .F., .F.,
 ( 4, 2, 1, 2, 2, 4 ),
 ( 0.000000000000000000, 0.2500000000000506262, 0.3750000000000652256, 0.4375000000000724976, 0.5000000000000797140, 1.000000000000000000 ),
 .UNSPECIFIED. ) ;
#15131=CARTESIAN_POINT ( 'NONE',  ( 13.56355163350000126, -96.34709473579999894, 17.13339730549999729 ) ) ;
#15132=ADVANCED_FACE ( 'NONE', ( #9372 ), #9407, .T. ) ;
#15144=CARTESIAN_POINT ( 'NONE',  ( 9.397459034720000659, -94.89420189139998740, -22.59846365579999983 ) ) ;
#15148=CARTESIAN_POINT ( 'NONE',  ( -15.61541000649999944, -92.60278524039999581, 23.76968555679999895 ) ) ;
#15150=EDGE_LOOP ( 'NONE', ( #20816, #21433, #13119, #18684 ) ) ;
#15152=CARTESIAN_POINT ( 'NONE',  ( 0.2341557092330000256, -101.3878691800000098, -16.10116432410000087 ) ) ;
#15154=CARTESIAN_POINT ( 'NONE',  ( 15.70072831049999706, -101.2995922080000071, 2.645407579260000031 ) ) ;
#15159=CARTESIAN_POINT ( 'NONE',  ( 6.693343950099999162, -101.2251655520000071, 14.77790851379999992 ) ) ;
#15160=CARTESIAN_POINT ( 'NONE',  ( 14.84965784370000108, -101.2530993010000060, 3.216001622850000352 ) ) ;
#15167=CARTESIAN_POINT ( 'NONE',  ( 3.402843465410000157, -92.87863185420000889, -28.93406916660000050 ) ) ;
#15169=CARTESIAN_POINT ( 'NONE',  ( 6.718680988475624005, -101.3846248971873223, 14.74555885599285432 ) ) ;
#15170=CARTESIAN_POINT ( 'NONE',  ( 0.000000000000000000, -107.1975888269999899, 0.000000000000000000 ) ) ;
#15172=CARTESIAN_POINT ( 'NONE',  ( -5.890277023240000354, -101.2306315440000049, 15.10563561669999899 ) ) ;
#15174=CARTESIAN_POINT ( 'NONE',  ( 12.77500156440000012, -92.50000000000000000, 27.05403395929999988 ) ) ;
#15184=CYLINDRICAL_SURFACE ( 'NONE', #19142, 0.7999999999999998224 ) ;
#15187=VERTEX_POINT ( 'NONE', #9944 ) ;
#15188=CARTESIAN_POINT ( 'NONE',  ( 0.1200718050890000055, -93.00000000000000000, -30.49976365090000030 ) ) ;
#15196=CARTESIAN_POINT ( 'NONE',  ( -27.18449005399999763, -93.39359504729999628, -0.5638341530459999307 ) ) ;
#15198=EDGE_CURVE ( 'NONE', #23834, #15494, #15797, .T. ) ;
#15201=CARTESIAN_POINT ( 'NONE',  ( 15.74738730109999807, -100.5717442099999914, 4.327233316820001008 ) ) ;
#15203=B_SPLINE_CURVE_WITH_KNOTS ( 'NONE', 5,
 ( #5467, #5609, #9832, #840, #25718, #12012 ),
 .UNSPECIFIED., .F., .F.,
 ( 6, 6 ),
 ( 0.000000000000000000, 1.000000000000000000 ),
 .UNSPECIFIED. ) ;
#15205=AXIS2_PLACEMENT_3D ( 'NONE', #25936, #21422, #16911 ) ;
#15207=ORIENTED_EDGE ( 'NONE', *, *, #19214, .F. ) ;
#15214=CARTESIAN_POINT ( 'NONE',  ( -13.36314309979999848, -101.1461874320000049, -9.085681040479999027 ) ) ;
#15216=CARTESIAN_POINT ( 'NONE',  ( -15.42268960139999834, -101.6484611540000031, 4.259183661159999801 ) ) ;
#15217=CARTESIAN_POINT ( 'NONE',  ( -12.51189201029999865, -101.4121386959999995, -9.936042548820001485 ) ) ;
#15219=CARTESIAN_POINT ( 'NONE',  ( -7.503851937626710544, -101.2111896144690348, 14.51426051703312048 ) ) ;
#15221=CARTESIAN_POINT ( 'NONE',  ( -0.9041074512197031510, -101.6174239712916574, -15.99763876592702161 ) ) ;
#15225=ORIENTED_EDGE ( 'NONE', *, *, #19369, .F. ) ;
#15226=ADVANCED_FACE ( 'NONE', ( #14043 ), #967, .F. ) ;
#15232=DIRECTION ( 'NONE',  ( 1.000000000000000000, 0.000000000000000000, 0.000000000000000000 ) ) ;
#15235=CARTESIAN_POINT ( 'NONE',  ( 24.18669557090000310, -93.21603318719999720, 12.26615263310000081 ) ) ;
#15240=DIRECTION ( 'NONE',  ( 0.000000000000000000, -1.000000000000000000, 0.000000000000000000 ) ) ;
#15246=CARTESIAN_POINT ( 'NONE',  ( 12.77836120849999801, -101.4829589650000088, -9.840357337720000430 ) ) ;
#15248=LINE ( 'NONE', #15400, #23974 ) ;
#15250=CARTESIAN_POINT ( 'NONE',  ( 29.91848600129237923, -92.52249206700025752, 5.927436511634884830 ) ) ;
#15258=CARTESIAN_POINT ( 'NONE',  ( -0.07760674669443720641, -92.74292563041224469, -30.49990831637531841 ) ) ;
#15267=CARTESIAN_POINT ( 'NONE',  ( 17.52693722629999939, -99.56347590660000435, 0.9950084100439999801 ) ) ;
#15272=DIRECTION ( 'NONE',  ( 1.000000000000000000, 0.000000000000000000, 0.000000000000000000 ) ) ;
#15277=CARTESIAN_POINT ( 'NONE',  ( -20.34966500099999820, -94.63958447440001009, 12.21934330610000075 ) ) ;
#15278=CARTESIAN_POINT ( 'NONE',  ( -29.61792381641411609, -92.58347372262699082, 7.282077114717079525 ) ) ;
#15279=CARTESIAN_POINT ( 'NONE',  ( 11.86655840719999944, -101.3150700380000018, -11.10431293650000129 ) ) ;
#15281=CARTESIAN_POINT ( 'NONE',  ( 8.799313986089998707, -92.58502644590001296, -27.24229809290000048 ) ) ;
#15287=CARTESIAN_POINT ( 'NONE',  ( -13.24502126470000007, -92.50000050830000475, 26.90831906640000071 ) ) ;
#15292=CARTESIAN_POINT ( 'NONE',  ( 0.7146172134730000014, -100.5717442099999914, -16.31546742289999941 ) ) ;
#15299=AXIS2_PLACEMENT_3D ( 'NONE', #20821, #7715, #14397 ) ;
#15301=CARTESIAN_POINT ( 'NONE',  ( 6.946330496749999917, -99.58396362730000817, 15.91260158950000303 ) ) ;
#15302=CARTESIAN_POINT ( 'NONE',  ( 15.61840456410000044, -101.6484611540000031, 3.474703039729999610 ) ) ;
#15303=CARTESIAN_POINT ( 'NONE',  ( -4.740443671060163844, -96.36359510251583060, 21.42699769422113576 ) ) ;
#15307=CARTESIAN_POINT ( 'NONE',  ( -17.38751286079999758, -93.83676151480000271, 17.80995846940000149 ) ) ;
#15309=CARTESIAN_POINT ( 'NONE',  ( 16.08037959500000014, -111.0000000000000000, 2.354223078750000031 ) ) ;
#15310=CARTESIAN_POINT ( 'NONE',  ( 9.370934950629999705, -94.71481161159999829, -22.48431492339999949 ) ) ;
#15316=DIRECTION ( 'NONE',  ( 0.000000000000000000, 1.000000000000000000, 0.000000000000000000 ) ) ;
#15319=CARTESIAN_POINT ( 'NONE',  ( 26.62516505820000035, -92.99999854809999533, -10.15609451739999969 ) ) ;
#15322=CARTESIAN_POINT ( 'NONE',  ( -1.025805314019999859, -101.2459394079999981, -15.92129411310000009 ) ) ;
#15323=EDGE_CURVE ( 'NONE', #5628, #22108, #20833, .T. ) ;
#15326=CARTESIAN_POINT ( 'NONE',  ( -20.26146926273735005, -92.62800705144270808, -22.79754751928403067 ) ) ;
#15328=CARTESIAN_POINT ( 'NONE',  ( -15.16614058569999912, -101.1716787529999948, 4.188334258429999402 ) ) ;
#15332=CARTESIAN_POINT ( 'NONE',  ( 11.86655840719999944, -101.3150700380000018, -11.10431293650000129 ) ) ;
#15336=CARTESIAN_POINT ( 'NONE',  ( 26.70978129881138230, -93.15741110562996141, 10.33020051488120750 ) ) ;
#15342=ORIENTED_EDGE ( 'NONE', *, *, #1713, .T. ) ;
#15345=CARTESIAN_POINT ( 'NONE',  ( -25.36533297769999962, -93.60790942680000626, -2.267491459940000009 ) ) ;
#15348=CARTESIAN_POINT ( 'NONE',  ( 16.30510774900000115, -100.5229262450000078, 4.375467603060000599 ) ) ;
#15365=ORIENTED_EDGE ( 'NONE', *, *, #976, .F. ) ;
#15367=CARTESIAN_POINT ( 'NONE',  ( -11.90690755189999983, -100.8685038539999965, -10.28167538419999971 ) ) ;
#15377=FACE_OUTER_BOUND ( 'NONE', #6495, .T. ) ;
#15378=AXIS2_PLACEMENT_3D ( 'NONE', #17803, #11662, #11217 ) ;
#15379=DIRECTION ( 'NONE',  ( 0.4794255386042041156, 0.000000000000000000, 0.8775825618903722036 ) ) ;
#15383=CARTESIAN_POINT ( 'NONE',  ( -19.23676770128301072, -97.09204376972030559, 7.281157557458501906 ) ) ;
#15385=CARTESIAN_POINT ( 'NONE',  ( 19.58568502800000033, -94.54719310899999130, 13.61987657130000073 ) ) ;
#15390=EDGE_LOOP ( 'NONE', ( #13495, #23648, #17785, #19918, #292, #19491 ) ) ;
#15392=CARTESIAN_POINT ( 'NONE',  ( 12.52134826220000186, -101.6311724339999927, -9.982697054739999132 ) ) ;
#15394=CARTESIAN_POINT ( 'NONE',  ( -16.52453304470000006, -93.48569568799999274, -21.60249615600000084 ) ) ;
#15397=CARTESIAN_POINT ( 'NONE',  ( -1.229530056899999835, -101.0685849509999912, -16.04536266459999894 ) ) ;
#15398=CARTESIAN_POINT ( 'NONE',  ( 12.91798634669999934, -101.2251655520000071, -9.813921847190000491 ) ) ;
#15400=CARTESIAN_POINT ( 'NONE',  ( 7.181689689069999716, -101.1889999979999999, 15.80535034289999885 ) ) ;
#15410=DIRECTION ( 'NONE',  ( 1.000000000000000000, 0.000000000000000000, 0.000000000000000000 ) ) ;
#15412=CARTESIAN_POINT ( 'NONE',  ( -24.38380614478478847, -92.52249206704190954, -18.32158033856656942 ) ) ;
#15415=B_SPLINE_SURFACE_WITH_KNOTS ( 'NONE', 5, 5, ( 
 ( #511, #8909, #9357, #15616, #4702, #10935 ),
 ( #22336, #9061, #24819, #17675, #4858, #2382 ),
 ( #6602, #13737, #24669, #11239, #24372, #20146 ),
 ( #11073, #22637, #2676, #26415, #22189, #13583 ),
 ( #2230, #62, #17820, #215, #17965, #6898 ),
 ( #15763, #22936, #11833, #4991, #20594, #5145 ) ),
 .UNSPECIFIED., .F., .F., .F.,
 ( 6, 6 ),
 ( 6, 6 ),
 ( 7.179431123180000540, 23.44689954740000104 ),
 ( 0.000000000000000000, 0.5000000000000000000 ),
 .UNSPECIFIED. ) ;
#15417=DIRECTION ( 'NONE',  ( 0.000000000000000000, -1.000000000000000000, 0.000000000000000000 ) ) ;
#15419=ADVANCED_BREP_SHAPE_REPRESENTATION ( '', ( #25670, #26433 ), #17143 ) ;
#15420=DIRECTION ( 'NONE',  ( 0.000000000000000000, -1.000000000000000000, 0.000000000000000000 ) ) ;
#15421=CARTESIAN_POINT ( 'NONE',  ( 15.98190521330000102, -101.1461869959999973, 2.387867047529999898 ) ) ;
#15425=EDGE_LOOP ( 'NONE', ( #5217, #5611, #9464, #15365, #14006, #24694 ) ) ;
#15426=AXIS2_PLACEMENT_3D ( 'NONE', #1342, #27587, #16769 ) ;
#15427=CARTESIAN_POINT ( 'NONE',  ( 15.64667777420000050, -100.8816835080000089, 2.154424203329999621 ) ) ;
#15428=ORIENTED_EDGE ( 'NONE', *, *, #18963, .F. ) ;
#15429=CARTESIAN_POINT ( 'NONE',  ( -8.825292394359999903, -96.19637846910001144, -20.90069174230000115 ) ) ;
#15432=CARTESIAN_POINT ( 'NONE',  ( -16.97615606580000147, -99.73367829289999520, 3.380302814300000236 ) ) ;
#15437=CARTESIAN_POINT ( 'NONE',  ( 10.37782365410000018, -92.68419354089999729, -25.56315968380000214 ) ) ;
#15443=CARTESIAN_POINT ( 'NONE',  ( -15.13518098839999837, -92.64783192670000744, 25.02785625110000112 ) ) ;
#15445=ORIENTED_EDGE ( 'NONE', *, *, #25096, .F. ) ;
#15449=CARTESIAN_POINT ( 'NONE',  ( 0.4780712722559999905, -101.0403179300000005, -15.46279129750000081 ) ) ;
#15457=CARTESIAN_POINT ( 'NONE',  ( -13.18661234450000030, -92.50000000000000000, 26.85581265420000108 ) ) ;
#15458=DIRECTION ( 'NONE',  ( 0.000000000000000000, -1.000000000000000000, 0.000000000000000000 ) ) ;
#15459=CARTESIAN_POINT ( 'NONE',  ( -4.643934244949999623, -95.55433883409999396, 22.13027033890000084 ) ) ;
#15461=FACE_OUTER_BOUND ( 'NONE', #23512, .T. ) ;
#15467=EDGE_CURVE ( 'NONE', #24004, #19902, #13161, .T. ) ;
#15473=CARTESIAN_POINT ( 'NONE',  ( 9.385332722619999402, -98.68450614990000247, 16.47661810339999988 ) ) ;
#15476=CARTESIAN_POINT ( 'NONE',  ( -19.63244573686088046, -92.50638022835023833, -23.34176391067345691 ) ) ;
#15478=CARTESIAN_POINT ( 'NONE',  ( -15.38823321699999980, -101.6484610359999863, 4.383952149800000697 ) ) ;
#15485=CARTESIAN_POINT ( 'NONE',  ( 13.80626276613105929, -99.96200787833144830, -10.48157719901313456 ) ) ;
#15489=CARTESIAN_POINT ( 'NONE',  ( 22.52953341510427521, -94.00303307112771734, 13.14769211859860576 ) ) ;
#15491=FACE_OUTER_BOUND ( 'NONE', #24433, .T. ) ;
#15492=CARTESIAN_POINT ( 'NONE',  ( 7.932078966940000697, -101.4167270020000018, 13.98634163589999879 ) ) ;
#15494=VERTEX_POINT ( 'NONE', #19600 ) ;
#15498=CARTESIAN_POINT ( 'NONE',  ( 6.114061450890000415, -93.00000000000000000, -13.40104985119999981 ) ) ;
#15500=DIRECTION ( 'NONE',  ( 0.000000000000000000, -1.000000000000000000, 0.000000000000000000 ) ) ;
#15501=CARTESIAN_POINT ( 'NONE',  ( 9.385332722619999402, -98.68450614990000247, 16.47661810339999988 ) ) ;
#15505=CARTESIAN_POINT ( 'NONE',  ( -13.36314236379999976, -101.1461869959999973, -9.085682662689999134 ) ) ;
#15506=EDGE_LOOP ( 'NONE', ( #24288, #26070, #14315, #20382, #13092, #27388, #13599 ) ) ;
#15507=CARTESIAN_POINT ( 'NONE',  ( 7.929587929925636658, -92.54893169919635909, 29.45117466200463952 ) ) ;
#15513=CARTESIAN_POINT ( 'NONE',  ( 24.47773556059999933, -92.99999932709999939, -17.01937738950000067 ) ) ;
#15516=CARTESIAN_POINT ( 'NONE',  ( -16.09756696615421134, -99.27923575797652234, 7.463221687748802680 ) ) ;
#15520=CARTESIAN_POINT ( 'NONE',  ( -12.37368733949999999, -100.1512121650000040, -11.12496841619999977 ) ) ;
#15523=ORIENTED_EDGE ( 'NONE', *, *, #8956, .F. ) ;
#15524=AXIS2_PLACEMENT_3D ( 'NONE', #26005, #14910, #23677 ) ;
#15527=ORIENTED_EDGE ( 'NONE', *, *, #19523, .T. ) ;
#15530=CARTESIAN_POINT ( 'NONE',  ( -6.665307709260000379, -101.1889999979999999, -13.13558364449999871 ) ) ;
#15533=MECHANICAL_DESIGN_GEOMETRIC_PRESENTATION_REPRESENTATION('',(#20699),#9977);
#15534=CARTESIAN_POINT ( 'NONE',  ( 12.80177023699999950, -92.76842269019999776, 27.50696703210000038 ) ) ;
#15536=CARTESIAN_POINT ( 'NONE',  ( 0.000000000000000000, -92.50000000000000000, 0.000000000000000000 ) ) ;
#15537=CARTESIAN_POINT ( 'NONE',  ( -19.96511697432906374, -95.86227943297046750, 9.608863210890680406 ) ) ;
#15540=CARTESIAN_POINT ( 'NONE',  ( -25.25510951461192732, -94.35876167706931028, -2.968759144345000323 ) ) ;
#15541=CARTESIAN_POINT ( 'NONE',  ( 21.82349187340000185, -93.59856831130001353, 12.95706236810000078 ) ) ;
#15545=CARTESIAN_POINT ( 'NONE',  ( 16.44117558850142302, -94.63960343439929090, 17.12038290499986459 ) ) ;
#15549=CARTESIAN_POINT ( 'NONE',  ( -14.18321254710000012, -94.09272382180000704, -21.64669162210000053 ) ) ;
#15553=CARTESIAN_POINT ( 'NONE',  ( 14.01704999690000086, -99.70407914540000149, -9.961568965490000593 ) ) ;
#15556=DIRECTION ( 'NONE',  ( 1.000000000000000000, 0.000000000000000000, 0.000000000000000000 ) ) ;
#15561=CIRCLE ( 'NONE', #13732, 30.50000000000000000 ) ;
#15575=CARTESIAN_POINT ( 'NONE',  ( 16.58537890990000108, -94.98812477769999418, 16.93952572510000110 ) ) ;
#15576=CARTESIAN_POINT ( 'NONE',  ( 16.03761577559999907, -101.2306310700000012, 2.381277126570000569 ) ) ;
#15581=VERTEX_POINT ( 'NONE', #18881 ) ;
#15582=CARTESIAN_POINT ( 'NONE',  ( 15.58784579500000156, -100.8733988930000010, 2.070706579690000382 ) ) ;
#15583=EDGE_CURVE ( 'NONE', #6867, #25460, #15203, .T. ) ;
#15585=CARTESIAN_POINT ( 'NONE',  ( -11.21687034500000024, -94.79905218150000223, -20.68493743190000345 ) ) ;
#15593=DIRECTION ( 'NONE',  ( 0.000000000000000000, -1.000000000000000000, 0.000000000000000000 ) ) ;
#15596=CARTESIAN_POINT ( 'NONE',  ( -12.82502785340713025, -92.59735406121865253, 27.67253584333921879 ) ) ;
#15599=CARTESIAN_POINT ( 'NONE',  ( -14.04679603149999956, -92.49999866209999766, 25.86342652180000101 ) ) ;
#15600=DIRECTION ( 'NONE',  ( 0.4794255386042040601, 0.000000000000000000, 0.8775825618903719816 ) ) ;
#15601=ORIENTED_EDGE ( 'NONE', *, *, #11336, .T. ) ;
#15603=CARTESIAN_POINT ( 'NONE',  ( 0.4195603051590000021, -100.9364576079999978, -15.94533468339999871 ) ) ;
#15610=CARTESIAN_POINT ( 'NONE',  ( 28.44652200260433972, -92.82529299094275643, 11.00206337811066959 ) ) ;
#15611=CARTESIAN_POINT ( 'NONE',  ( 8.630545616070000037, -99.09990215500000943, 16.29201985859999624 ) ) ;
#15616=CARTESIAN_POINT ( 'NONE',  ( 26.48196640509999966, -92.56168957700000988, 13.31191097970000037 ) ) ;
#15619=CARTESIAN_POINT ( 'NONE',  ( -7.515932239300000539, -100.7707614970000094, 13.96005744500000034 ) ) ;
#15624=ORIENTED_EDGE ( 'NONE', *, *, #27264, .F. ) ;
#15625=CARTESIAN_POINT ( 'NONE',  ( 7.609509498830000496, -99.68121713349998458, 15.96225029060000011 ) ) ;
#15628=CARTESIAN_POINT ( 'NONE',  ( -5.703789389510000696, -95.94970068800000718, -21.79542136019999887 ) ) ;
#15629=CARTESIAN_POINT ( 'NONE',  ( -19.92269764396411347, -92.54893169919635909, -23.09407223288071620 ) ) ;
#15631=CARTESIAN_POINT ( 'NONE',  ( -15.48258886210000185, -101.2306315829999903, 4.813006563600000121 ) ) ;
#15633=CARTESIAN_POINT ( 'NONE',  ( 15.04667461659597016, -95.25682781127063947, 17.31483459787338575 ) ) ;
#15634=DIRECTION ( 'NONE',  ( 0.000000000000000000, -1.000000000000000000, 0.000000000000000000 ) ) ;
#15635=DIRECTION ( 'NONE',  ( -0.2287893768880245038, 0.000000000000000000, 0.9734759478401042720 ) ) ;
#15637=CARTESIAN_POINT ( 'NONE',  ( 24.70277711335754844, -93.45279863401688658, -11.97073514444795173 ) ) ;
#15641=CARTESIAN_POINT ( 'NONE',  ( 8.185346603670000221, -101.3150705270000032, 14.03998133939999882 ) ) ;
#15642=EDGE_CURVE ( 'NONE', #26855, #25651, #10094, .T. ) ;
#15644=CARTESIAN_POINT ( 'NONE',  ( -0.7543003842240000312, -101.1889999979999999, -16.73300722909999649 ) ) ;
#15645=CARTESIAN_POINT ( 'NONE',  ( 30.00028607799999847, -92.50000000000000000, 5.498439345520000465 ) ) ;
#15646=B_SPLINE_CURVE_WITH_KNOTS ( 'NONE', 5,
 ( #13938, #20347, #5049, #416, #9266, #9412 ),
 .UNSPECIFIED., .F., .F.,
 ( 6, 6 ),
 ( 0.000000000000000000, 1.000000000000000000 ),
 .UNSPECIFIED. ) ;
#15647=CARTESIAN_POINT ( 'NONE',  ( -26.83792192550000166, -92.99570653130000153, -0.4343255661159999836 ) ) ;
#15649=EDGE_CURVE ( 'NONE', #12485, #19902, #11724, .T. ) ;
#15651=CARTESIAN_POINT ( 'NONE',  ( 16.51865411080000001, -99.74726900420000675, 4.630948717549999927 ) ) ;
#15659=LINE ( 'NONE', #11429, #21426 ) ;
#15661=DIRECTION ( 'NONE',  ( -0.000000000000000000, 1.000000000000000000, 0.000000000000000000 ) ) ;
#15662=CARTESIAN_POINT ( 'NONE',  ( 23.68384408339999680, -92.51542729400000553, -18.51872027609999805 ) ) ;
#15665=CARTESIAN_POINT ( 'NONE',  ( -16.23097981328315953, -99.08289723854821318, 7.775255002977575991 ) ) ;
#15668=CARTESIAN_POINT ( 'NONE',  ( 8.185346967789998374, -101.3150701389999995, 14.03998109830000018 ) ) ;
#15670=CARTESIAN_POINT ( 'NONE',  ( -12.08161827610000039, -100.4808658609999981, -10.82458641699999902 ) ) ;
#15674=CARTESIAN_POINT ( 'NONE',  ( 26.64643508839107255, -92.66777315148785021, -14.83972869400399652 ) ) ;
#15676=EDGE_CURVE ( 'NONE', #7443, #13918, #1679, .T. ) ;
#15677=CYLINDRICAL_SURFACE ( 'NONE', #16039, 20.64285714289998452 ) ;
#15681=CARTESIAN_POINT ( 'NONE',  ( 12.80359094900000017, -92.84292109160000450, 27.53777204920000088 ) ) ;
#15685=CARTESIAN_POINT ( 'NONE',  ( -27.01692611455537829, -93.59825775049449703, -0.6446940546961127394 ) ) ;
#15687=DIRECTION ( 'NONE',  ( 0.000000000000000000, -1.000000000000000000, 0.000000000000000000 ) ) ;
#15693=FACE_OUTER_BOUND ( 'NONE', #22294, .T. ) ;
#15696=ORIENTED_EDGE ( 'NONE', *, *, #12267, .T. ) ;
#15707=CARTESIAN_POINT ( 'NONE',  ( -11.98151724899999948, -93.50556391630000519, -23.51195765390000147 ) ) ;
#15708=B_SPLINE_CURVE_WITH_KNOTS ( 'NONE', 3,
 ( #16890, #19208, #12220, #21130, #1188, #5807, #17022, #18938, #27822, #25909, #25640, #5669, #14548, #14687, #23582, #5936, #4184, #28650, #24444, #16091, #15383, #28798, #6227, #1870, #21968, #4338, #6672, #10566, #4479, #2019, #28517, #10858, #20474, #15537, #1726, #19910, #545, #24993, #4039, #15094, #24152, #24294, #21678, #13059 ),
 .UNSPECIFIED., .F., .F.,
 ( 4, 2, 2, 1, 1, 1, 1, 2, 2, 2, 2, 1, 1, 1, 1, 1, 2, 2, 2, 2, 1, 1, 1, 1, 1, 2, 2, 2, 4 ),
 ( 0.000000000000000000, 0.1250000000000717204, 0.1875000000001076916, 0.2187500000001266487, 0.2343750000001371681, 0.2421875000001423583, 0.2460937500001457723, 0.2480468750001485201, 0.2500000000001512679, 0.3750000000003486100, 0.4375000000004475309, 0.4687500000004961587, 0.4843750000005205281, 0.4921875000005318523, 0.4960937500005382361, 0.4980468750005404011, 0.4990234375005415668, 0.5000000000005426770, 0.6250000000004817258, 0.6875000000004524159, 0.7187500000004385381, 0.7343750000004307665, 0.7421875000004278800, 0.7460937500004269918, 0.7480468750004258816, 0.7490234375004246603, 0.7500000000004234391, 0.8750000000002117195, 1.000000000000000000 ),
 .UNSPECIFIED. ) ;
#15710=CARTESIAN_POINT ( 'NONE',  ( -24.12489041853968885, -92.59735406125496127, -18.66119614963135120 ) ) ;
#15713=CARTESIAN_POINT ( 'NONE',  ( -14.60468409838225234, -101.1900861939869429, 4.477069939566454160 ) ) ;
#15716=LINE ( 'NONE', #26967, #23333 ) ;
#15718=CARTESIAN_POINT ( 'NONE',  ( 15.64667784240000081, -100.8816831189999874, 2.154425576790000019 ) ) ;
#15723=VERTEX_POINT ( 'NONE', #8489 ) ;
#15726=B_SPLINE_CURVE_WITH_KNOTS ( 'NONE', 3,
 ( #26662, #6704, #6849, #2332, #20099, #13689, #164, #15713, #13532, #15865, #19172, #13831 ),
 .UNSPECIFIED., .F., .F.,
 ( 4, 2, 2, 2, 2, 4 ),
 ( 0.000000000000000000, 0.2499999999999875100, 0.3749999999999895639, 0.4999999999999916733, 0.7499999999999957812, 1.000000000000000000 ),
 .UNSPECIFIED. ) ;
#15727=CARTESIAN_POINT ( 'NONE',  ( 5.725409811050989894, -93.38817447844444075, -27.06492380005755649 ) ) ;
#15729=DIRECTION ( 'NONE',  ( 1.000000000000000000, 0.000000000000000000, 0.000000000000000000 ) ) ;
#15732=ORIENTED_EDGE ( 'NONE', *, *, #21387, .F. ) ;
#15737=CARTESIAN_POINT ( 'NONE',  ( -12.41862539467342508, -92.52048598158050652, 27.85727924331794725 ) ) ;
#15738=ORIENTED_EDGE ( 'NONE', *, *, #12834, .F. ) ;
#15739=CARTESIAN_POINT ( 'NONE',  ( 13.12744653600000078, -94.59276292389999696, -19.84842857619999990 ) ) ;
#15741=CARTESIAN_POINT ( 'NONE',  ( 15.74335372269999844, -101.6484611540000031, 2.854262350110000401 ) ) ;
#15744=CARTESIAN_POINT ( 'NONE',  ( -14.86197364899999940, -100.8869795979999964, 4.957594172660000353 ) ) ;
#15745=CARTESIAN_POINT ( 'NONE',  ( -12.94585355975605445, -101.5555610555526869, -9.402386697501409429 ) ) ;
#15746=CARTESIAN_POINT ( 'NONE',  ( 0.6332782371249999764, -100.6809449770000100, -16.42402731589999831 ) ) ;
#15747=DIRECTION ( 'NONE',  ( 0.000000000000000000, -1.000000000000000000, 0.000000000000000000 ) ) ;
#15752=DIRECTION ( 'NONE',  ( 0.000000000000000000, 1.000000000000000000, 0.000000000000000000 ) ) ;
#15757=AXIS2_PLACEMENT_3D ( 'NONE', #28417, #8452, #19256 ) ;
#15760=CARTESIAN_POINT ( 'NONE',  ( 8.137532908689999900, -101.2306311739999956, 14.02341457380000023 ) ) ;
#15763=CARTESIAN_POINT ( 'NONE',  ( 16.58537991969999936, -94.98812656900000206, 16.93952948469999953 ) ) ;
#15770=DIRECTION ( 'NONE',  ( 0.000000000000000000, -1.000000000000000000, 0.000000000000000000 ) ) ;
#15772=CARTESIAN_POINT ( 'NONE',  ( -2.288843675430000335, -97.83383802270000729, -19.83674288659999974 ) ) ;
#15774=CARTESIAN_POINT ( 'NONE',  ( 0.000000000000000000, -101.1889999979999999, 0.000000000000000000 ) ) ;
#15775=EDGE_LOOP ( 'NONE', ( #25010, #19118, #9970, #3458 ) ) ;
#15776=CARTESIAN_POINT ( 'NONE',  ( -15.15665000090000092, -101.0314213319999936, 4.653947536529999596 ) ) ;
#15778=VECTOR ( 'NONE', #26311, 1000.000000000000000 ) ;
#15782=DIRECTION ( 'NONE',  ( 1.000000000000000000, 0.000000000000000000, 0.000000000000000000 ) ) ;
#15785=CARTESIAN_POINT ( 'NONE',  ( 15.34608781240000042, -101.0356131030000029, 1.995616791270000023 ) ) ;
#15786=CARTESIAN_POINT ( 'NONE',  ( 25.92294088882810499, -93.25521311087592835, 11.00152434285968361 ) ) ;
#15790=CARTESIAN_POINT ( 'NONE',  ( 8.023929893669999203, -101.0253300669999987, 13.24802822849999906 ) ) ;
#15795=DIRECTION ( 'NONE',  ( 0.000000000000000000, 1.000000000000000000, 0.000000000000000000 ) ) ;
#15797=CIRCLE ( 'NONE', #20477, 29.91857981989999971 ) ;
#15800=CARTESIAN_POINT ( 'NONE',  ( 16.48292494720000079, -100.3063911739999980, 4.382887648540000569 ) ) ;
#15801=EDGE_LOOP ( 'NONE', ( #8263, #23458, #6370, #9870 ) ) ;
#15803=CARTESIAN_POINT ( 'NONE',  ( -22.29259858720000054, -96.16784750930000314, -5.870011727330000539 ) ) ;
#15807=DIRECTION ( 'NONE',  ( 0.000000000000000000, 1.000000000000000000, 0.000000000000000000 ) ) ;
#15809=ADVANCED_FACE ( 'NONE', ( #12708 ), #26397, .T. ) ;
#15811=CARTESIAN_POINT ( 'NONE',  ( 22.95300118209999951, -94.52293239719999463, -6.773262432920000187 ) ) ;
#15815=CARTESIAN_POINT ( 'NONE',  ( -16.61661837067523351, -98.46254901739948195, 8.790168390964289813 ) ) ;
#15818=CARTESIAN_POINT ( 'NONE',  ( -3.153926688883155194, -98.09459569084205555, 20.20253999486456564 ) ) ;
#15819=CARTESIAN_POINT ( 'NONE',  ( -12.73014500989999931, -100.0496341300000154, -11.13483849640000045 ) ) ;
#15821=CIRCLE ( 'NONE', #2828, 5.499999999999998224 ) ;
#15826=CARTESIAN_POINT ( 'NONE',  ( 26.26892325874138123, -92.86276748829368444, -15.49872433666240745 ) ) ;
#15831=CARTESIAN_POINT ( 'NONE',  ( 11.26686242699999951, -92.77082804750000378, 27.55452589829999965 ) ) ;
#15836=CARTESIAN_POINT ( 'NONE',  ( 23.88581173909999933, -92.98481359359999487, 11.87508144250000086 ) ) ;
#15838=EDGE_LOOP ( 'NONE', ( #13656, #25332, #15624, #8375 ) ) ;
#15840=DIRECTION ( 'NONE',  ( 0.000000000000000000, 1.000000000000000000, 0.000000000000000000 ) ) ;
#15843=AXIS2_PLACEMENT_3D ( 'NONE', #23573, #3614, #3481 ) ;
#15850=CARTESIAN_POINT ( 'NONE',  ( -16.89186647220000026, -100.0262800969999972, 3.317271451419999906 ) ) ;
#15857=ORIENTED_EDGE ( 'NONE', *, *, #27023, .F. ) ;
#15858=CARTESIAN_POINT ( 'NONE',  ( -9.636993756300000769, -93.95774545369999942, -23.10706980140000155 ) ) ;
#15861=CARTESIAN_POINT ( 'NONE',  ( 15.98533867912071216, -100.9616911410360984, 4.227991388196914890 ) ) ;
#15865=CARTESIAN_POINT ( 'NONE',  ( -14.60853884240962408, -101.2450099480301020, 4.215530974001670650 ) ) ;
#15867=AXIS2_PLACEMENT_3D ( 'NONE', #17944, #6728, #7021 ) ;
#15877=CARTESIAN_POINT ( 'NONE',  ( 9.165534020747788446, -98.33329995119029832, 16.60371393490449421 ) ) ;
#15878=ORIENTED_EDGE ( 'NONE', *, *, #21606, .F. ) ;
#15880=CARTESIAN_POINT ( 'NONE',  ( 4.340170735955752868, -93.18010901074717367, -28.18556222814888912 ) ) ;
#15881=CARTESIAN_POINT ( 'NONE',  ( 1.563021348000000144, -94.54719592040000009, 23.80457129850000086 ) ) ;
#15882=CARTESIAN_POINT ( 'NONE',  ( -19.56140538540000051, -96.65247697220000589, 8.334726878210000578 ) ) ;
#15883=CARTESIAN_POINT ( 'NONE',  ( 15.50925563669999896, -100.9197081840000010, 1.894558565230000102 ) ) ;
#15886=ORIENTED_EDGE ( 'NONE', *, *, #21882, .T. ) ;
#15887=CIRCLE ( 'NONE', #3349, 20.64285714290000229 ) ;
#15891=CARTESIAN_POINT ( 'NONE',  ( -13.26438106576386744, -92.82709422631874929, 27.46463547702218122 ) ) ;
#15894=DIRECTION ( 'NONE',  ( 0.000000000000000000, 1.000000000000000000, 0.000000000000000000 ) ) ;
#15895=DIRECTION ( 'NONE',  ( 0.4238361315509043825, 0.000000000000000000, -0.9057388881967940453 ) ) ;
#15897=CARTESIAN_POINT ( 'NONE',  ( -18.05296423140000073, -94.57749571930000343, 16.11415966959999935 ) ) ;
#15903=CARTESIAN_POINT ( 'NONE',  ( 7.130058149629999953, -99.83167681540000160, 15.79461927190000203 ) ) ;
#15905=EDGE_LOOP ( 'NONE', ( #4305, #22127, #1163, #26199, #27685 ) ) ;
#15907=CARTESIAN_POINT ( 'NONE',  ( 28.21054109043858915, -92.66455718075739867, 11.59376651551000315 ) ) ;
#15909=EDGE_CURVE ( 'NONE', #23006, #23088, #8915, .T. ) ;
#15910=CARTESIAN_POINT ( 'NONE',  ( 14.78896428320000034, -96.97547306780001009, 14.66850198189999865 ) ) ;
#15913=CARTESIAN_POINT ( 'NONE',  ( 6.258798239620000814, -92.50000000000000000, -29.85092033080000107 ) ) ;
#15920=CARTESIAN_POINT ( 'NONE',  ( 7.132709192110000096, -99.83167692499999646, 15.78738634319999967 ) ) ;
#15923=CARTESIAN_POINT ( 'NONE',  ( 0.4235579524470000634, -99.83167544280000527, -17.31869659160000197 ) ) ;
#15929=CARTESIAN_POINT ( 'NONE',  ( -24.15516222759999820, -94.98812477599999227, -4.102682929219999330 ) ) ;
#15930=DIRECTION ( 'NONE',  ( 1.000000000000000000, 0.000000000000000000, 0.000000000000000000 ) ) ;
#15941=CIRCLE ( 'NONE', #10799, 29.91857981989999971 ) ;
#15944=CIRCLE ( 'NONE', #3408, 10.00000000000000000 ) ;
#15946=B_SPLINE_CURVE_WITH_KNOTS ( 'NONE', 5,
 ( #9980, #18894, #25592, #23122, #20797, #2879 ),
 .UNSPECIFIED., .F., .F.,
 ( 6, 6 ),
 ( 0.000000000000000000, 1.000000000000000000 ),
 .UNSPECIFIED. ) ;
#15948=CARTESIAN_POINT ( 'NONE',  ( -13.34153245340000105, -91.50000000000000000, 27.42724032409999779 ) ) ;
#15952=CARTESIAN_POINT ( 'NONE',  ( -17.58990901810000196, -98.24904979049999554, -7.931573376680000287 ) ) ;
#15955=CARTESIAN_POINT ( 'NONE',  ( 9.264753623212678590, -92.86276748881633125, 29.05909712188475780 ) ) ;
#15957=DIRECTION ( 'NONE',  ( 0.000000000000000000, 1.000000000000000000, 0.000000000000000000 ) ) ;
#15958=CARTESIAN_POINT ( 'NONE',  ( -7.639087602144537748, -98.53908159008453538, 17.12000419490125580 ) ) ;
#15959=CIRCLE ( 'NONE', #2013, 30.50000000000000000 ) ;
#15963=CARTESIAN_POINT ( 'NONE',  ( -8.929965488379998817, -95.98352844290000974, -20.19091974539999867 ) ) ;
#15964=CARTESIAN_POINT ( 'NONE',  ( -17.02803783414526961, -97.66783633811731136, 10.15242468662800412 ) ) ;
#15968=CARTESIAN_POINT ( 'NONE',  ( -13.15237738589999950, -99.55609327400000552, -11.37038234410000115 ) ) ;
#15969=AXIS2_PLACEMENT_3D ( 'NONE', #24791, #13254, #15729 ) ;
#15975=LINE ( 'NONE', #22559, #13715 ) ;
#15977=FACE_OUTER_BOUND ( 'NONE', #18481, .T. ) ;
#15978=CARTESIAN_POINT ( 'NONE',  ( 2.731422428999999763, -93.80378326950000201, 24.76396224019999792 ) ) ;
#15979=ORIENTED_EDGE ( 'NONE', *, *, #5439, .T. ) ;
#15986=ORIENTED_EDGE ( 'NONE', *, *, #1470, .F. ) ;
#15994=DIRECTION ( 'NONE',  ( 0.000000000000000000, 1.000000000000000000, 0.000000000000000000 ) ) ;
#15997=CIRCLE ( 'NONE', #14609, 0.4999999999999987232 ) ;
#15998=CARTESIAN_POINT ( 'NONE',  ( 13.78129364559999814, -99.94751438429999268, -10.21817317360000210 ) ) ;
#16004=CARTESIAN_POINT ( 'NONE',  ( -0.1689899845689999958, -101.2530993010000060, -15.19297360289999865 ) ) ;
#16007=CARTESIAN_POINT ( 'NONE',  ( -13.09440877569999984, -92.84550106799999014, -23.96917193350000019 ) ) ;
#16010=CARTESIAN_POINT ( 'NONE',  ( 16.37130097589949784, -100.4507315479511078, 4.354834957207184054 ) ) ;
#16014=AXIS2_PLACEMENT_3D ( 'NONE', #6659, #20058, #24574 ) ;
#16018=DIRECTION ( 'NONE',  ( 1.000000000000000000, 0.000000000000000000, 0.000000000000000000 ) ) ;
#16019=CARTESIAN_POINT ( 'NONE',  ( 10.60935311512664647, -93.02766005061967292, 27.57871627749636545 ) ) ;
#16023=ORIENTED_EDGE ( 'NONE', *, *, #18844, .F. ) ;
#16027=CARTESIAN_POINT ( 'NONE',  ( -18.09292965979135914, -92.55388824293693517, -23.53605431443747520 ) ) ;
#16029=CARTESIAN_POINT ( 'NONE',  ( -29.91144828099999842, -92.50000000000000000, -0.6532076026720000650 ) ) ;
#16031=CARTESIAN_POINT ( 'NONE',  ( -19.97010144720000113, -95.85316701180001075, 10.36429926879999996 ) ) ;
#16035=CARTESIAN_POINT ( 'NONE',  ( 12.33671740429999986, -93.75379239689999622, -21.67807059210000276 ) ) ;
#16039=AXIS2_PLACEMENT_3D ( 'NONE', #15530, #24437, #24738 ) ;
#16042=FACE_OUTER_BOUND ( 'NONE', #8891, .T. ) ;
#16044=CARTESIAN_POINT ( 'NONE',  ( -17.52609522539999887, -98.43713976429998525, 8.802680806179999706 ) ) ;
#16047=CARTESIAN_POINT ( 'NONE',  ( 0.5239533329500000169, -99.69348480060000384, -17.31365208049999893 ) ) ;
#16053=VERTEX_POINT ( 'NONE', #23080 ) ;
#16059=CARTESIAN_POINT ( 'NONE',  ( 23.53235809685696367, -92.58608763741389680, -19.40304636274978378 ) ) ;
#16067=CARTESIAN_POINT ( 'NONE',  ( 8.316147692919997780, -98.89962500040000748, 16.28909968399999997 ) ) ;
#16069=CARTESIAN_POINT ( 'NONE',  ( -2.157875506039999891, -97.64874574800001028, -19.85504165189999881 ) ) ;
#16070=CARTESIAN_POINT ( 'NONE',  ( 26.75649127029999619, -93.00000000000000000, -13.26822602009999841 ) ) ;
#16072=CARTESIAN_POINT ( 'NONE',  ( -15.03193870770000018, -100.8816836399999914, 4.847770938290000053 ) ) ;
#16074=CARTESIAN_POINT ( 'NONE',  ( -18.94876721349164583, -98.12113811964421473, -7.590811461915794034 ) ) ;
#16076=EDGE_CURVE ( 'NONE', #12485, #22153, #20848, .T. ) ;
#16080=CARTESIAN_POINT ( 'NONE',  ( 24.72534431299499147, -93.40025063776721481, -12.31560360671905840 ) ) ;
#16081=CARTESIAN_POINT ( 'NONE',  ( -15.23837145989999797, -101.0223441809999940, 2.799506657709999846 ) ) ;
#16084=CARTESIAN_POINT ( 'NONE',  ( 6.783366714739999637, -101.1848541609999899, 13.69406429940000081 ) ) ;
#16085=CARTESIAN_POINT ( 'NONE',  ( 7.824897742070000106, -101.4837543189999991, 13.99581122470000061 ) ) ;
#16086=AXIS2_PLACEMENT_3D ( 'NONE', #7069, #13305, #20462 ) ;
#16091=CARTESIAN_POINT ( 'NONE',  ( -19.20225722901159315, -97.14187005060139768, 7.190316099514493686 ) ) ;
#16092=CARTESIAN_POINT ( 'NONE',  ( -20.54204892785229219, -95.55433702432603127, -9.451947527820101058 ) ) ;
#16094=CARTESIAN_POINT ( 'NONE',  ( 16.79424914329999652, -99.83167681540000160, 4.273280107039999720 ) ) ;
#16097=CARTESIAN_POINT ( 'NONE',  ( -23.69410997499999993, -94.52419709919999491, -3.934991024959999972 ) ) ;
#16099=DIRECTION ( 'NONE',  ( -2.370544285295434954E-14, -1.000000000000000000, 5.540271532162629942E-15 ) ) ;
#16101=CARTESIAN_POINT ( 'NONE',  ( -3.116266000930000057, -91.00000000000000000, -5.704286652290000426 ) ) ;
#16105=CARTESIAN_POINT ( 'NONE',  ( 23.24434528660000154, -94.16309976680000204, -7.473846836599999932 ) ) ;
#16108=CARTESIAN_POINT ( 'NONE',  ( -17.02652586798041412, -97.67115222923675333, 10.14659588024298209 ) ) ;
#16112=CARTESIAN_POINT ( 'NONE',  ( 8.002080211126466835, -101.4862650398017792, 13.99634146016975755 ) ) ;
#16113=FACE_OUTER_BOUND ( 'NONE', #20435, .T. ) ;
#16118=CARTESIAN_POINT ( 'NONE',  ( 27.03564186867965091, -92.52498922770500656, -14.11841734613871857 ) ) ;
#16119=EDGE_LOOP ( 'NONE', ( #1845, #2674, #15986, #21128 ) ) ;
#16120=EDGE_CURVE ( 'NONE', #4490, #4878, #11574, .T. ) ;
#16121=ADVANCED_FACE ( 'NONE', ( #2825 ), #7816, .F. ) ;
#16124=CARTESIAN_POINT ( 'NONE',  ( -2.545777994589999871, -97.01677120690000322, 20.99408306970000382 ) ) ;
#16125=CARTESIAN_POINT ( 'NONE',  ( 4.045673151789999089, -93.38241536079999605, 25.84256226979999838 ) ) ;
#16127=CARTESIAN_POINT ( 'NONE',  ( -25.76781702903437221, -94.10917102444695104, -2.365844001559266108 ) ) ;
#16133=CARTESIAN_POINT ( 'NONE',  ( -8.777511001860000661, -95.97839747389998877, -20.67514097709999987 ) ) ;
#16134=CARTESIAN_POINT ( 'NONE',  ( 7.279457176439408705, -101.1604341890527365, 13.52204713848896311 ) ) ;
#16140=CARTESIAN_POINT ( 'NONE',  ( 13.81414405219999963, -99.85455315880000171, -10.14094832980000049 ) ) ;
#16143=ORIENTED_EDGE ( 'NONE', *, *, #14787, .T. ) ;
#16144=CARTESIAN_POINT ( 'NONE',  ( -12.42556073345063261, -101.1604341566395107, -9.024505522341051744 ) ) ;
#16146=CARTESIAN_POINT ( 'NONE',  ( 0.2554224435499999890, -101.2010924020000004, -15.25977029010000052 ) ) ;
#16147=CARTESIAN_POINT ( 'NONE',  ( 23.98651103399999940, -93.13202907830000754, -10.86104031880000065 ) ) ;
#16148=ORIENTED_EDGE ( 'NONE', *, *, #14699, .F. ) ;
#16150=CARTESIAN_POINT ( 'NONE',  ( -7.498699138939999287, -94.79581646409999962, -22.45487619560000070 ) ) ;
#16153=CARTESIAN_POINT ( 'NONE',  ( 16.49344491490923303, -100.3041487037201449, 4.352733011544403396 ) ) ;
#16156=EDGE_CURVE ( 'NONE', #17343, #13209, #9023, .T. ) ;
#16157=B_SPLINE_SURFACE_WITH_KNOTS ( 'NONE', 5, 5, ( 
 ( #3586, #12181, #12591, #10264, #19175, #1696, #10405, #25880, #14785 ),
 ( #10123, #12321, #3869, #12733, #23686, #17126, #21646, #26014, #6038 ),
 ( #14924, #10532, #19449, #7701, #1154, #9991, #7829, #5493, #14382 ),
 ( #23276, #23416, #3319, #21227, #1281, #19039, #27925, #7962, #16852 ),
 ( #15062, #15196, #11109, #20029, #21783, #15647, #21934, #10965, #95 ),
 ( #4300, #23971, #2128, #28622, #1836, #15345, #6334, #24114, #28756 ),
 ( #22371, #4008, #17273, #13021, #4148, #8796, #26452, #26752, #6484 ),
 ( #22220, #17709, #8654, #2267, #17557, #8944, #17853, #26595, #10826 ),
 ( #6784, #24261, #24550, #13316, #13172, #6636, #4590, #19593, #13465 ) ),
 .UNSPECIFIED., .F., .F., .F.,
 ( 6, 3, 6 ),
 ( 6, 3, 6 ),
 ( 7.186332008689999995, 18.82032538949999889, 25.08217526769999850 ),
 ( 0.000000000000000000, 0.2500000000000000000, 0.5000000000000000000 ),
 .UNSPECIFIED. ) ;
#16162=ORIENTED_EDGE ( 'NONE', *, *, #18345, .T. ) ;
#16163=VECTOR ( 'NONE', #14489, 1000.000000000000000 ) ;
#16165=ORIENTED_EDGE ( 'NONE', *, *, #9439, .F. ) ;
#16171=CARTESIAN_POINT ( 'NONE',  ( 0.4184115225550000261, -93.00000000000000000, -30.38020727889999861 ) ) ;
#16173=CARTESIAN_POINT ( 'NONE',  ( -13.12479279440870350, -101.5902664364219135, -9.227018890821359065 ) ) ;
#16178=CARTESIAN_POINT ( 'NONE',  ( 22.78264860270000014, -94.59276292389999696, -6.873201011689999085 ) ) ;
#16184=DIRECTION ( 'NONE',  ( -0.9037419867099893978, 0.000000000000000000, 0.4280775881279952344 ) ) ;
#16185=ORIENTED_EDGE ( 'NONE', *, *, #1002, .T. ) ;
#16188=CARTESIAN_POINT ( 'NONE',  ( -18.19850021250000083, -94.71481160550000311, 16.19177116950000084 ) ) ;
#16197=B_SPLINE_CURVE_WITH_KNOTS ( 'NONE', 3,
 ( #26985, #7171, #487, #11364, #9180, #20269, #11052, #22169, #15891, #2208, #337, #37, #2803, #17798, #24942, #17654, #26689, #11657, #17945, #6730, #15596, #13408, #2357, #4835, #11510, #189, #18235, #26839, #6871, #15737, #13713, #11954, #14158 ),
 .UNSPECIFIED., .F., .F.,
 ( 4, 2, 1, 1, 2, 2, 1, 1, 1, 2, 2, 2, 1, 1, 2, 2, 1, 1, 2, 2, 4 ),
 ( 0.000000000000000000, 0.06249999999993549604, 0.09374999999991442956, 0.1093749999999134026, 0.1171874999999128891, 0.1249999999999123756, 0.1874999999998872846, 0.2187499999998759326, 0.2343749999998691325, 0.2421874999998724076, 0.2499999999998757105, 0.3749999999998923084, 0.4374999999998991362, 0.4687499999999059086, 0.4843749999999075739, 0.4999999999999092948, 0.6249999999999331646, 0.6874999999999445999, 0.7187499999999488187, 0.7499999999999531486, 1.000000000000000000 ),
 .UNSPECIFIED. ) ;
#16199=CARTESIAN_POINT ( 'NONE',  ( 14.82656590110000039, -97.01677250859999901, 15.07996639799999983 ) ) ;
#16204=CARTESIAN_POINT ( 'NONE',  ( -7.944280978800001058, -100.1981337080000003, 15.01052544650000087 ) ) ;
#16208=CARTESIAN_POINT ( 'NONE',  ( 7.286238495500000134, -101.2500498790000023, 13.33737010350000141 ) ) ;
#16212=CARTESIAN_POINT ( 'NONE',  ( 11.60189548900000034, -99.55619081909999579, -13.07744430270000002 ) ) ;
#16213=ORIENTED_EDGE ( 'NONE', *, *, #3350, .T. ) ;
#16215=CARTESIAN_POINT ( 'NONE',  ( 11.90107424179999995, -101.3957169669999985, -10.67378013559999950 ) ) ;
#16217=CARTESIAN_POINT ( 'NONE',  ( 14.81349357762022478, -95.37019131402171013, 17.32245915622085519 ) ) ;
#16218=ADVANCED_FACE ( 'NONE', ( #7907 ), #4992, .F. ) ;
#16219=EDGE_CURVE ( 'NONE', #26789, #15187, #11848, .T. ) ;
#16226=CARTESIAN_POINT ( 'NONE',  ( 6.901963694340000011, -101.4908759489999994, 14.46911387129999937 ) ) ;
#16228=AXIS2_PLACEMENT_3D ( 'NONE', #2104, #6759, #24084 ) ;
#16229=CARTESIAN_POINT ( 'NONE',  ( 7.640382384829999651, -101.0974005930000033, 13.42254915319999853 ) ) ;
#16234=CARTESIAN_POINT ( 'NONE',  ( 2.412292587909999959E-12, -111.0000000000000000, -5.497824417940001177E-12 ) ) ;
#16237=CARTESIAN_POINT ( 'NONE',  ( 16.78053306740000039, -99.78393592979999482, 4.299646967080000159 ) ) ;
#16238=ORIENTED_EDGE ( 'NONE', *, *, #4571, .F. ) ;
#16240=CARTESIAN_POINT ( 'NONE',  ( 8.140397668380000340, -100.8869818179999953, 13.38618156149999905 ) ) ;
#16242=VERTEX_POINT ( 'NONE', #4518 ) ;
#16243=CARTESIAN_POINT ( 'NONE',  ( 9.127577618711740115, -92.82334897400379248, 29.10218788055306405 ) ) ;
#16247=CARTESIAN_POINT ( 'NONE',  ( 0.6074919593152650066, -100.4872618012716288, -16.90062116310696894 ) ) ;
#16248=DIRECTION ( 'NONE',  ( 0.4794255386042041156, 0.000000000000000000, 0.8775825618903722036 ) ) ;
#16252=EDGE_CURVE ( 'NONE', #24500, #15581, #3475, .T. ) ;
#16255=CARTESIAN_POINT ( 'NONE',  ( 13.89851760690000049, -96.93384555689999615, -16.12486289770000170 ) ) ;
#16263=EDGE_LOOP ( 'NONE', ( #10180, #5712, #15032, #6778 ) ) ;
#16264=VECTOR ( 'NONE', #19838, 1000.000000000000000 ) ;
#16267=CARTESIAN_POINT ( 'NONE',  ( 6.981684465299999864, -101.1889999979999999, 29.03810821740000137 ) ) ;
#16268=CARTESIAN_POINT ( 'NONE',  ( -0.8119073803659999644, -95.90105813370000476, 22.89043856289999823 ) ) ;
#16269=CARTESIAN_POINT ( 'NONE',  ( 5.686419033639999121, -92.95927362729999288, 26.23007088160000322 ) ) ;
#16290=CARTESIAN_POINT ( 'NONE',  ( -15.55924707670000018, -101.2720154369999932, 3.463031180029999767 ) ) ;
#16294=DIRECTION ( 'NONE',  ( 1.000000000000000000, 0.000000000000000000, 0.000000000000000000 ) ) ;
#16296=CARTESIAN_POINT ( 'NONE',  ( 24.12664335590000064, -92.56290624670000966, -15.50499703690000075 ) ) ;
#16297=VERTEX_POINT ( 'NONE', #20817 ) ;
#16298=CARTESIAN_POINT ( 'NONE',  ( -8.594687425180000062, -94.47838212999999996, -22.80941933420000112 ) ) ;
#16301=CARTESIAN_POINT ( 'NONE',  ( 16.83483077069999823, -99.92967571559999840, 4.239603657359999112 ) ) ;
#16309=CARTESIAN_POINT ( 'NONE',  ( 3.812263950998352691, -93.98965247056261774, 25.83266599306846700 ) ) ;
#16314=CARTESIAN_POINT ( 'NONE',  ( 11.70455088819999823, -92.50000000000000000, 8.942783294160001617 ) ) ;
#16316=CARTESIAN_POINT ( 'NONE',  ( -5.761619419100000528, -101.1130130960000031, 14.30911249059999868 ) ) ;
#16329=DIRECTION ( 'NONE',  ( 1.000000000000000000, 0.000000000000000000, 0.000000000000000000 ) ) ;
#16330=CARTESIAN_POINT ( 'NONE',  ( 13.12744653600000078, -94.59276292389999696, -19.84842857619999990 ) ) ;
#16340=CARTESIAN_POINT ( 'NONE',  ( -18.00116235329999625, -97.01638956499999722, 11.09997051220000053 ) ) ;
#16346=B_SPLINE_CURVE_WITH_KNOTS ( 'NONE', 3,
 ( #25761, #23845, #8248, #12202, #3748, #16729, #19337, #26181, #21379, #27946, #16874, #5790, #14674, #23568, #21522, #1579, #10420 ),
 .UNSPECIFIED., .F., .F.,
 ( 4, 2, 2, 1, 1, 1, 1, 1, 2, 2, 4 ),
 ( 0.000000000000000000, 0.2500000000000119904, 0.3750000000000182077, 0.4375000000000205391, 0.4687500000000224820, 0.4843750000000234812, 0.4921875000000247025, 0.4960937500000253686, 0.4980468750000248690, 0.5000000000000244249, 1.000000000000000000 ),
 .UNSPECIFIED. ) ;
#16348=CARTESIAN_POINT ( 'NONE',  ( 8.354902469970001633, -98.70454033420000428, 16.50015517690000166 ) ) ;
#16352=CARTESIAN_POINT ( 'NONE',  ( 19.58569113819999785, -94.54719592040000009, 13.61988814439999906 ) ) ;
#16356=DIRECTION ( 'NONE',  ( 0.000000000000000000, 1.000000000000000000, 0.000000000000000000 ) ) ;
#16362=CARTESIAN_POINT ( 'NONE',  ( 7.601924345689999640, -101.4240865590000027, 14.04435494200000001 ) ) ;
#16364=EDGE_CURVE ( 'NONE', #7118, #3430, #14514, .T. ) ;
#16366=DIRECTION ( 'NONE',  ( 0.000000000000000000, -1.000000000000000000, 0.000000000000000000 ) ) ;
#16367=CARTESIAN_POINT ( 'NONE',  ( 11.43947858090000125, -98.26007807919999948, -15.36247001880000163 ) ) ;
#16370=CARTESIAN_POINT ( 'NONE',  ( 11.97711149329999891, -101.3256027139999986, -10.46763994119999985 ) ) ;
#16372=CARTESIAN_POINT ( 'NONE',  ( -17.05616532261941742, -92.82529299097730302, 25.28511888657223139 ) ) ;
#16376=DIRECTION ( 'NONE',  ( 1.000000000000000000, 0.000000000000000000, 0.000000000000000000 ) ) ;
#16380=B_SPLINE_CURVE_WITH_KNOTS ( 'NONE', 3,
 ( #19997, #4270, #1956, #70, #6609, #13290, #24236, #10800, #8766, #4121, #19710, #8491, #12994, #8916, #22194, #3845, #2235, #11080, #17679, #26567, #12844, #8625, #17391, #1675, #26285, #28728, #28308, #8342, #21758, #13145, #26423, #24377, #12709, #26719, #28597, #21624, #17247, #17825, #19845, #10512, #17533, #19428, #10651, #19568, #26139, #15034, #17970, #2539, #7052, #20446, #22341, #362, #221, #27010, #20150, #9067, #13741, #22641, #2680, #516 ),
 .UNSPECIFIED., .F., .F.,
 ( 4, 2, 1, 1, 2, 2, 2, 2, 1, 1, 2, 2, 2, 2, 2, 2, 2, 1, 1, 2, 2, 2, 2, 1, 2, 2, 2, 1, 2, 2, 2, 2, 2, 4 ),
 ( 0.000000000000000000, 0.06250000000003833045, 0.09375000000005272172, 0.1093750000000599104, 0.1171875000000641293, 0.1250000000000683342, 0.1875000000000456302, 0.2187500000000350553, 0.2343750000000292821, 0.2421875000000203448, 0.2460937500000166256, 0.2500000000000128786, 0.3124999999999367173, 0.3437499999998986921, 0.3749999999998606115, 0.4374999999997844502, 0.4687499999997468692, 0.4843749999997351008, 0.4921874999997297162, 0.4960937499997356559, 0.4999999999997415956, 0.5624999999997376543, 0.5937499999997348787, 0.6093749999997334355, 0.6171874999997395417, 0.6249999999997456479, 0.6874999999997927214, 0.7187499999998162581, 0.7343749999998224753, 0.7499999999998285816, 0.8124999999998643307, 0.8437499999998877565, 0.8749999999999110711, 1.000000000000000000 ),
 .UNSPECIFIED. ) ;
#16388=FACE_OUTER_BOUND ( 'NONE', #7010, .T. ) ;
#16390=DIRECTION ( 'NONE',  ( 0.000000000000000000, 1.000000000000000000, 0.000000000000000000 ) ) ;
#16391=ORIENTED_EDGE ( 'NONE', *, *, #17445, .F. ) ;
#16393=B_SPLINE_CURVE_WITH_KNOTS ( 'NONE', 3,
 ( #18672, #10033, #1198, #27570, #7611, #16173, #13999, #18947, #27831, #23464, #5263, #3503 ),
 .UNSPECIFIED., .F., .F.,
 ( 4, 2, 2, 2, 2, 4 ),
 ( 0.000000000000000000, 0.2499999999999856781, 0.3749999999999847344, 0.4374999999999733546, 0.4999999999999619194, 1.000000000000000000 ),
 .UNSPECIFIED. ) ;
#16394=CARTESIAN_POINT ( 'NONE',  ( -24.07228109569999930, -94.80026829410000744, -4.144186737870000137 ) ) ;
#16401=CARTESIAN_POINT ( 'NONE',  ( 0.4381803858471648438, -99.99762666406154210, -17.29986369493340703 ) ) ;
#16404=CARTESIAN_POINT ( 'NONE',  ( -11.94559458280000008, -100.4792519539999915, -10.93369168340000108 ) ) ;
#16407=CARTESIAN_POINT ( 'NONE',  ( 13.60163640490000070, -95.66919271840001215, -17.93630288140000317 ) ) ;
#16414=ORIENTED_EDGE ( 'NONE', *, *, #4334, .F. ) ;
#16415=CARTESIAN_POINT ( 'NONE',  ( -2.796429754430000392E-12, -111.0000000000000000, -5.314859663490001141E-12 ) ) ;
#16421=CARTESIAN_POINT ( 'NONE',  ( -2.332908480600000001, -96.95622424260000116, 20.76785060539999961 ) ) ;
#16422=CARTESIAN_POINT ( 'NONE',  ( 11.27141356559999963, -93.01024347330000808, 27.60408353590000274 ) ) ;
#16426=CARTESIAN_POINT ( 'NONE',  ( -29.71161737690000137, -93.00000000000000000, 6.352311025380000586 ) ) ;
#16435=DIRECTION ( 'NONE',  ( 0.7887177114147766455, 0.000000000000000000, 0.6147555381618264869 ) ) ;
#16441=CARTESIAN_POINT ( 'NONE',  ( -6.781378104809999030, -101.1889999979999999, 14.49182221120000058 ) ) ;
#16442=CARTESIAN_POINT ( 'NONE',  ( -16.71474937220000001, -100.0946963879999885, 3.139046040560000250 ) ) ;
#16446=CARTESIAN_POINT ( 'NONE',  ( 11.70455088819999823, -111.0000000000000000, 8.942783294160001617 ) ) ;
#16449=ORIENTED_EDGE ( 'NONE', *, *, #22051, .F. ) ;
#16451=ADVANCED_FACE ( 'NONE', ( #27197 ), #22537, .T. ) ;
#16453=LINE ( 'NONE', #16735, #8380 ) ;
#16455=CARTESIAN_POINT ( 'NONE',  ( 16.20256441434644401, -100.6644468685070279, 4.326382415546095039 ) ) ;
#16467=CARTESIAN_POINT ( 'NONE',  ( -5.909348975229999468, -101.1659666750000071, 14.88340913230000062 ) ) ;
#16472=VECTOR ( 'NONE', #13158, 1000.000000000000000 ) ;
#16476=CARTESIAN_POINT ( 'NONE',  ( 7.286238495500000134, -101.2500498790000023, 13.33737010350000141 ) ) ;
#16480=CARTESIAN_POINT ( 'NONE',  ( 19.91489110990000100, -97.53592492930000901, 2.489640473879999760 ) ) ;
#16481=CARTESIAN_POINT ( 'NONE',  ( -20.43932690519999795, -94.59275946379999311, 12.18704468149999975 ) ) ;
#16482=CARTESIAN_POINT ( 'NONE',  ( 24.01308102359999808, -93.00000902169999506, -18.61461954819999676 ) ) ;
#16488=FACE_OUTER_BOUND ( 'NONE', #11986, .T. ) ;
#16489=CARTESIAN_POINT ( 'NONE',  ( 0.9512194931930000319, -99.70407914540000149, -17.16990763940000164 ) ) ;
#16495=EDGE_CURVE ( 'NONE', #13319, #20241, #264, .T. ) ;
#16499=ADVANCED_FACE ( 'NONE', ( #18454 ), #10865, .F. ) ;
#16501=FACE_OUTER_BOUND ( 'NONE', #19364, .T. ) ;
#16503=CARTESIAN_POINT ( 'NONE',  ( 7.292753731799999528, -92.50000000000000000, -29.01615345709999971 ) ) ;
#16504=VERTEX_POINT ( 'NONE', #11127 ) ;
#16507=CARTESIAN_POINT ( 'NONE',  ( -18.08359759629999886, -92.56168670950000887, -23.48371534130000171 ) ) ;
#16511=CARTESIAN_POINT ( 'NONE',  ( 7.252148862920000383, -101.2521831870000142, 13.35282088509999987 ) ) ;
#16512=ORIENTED_EDGE ( 'NONE', *, *, #9543, .T. ) ;
#16514=CARTESIAN_POINT ( 'NONE',  ( -29.77335029849999870, -92.50000460620000808, -0.5783696374510000071 ) ) ;
#16516=CARTESIAN_POINT ( 'NONE',  ( 11.21565222179999921, -96.96081043319999537, -17.72906860990000411 ) ) ;
#16518=AXIS2_PLACEMENT_3D ( 'NONE', #11855, #20460, #15930 ) ;
#16520=CARTESIAN_POINT ( 'NONE',  ( 11.97277113790000058, -101.5369810359999860, -10.61440544620000104 ) ) ;
#16526=CARTESIAN_POINT ( 'NONE',  ( 13.77871658040979419, -98.12113978595867536, 15.06064669432830705 ) ) ;
#16527=CARTESIAN_POINT ( 'NONE',  ( -16.97397862119999701, -99.68179698959998802, 2.927883187840000012 ) ) ;
#16528=VERTEX_POINT ( 'NONE', #11428 ) ;
#16529=EDGE_CURVE ( 'NONE', #19071, #20556, #19294, .T. ) ;
#16532=AXIS2_PLACEMENT_3D ( 'NONE', #11869, #11718, #22970 ) ;
#16534=CARTESIAN_POINT ( 'NONE',  ( -11.18841398930000075, -94.77531363049999413, -20.78536845970000257 ) ) ;
#16539=CARTESIAN_POINT ( 'NONE',  ( 23.58466923419999972, -94.98812477769999418, -2.405350023570000051 ) ) ;
#16540=CARTESIAN_POINT ( 'NONE',  ( -20.54445053870980686, -93.08694455160939185, -20.58885575223966669 ) ) ;
#16541=DIRECTION ( 'NONE',  ( 0.000000000000000000, 1.000000000000000000, 0.000000000000000000 ) ) ;
#16548=CARTESIAN_POINT ( 'NONE',  ( 0.5866164698262277266, -100.8738282930437720, -16.59383815637838566 ) ) ;
#16551=CARTESIAN_POINT ( 'NONE',  ( -12.45019672459999960, -94.16701134360000935, -21.10503017290000116 ) ) ;
#16555=CARTESIAN_POINT ( 'NONE',  ( 23.85248605308397885, -92.80442066019703873, -19.00813913752200790 ) ) ;
#16559=SURFACE_STYLE_USAGE ( .BOTH. , #7695 ) ;
#16563=ORIENTED_EDGE ( 'NONE', *, *, #4617, .T. ) ;
#16564=EDGE_CURVE ( 'NONE', #3430, #18376, #28736, .T. ) ;
#16571=CARTESIAN_POINT ( 'NONE',  ( -28.88915324434640652, -93.08996811601012666, 3.176849059424360355 ) ) ;
#16582=CARTESIAN_POINT ( 'NONE',  ( -14.42556421679999978, -93.00000000000000000, -2.978755036369999942 ) ) ;
#16583=CARTESIAN_POINT ( 'NONE',  ( -14.88703466399999975, -101.2270092189999957, 3.209821742049999926 ) ) ;
#16588=CARTESIAN_POINT ( 'NONE',  ( 0.000000000000000000, -102.8486084350000027, 0.000000000000000000 ) ) ;
#16590=CARTESIAN_POINT ( 'NONE',  ( -7.905721070053497002, -100.3617719037266767, 15.06330732917539095 ) ) ;
#16592=EDGE_CURVE ( 'NONE', #10781, #8949, #5138, .T. ) ;
#16614=ORIENTED_EDGE ( 'NONE', *, *, #217, .T. ) ;
#16616=CARTESIAN_POINT ( 'NONE',  ( 10.49047210377122497, -92.65509297689168022, -25.64082608166361155 ) ) ;
#16617=CARTESIAN_POINT ( 'NONE',  ( -20.45316973280000283, -93.85308800720000022, 14.21304034189999932 ) ) ;
#16618=CARTESIAN_POINT ( 'NONE',  ( 0.000000000000000000, -108.5000000000000000, 0.000000000000000000 ) ) ;
#16619=VERTEX_POINT ( 'NONE', #10659 ) ;
#16625=DIRECTION ( 'NONE',  ( 0.000000000000000000, -1.000000000000000000, 0.000000000000000000 ) ) ;
#16635=TOROIDAL_SURFACE ( 'NONE', #4519, 16.50000000000000000, 5.500000000000000000 ) ;
#16638=EDGE_LOOP ( 'NONE', ( #24081, #2069, #1230, #11769 ) ) ;
#16641=ADVANCED_FACE ( 'NONE', ( #13001 ), #27345, .T. ) ;
#16642=CARTESIAN_POINT ( 'NONE',  ( 0.000000000000000000, -92.50000000000000000, 0.000000000000000000 ) ) ;
#16649=CARTESIAN_POINT ( 'NONE',  ( -28.39500908420000158, -92.99999854809999533, -2.401901190519999840 ) ) ;
#16650=CARTESIAN_POINT ( 'NONE',  ( 10.69569866790000034, -95.98460637910000059, -20.33107714349999995 ) ) ;
#16659=AXIS2_PLACEMENT_3D ( 'NONE', #21699, #19508, #20095 ) ;
#16664=CARTESIAN_POINT ( 'NONE',  ( 6.963769279919999278, -101.5216621940000152, 14.41672748959999950 ) ) ;
#16665=DIRECTION ( 'NONE',  ( 1.000000000000000000, 0.000000000000000000, 0.000000000000000000 ) ) ;
#16666=CARTESIAN_POINT ( 'NONE',  ( 7.358959778060000012, -101.1389411659999951, 13.51882459459999986 ) ) ;
#16667=AXIS2_PLACEMENT_3D ( 'NONE', #22275, #24461, #26950 ) ;
#16668=CARTESIAN_POINT ( 'NONE',  ( -11.56445414979999953, -94.58710607640000489, -20.95866303660000085 ) ) ;
#16671=CARTESIAN_POINT ( 'NONE',  ( 23.95218086839091498, -94.65677004896707558, -2.989273988903572210 ) ) ;
#16673=DIRECTION ( 'NONE',  ( 0.000000000000000000, 1.000000000000000000, 0.000000000000000000 ) ) ;
#16676=CARTESIAN_POINT ( 'NONE',  ( 12.01505635090000190, -101.1292389600000092, -9.802278386409998490 ) ) ;
#16681=CARTESIAN_POINT ( 'NONE',  ( 0.4132369963184429618, -99.96200787827957868, -17.32932737678238055 ) ) ;
#16684=CARTESIAN_POINT ( 'NONE',  ( -14.04223022189999881, -93.60790942709999740, -21.24517368629999936 ) ) ;
#16685=ADVANCED_FACE ( 'NONE', ( #27016 ), #9155, .T. ) ;
#16687=EDGE_CURVE ( 'NONE', #16053, #10781, #12294, .T. ) ;
#16688=CIRCLE ( 'NONE', #1796, 13.13304743849999845 ) ;
#16691=CARTESIAN_POINT ( 'NONE',  ( 26.66586753799999698, -92.50000000000000000, 13.56661073689999952 ) ) ;
#16699=B_SPLINE_CURVE_WITH_KNOTS ( 'NONE', 5,
 ( #6027, #19165, #1684, #8220, #23263, #12170, #7818, #9982, #27915 ),
 .UNSPECIFIED., .F., .F.,
 ( 6, 3, 6 ),
 ( 0.000000000000000000, 0.5000000000000000000, 1.000000000000000000 ),
 .UNSPECIFIED. ) ;
#16703=CYLINDRICAL_SURFACE ( 'NONE', #9757, 0.7999999999999994893 ) ;
#16712=EDGE_CURVE ( 'NONE', #22101, #21750, #2544, .T. ) ;
#16713=CARTESIAN_POINT ( 'NONE',  ( 0.000000000000000000, -108.5000000000000000, 0.000000000000000000 ) ) ;
#16718=CARTESIAN_POINT ( 'NONE',  ( 27.23270669000000055, -92.50000467790000869, -12.38956474639999961 ) ) ;
#16723=CARTESIAN_POINT ( 'NONE',  ( -14.68103708169999955, -101.1848540220000103, 4.247747895729999890 ) ) ;
#16724=CARTESIAN_POINT ( 'NONE',  ( -16.65233384409999928, -100.4382163219999882, 3.162646594119999932 ) ) ;
#16729=CARTESIAN_POINT ( 'NONE',  ( 19.66608320708412805, -98.68740020691039661, -0.5966002485424611868 ) ) ;
#16733=CIRCLE ( 'NONE', #25583, 6.000000000000000000 ) ;
#16735=CARTESIAN_POINT ( 'NONE',  ( -14.62247892739999955, -91.50000000000000000, -26.76626813769999913 ) ) ;
#16740=CARTESIAN_POINT ( 'NONE',  ( 6.838213422042789702, -100.3796496173189894, 15.56132088991555129 ) ) ;
#16742=EDGE_LOOP ( 'NONE', ( #18738, #27580, #23046, #21002 ) ) ;
#16744=ORIENTED_EDGE ( 'NONE', *, *, #17606, .T. ) ;
#16745=CARTESIAN_POINT ( 'NONE',  ( 28.56683165460000140, -92.91851489520000484, 8.527576185230000050 ) ) ;
#16746=CARTESIAN_POINT ( 'NONE',  ( -6.249265825439999311, -101.3256027139999986, 14.62769162600000072 ) ) ;
#16749=DIRECTION ( 'NONE',  ( 0.4794255386042041156, 0.000000000000000000, 0.8775825618903722036 ) ) ;
#16752=ORIENTED_EDGE ( 'NONE', *, *, #18745, .F. ) ;
#16754=CARTESIAN_POINT ( 'NONE',  ( 16.77269055116476792, -99.57060688044040830, 4.505412732972978951 ) ) ;
#16756=ORIENTED_EDGE ( 'NONE', *, *, #397, .T. ) ;
#16757=CARTESIAN_POINT ( 'NONE',  ( -16.98465565300000080, -97.93128678269999909, -10.56456529129999922 ) ) ;
#16762=B_SPLINE_CURVE_WITH_KNOTS ( 'NONE', 5,
 ( #14430, #23321, #5947, #1886, #10723, #12496, #6380, #12637, #1736 ),
 .UNSPECIFIED., .F., .F.,
 ( 6, 3, 6 ),
 ( 0.000000000000000000, 0.5240999523975469199, 1.000000000000000000 ),
 .UNSPECIFIED. ) ;
#16765=EDGE_LOOP ( 'NONE', ( #10913, #2105 ) ) ;
#16766=CARTESIAN_POINT ( 'NONE',  ( -30.31271238969999970, -93.00000000000000000, 0.1252161350790000072 ) ) ;
#16769=DIRECTION ( 'NONE',  ( 0.9397523434780248319, 0.000000000000000000, 0.3418560119810096221 ) ) ;
#16770=DIRECTION ( 'NONE',  ( 0.000000000000000000, 1.000000000000000000, 0.000000000000000000 ) ) ;
#16773=AXIS2_PLACEMENT_3D ( 'NONE', #27997, #3801, #8035 ) ;
#16780=CARTESIAN_POINT ( 'NONE',  ( 12.82422237299999956, -94.98812477769999418, -19.93894812050000098 ) ) ;
#16782=CARTESIAN_POINT ( 'NONE',  ( -13.14541460800000117, -101.3350617309999961, -9.160026903060000336 ) ) ;
#16783=CARTESIAN_POINT ( 'NONE',  ( -29.21843812340000213, -93.00000000000000000, 6.434616699369999360 ) ) ;
#16784=ADVANCED_FACE ( 'NONE', ( #22943 ), #2568, .F. ) ;
#16786=CARTESIAN_POINT ( 'NONE',  ( -7.930433002940000975, -100.4731125450000064, 14.12856493100000144 ) ) ;
#16788=CARTESIAN_POINT ( 'NONE',  ( 1.869767860340000087, -92.87437365140000622, 27.35099196270000022 ) ) ;
#16790=CARTESIAN_POINT ( 'NONE',  ( -13.55269044519999966, -101.1889999979999999, -9.843123574170000722 ) ) ;
#16792=CARTESIAN_POINT ( 'NONE',  ( 7.383226538699999786, -101.1286588279999989, 13.63651901270000089 ) ) ;
#16797=CARTESIAN_POINT ( 'NONE',  ( -22.24124310690000073, -94.63960343439998724, -8.291373264160000645 ) ) ;
#16801=CARTESIAN_POINT ( 'NONE',  ( 11.29156748259999965, -101.1516803200000112, -10.36374020140000063 ) ) ;
#16803=CARTESIAN_POINT ( 'NONE',  ( -17.48893075979999878, -94.09609773500001495, 17.08751209079999711 ) ) ;
#16804=CARTESIAN_POINT ( 'NONE',  ( -18.08183833912162441, -92.54893169919637330, 24.56210854116960718 ) ) ;
#16806=CARTESIAN_POINT ( 'NONE',  ( -0.03272619456850000413, -101.4121386959999995, -15.97721227889999795 ) ) ;
#16812=CARTESIAN_POINT ( 'NONE',  ( 6.324210420500000929, -100.7833805400000102, 14.60206476039999934 ) ) ;
#16816=CIRCLE ( 'NONE', #20049, 4.999999999999999112 ) ;
#16817=CARTESIAN_POINT ( 'NONE',  ( -11.55953761080000142, -94.64048054399999899, -21.16633973740000130 ) ) ;
#16821=EDGE_CURVE ( 'NONE', #4122, #10810, #20733, .T. ) ;
#16822=DIRECTION ( 'NONE',  ( 0.000000000000000000, 1.000000000000000000, 0.000000000000000000 ) ) ;
#16825=B_SPLINE_SURFACE_WITH_KNOTS ( 'NONE', 5, 5, ( 
 ( #13782, #4609, #410, #24425, #9261, #2438 ),
 ( #22683, #8966, #11292, #20491, #562, #28777 ),
 ( #4463, #13331, #22238, #11133, #14080, #7815 ),
 ( #16255, #998, #3032, #709, #14370, #18609 ),
 ( #12169, #27648, #9694, #16407, #23262, #27500 ),
 ( #5483, #7550, #12022, #21083, #7390, #1143 ) ),
 .UNSPECIFIED., .F., .F., .F.,
 ( 6, 6 ),
 ( 6, 6 ),
 ( 15.82768567779999991, 30.79603606440000263 ),
 ( 0.000000000000000000, 0.5000000000000000000 ),
 .UNSPECIFIED. ) ;
#16830=DIRECTION ( 'NONE',  ( 0.000000000000000000, -1.000000000000000000, 0.000000000000000000 ) ) ;
#16833=CARTESIAN_POINT ( 'NONE',  ( 0.5946929504664082433, -100.4010812937833350, -16.96993233685614300 ) ) ;
#16834=FACE_OUTER_BOUND ( 'NONE', #24267, .T. ) ;
#16835=CARTESIAN_POINT ( 'NONE',  ( 13.94204884902214658, -92.53260370676606783, 27.12694900991376912 ) ) ;
#16840=CARTESIAN_POINT ( 'NONE',  ( 11.83146313070000133, -101.1461874320000049, -11.00634697169999932 ) ) ;
#16852=CARTESIAN_POINT ( 'NONE',  ( -27.80414915030000245, -92.67327634539999792, 1.811697503490000027 ) ) ;
#16857=ORIENTED_EDGE ( 'NONE', *, *, #26998, .F. ) ;
#16858=CARTESIAN_POINT ( 'NONE',  ( -28.76693335801717666, -93.11247489672756217, 2.840853404041298713 ) ) ;
#16867=CARTESIAN_POINT ( 'NONE',  ( -15.38068916850000001, -101.6095197629999944, 4.516181925269999731 ) ) ;
#16868=CARTESIAN_POINT ( 'NONE',  ( -16.12803325799999854, -100.3774201490000024, 2.700167859220000022 ) ) ;
#16870=CARTESIAN_POINT ( 'NONE',  ( -6.143223556138350361, -101.1586404113043898, 14.37947789112424601 ) ) ;
#16871=AXIS2_PLACEMENT_3D ( 'NONE', #22973, #3018, #5032 ) ;
#16872=ORIENTED_EDGE ( 'NONE', *, *, #4281, .T. ) ;
#16874=CARTESIAN_POINT ( 'NONE',  ( 20.39783485576944599, -98.09459568642344607, -1.420636912331782353 ) ) ;
#16878=CARTESIAN_POINT ( 'NONE',  ( -7.286203202325246764, -101.4304678898307372, 14.43370055275712183 ) ) ;
#16886=CARTESIAN_POINT ( 'NONE',  ( 6.664891844591124936, -100.9229461904473339, 15.16559953918201664 ) ) ;
#16890=CARTESIAN_POINT ( 'NONE',  ( -17.12548553040000243, -99.53431416519998720, 3.156821174210000081 ) ) ;
#16891=ORIENTED_EDGE ( 'NONE', *, *, #26187, .T. ) ;
#16893=CARTESIAN_POINT ( 'NONE',  ( 28.28014364260000235, -92.50732182220001221, 8.299785262969999522 ) ) ;
#16897=CARTESIAN_POINT ( 'NONE',  ( -28.39367414323790229, -93.04141874247781629, -2.227239965210703776 ) ) ;
#16902=EDGE_LOOP ( 'NONE', ( #10752, #20405, #8000, #27717, #3874, #9574, #3310 ) ) ;
#16903=CARTESIAN_POINT ( 'NONE',  ( -20.55443039410000239, -95.85308664750000673, -9.151112246150001184 ) ) ;
#16904=CARTESIAN_POINT ( 'NONE',  ( 15.75263236761972863, -101.6484611539999747, 2.803083806627801433 ) ) ;
#16905=CARTESIAN_POINT ( 'NONE',  ( -20.44152562849999910, -92.68419405429999358, 18.52892094230000097 ) ) ;
#16906=CARTESIAN_POINT ( 'NONE',  ( 24.47825540369999686, -92.91851489729999969, -17.01759270650000033 ) ) ;
#16908=CARTESIAN_POINT ( 'NONE',  ( 29.75862214763936819, -92.72722989466579691, 6.683900548007907894 ) ) ;
#16911=DIRECTION ( 'NONE',  ( 0.6601796052711899065, 0.000000000000000000, -0.7511077744132169665 ) ) ;
#16915=AXIS2_PLACEMENT_3D ( 'NONE', #17901, #7125, #296 ) ;
#16926=CARTESIAN_POINT ( 'NONE',  ( -12.96048168789999977, -101.0356131030000029, -8.456406562079997968 ) ) ;
#16927=DIRECTION ( 'NONE',  ( -0.1646113479699435889, 0.000000000000000000, 0.9863585068926603583 ) ) ;
#16929=CARTESIAN_POINT ( 'NONE',  ( -7.941456924969999775, -100.0994409990000094, 15.28316630279999977 ) ) ;
#16931=CARTESIAN_POINT ( 'NONE',  ( -0.009295818923119999674, -93.24058218830001010, 26.19215823259999709 ) ) ;
#16932=CARTESIAN_POINT ( 'NONE',  ( -8.394720798919559357, -94.58015680889037924, -22.73927332636950993 ) ) ;
#16937=CARTESIAN_POINT ( 'NONE',  ( 12.67863569023319492, -101.5409490182417329, -9.895065346989536437 ) ) ;
#16941=CARTESIAN_POINT ( 'NONE',  ( 7.007938636740000504, -99.64579651319999698, 15.84020959899999959 ) ) ;
#16945=DIRECTION ( 'NONE',  ( 1.000000000000000000, 0.000000000000000000, 0.000000000000000000 ) ) ;
#16948=AXIS2_PLACEMENT_3D ( 'NONE', #7071, #23099, #2844 ) ;
#16957=CARTESIAN_POINT ( 'NONE',  ( 6.630693261409999373, -100.8088109309999965, 15.16285646280000066 ) ) ;
#16958=CARTESIAN_POINT ( 'NONE',  ( 15.04054737160000066, -101.1411470200000053, 3.257342712189999823 ) ) ;
#16959=CARTESIAN_POINT ( 'NONE',  ( -5.819199518928550141, -97.34036579023693037, 19.85381770611325791 ) ) ;
#16962=CARTESIAN_POINT ( 'NONE',  ( 5.003143695574637562, -92.66972459460949096, -30.08685070979726817 ) ) ;
#16964=CARTESIAN_POINT ( 'NONE',  ( -6.670601060500000123, -97.64874574759998893, 18.82504149280000050 ) ) ;
#16965=CARTESIAN_POINT ( 'NONE',  ( 6.598815769619999827, -93.39359504719999450, -26.37745322970000217 ) ) ;
#16970=CARTESIAN_POINT ( 'NONE',  ( -17.12548553040000243, -99.53431416519998720, 3.156821174210000081 ) ) ;
#16972=CARTESIAN_POINT ( 'NONE',  ( -1.060320034430000113, -101.4334236450000049, -16.03230495190000227 ) ) ;
#16975=DIRECTION ( 'NONE',  ( 0.000000000000000000, -1.000000000000000000, 0.000000000000000000 ) ) ;
#16977=CARTESIAN_POINT ( 'NONE',  ( 15.82549146240000049, -101.1976625110000043, 4.106801947200000136 ) ) ;
#16978=CARTESIAN_POINT ( 'NONE',  ( -8.306762876789999694, -99.70407914540000149, 15.05683357740000083 ) ) ;
#16980=AXIS2_PLACEMENT_3D ( 'NONE', #14854, #8293, #12799 ) ;
#16981=CARTESIAN_POINT ( 'NONE',  ( 11.33780648110000122, -100.8733988930000010, -10.89600415129999966 ) ) ;
#16996=ORIENTED_EDGE ( 'NONE', *, *, #8198, .T. ) ;
#17007=CARTESIAN_POINT ( 'NONE',  ( -12.46057752100000116, -101.1191090859999946, -10.51508789569999891 ) ) ;
#17010=CARTESIAN_POINT ( 'NONE',  ( -7.888607335952146471, -100.4507315480479548, 14.99179633818354240 ) ) ;
#17018=CARTESIAN_POINT ( 'NONE',  ( 6.661181729204114887, -100.9609609850482883, 15.13455079199698083 ) ) ;
#17020=CARTESIAN_POINT ( 'NONE',  ( 11.49573228323775531, -101.1962283502455335, -10.04692880049169013 ) ) ;
#17021=ORIENTED_EDGE ( 'NONE', *, *, #1470, .T. ) ;
#17022=CARTESIAN_POINT ( 'NONE',  ( -18.13582102693932896, -98.48184326581569792, 4.852288895080256736 ) ) ;
#17024=CARTESIAN_POINT ( 'NONE',  ( 27.05235185969999634, -92.55031885960001148, 9.384696477129999437 ) ) ;
#17026=CARTESIAN_POINT ( 'NONE',  ( 4.226834115039999951, -93.34497626389999425, 25.39917024580000060 ) ) ;
#17030=EDGE_LOOP ( 'NONE', ( #186, #2820, #26173, #19342 ) ) ;
#17031=CARTESIAN_POINT ( 'NONE',  ( 24.01307781190000057, -93.00000000000000000, -18.61462211579999959 ) ) ;
#17032=CARTESIAN_POINT ( 'NONE',  ( 7.500294343269999331, -101.1699703470000031, 13.83260060669999980 ) ) ;
#17035=EDGE_CURVE ( 'NONE', #3774, #13014, #13721, .T. ) ;
#17037=CARTESIAN_POINT ( 'NONE',  ( 13.31770606849999972, -100.4792519539999915, -9.213118301410000655 ) ) ;
#17038=CARTESIAN_POINT ( 'NONE',  ( -16.54318588419999969, -93.00000000000000000, 25.62368046950000178 ) ) ;
#17039=CARTESIAN_POINT ( 'NONE',  ( 24.05283483419999868, -94.34469964500000572, -8.234368469370000554 ) ) ;
#17043=ORIENTED_EDGE ( 'NONE', *, *, #28760, .T. ) ;
#17044=ADVANCED_FACE ( 'NONE', ( #5590 ), #1514, .F. ) ;
#17045=CARTESIAN_POINT ( 'NONE',  ( 27.36513940969999936, -92.50000000000000000, 13.03937715500000039 ) ) ;
#17050=B_SPLINE_SURFACE_WITH_KNOTS ( 'NONE', 5, 5, ( 
 ( #12566, #28305, #12706, #19565, #23945, #24234, #3982, #6015, #19842 ),
 ( #1806, #28594, #15031, #4267, #26419, #14896, #28725, #21620, #8763 ),
 ( #5880, #21902, #25856, #23805, #8338, #10648, #28453, #8487, #17388 ),
 ( #26861, #24519, #4706, #4994, #514, #6606, #13434, #11077, #7050 ),
 ( #19994, #13586, #22191, #20292, #67, #9206, #22494, #8913, #9361 ),
 ( #22338, #17822, #11390, #2386, #2536, #13739, #13881, #22639, #26716 ),
 ( #18262, #22786, #2824, #11242, #11686, #20597, #15619, #657, #11977 ),
 ( #12261, #5434, #27857, #7906, #5575, #955, #12116, #16786, #9932 ),
 ( #23353, #18846, #25682, #14591, #808, #27300, #7495, #7338, #2977 ),
 ( #11836, #9649, #16204, #27450, #25269, #23625, #28005, #8041, #14860 ),
 ( #16929, #3944, #3665, #12808, #12668, #12527, #24043, #23907, #5978 ),
 ( #25821, #23764, #1498, #21580, #6408, #5844, #26092, #6121, #21717 ) ),
 .UNSPECIFIED., .F., .F., .F.,
 ( 6, 3, 3, 6 ),
 ( 6, 3, 6 ),
 ( 3.852920539479999906, 4.834764074430000669, 6.134713715060000183, 8.383984506240000911 ),
 ( 0.000000000000000000, 0.2500000000000000000, 0.5000000000000000000 ),
 .UNSPECIFIED. ) ;
#17051=VERTEX_POINT ( 'NONE', #23368 ) ;
#17052=B_SPLINE_CURVE_WITH_KNOTS ( 'NONE', 5,
 ( #16691, #28326, #25593, #7951, #5759, #1270 ),
 .UNSPECIFIED., .F., .F.,
 ( 6, 6 ),
 ( 0.000000000000000000, 1.000000000000000000 ),
 .UNSPECIFIED. ) ;
#17056=CARTESIAN_POINT ( 'NONE',  ( -20.70743651480000125, -111.0000000000000000, -4.683547831859999455 ) ) ;
#17058=CARTESIAN_POINT ( 'NONE',  ( 12.05761442979999920, -96.99283697629999779, 17.05217550289999906 ) ) ;
#17061=CARTESIAN_POINT ( 'NONE',  ( 1.924356917819999957, -93.14733690340000294, 27.32343874049999854 ) ) ;
#17068=CARTESIAN_POINT ( 'NONE',  ( -27.08130798099999836, -92.87437365140000622, -4.263279399680000026 ) ) ;
#17076=EDGE_CURVE ( 'NONE', #21210, #11981, #26774, .T. ) ;
#17078=CARTESIAN_POINT ( 'NONE',  ( 0.08847858422719999394, -101.5964542560000012, -16.04011128580000189 ) ) ;
#17081=CARTESIAN_POINT ( 'NONE',  ( 6.153546133999999945, -93.00000450890000536, 28.82528558229999760 ) ) ;
#17085=CARTESIAN_POINT ( 'NONE',  ( 6.664266769160000159, -101.1191090859999946, 14.88020880370000043 ) ) ;
#17086=CARTESIAN_POINT ( 'NONE',  ( -15.68499803141670057, -92.57495907656227985, -24.03044298549235691 ) ) ;
#17087=AXIS2_PLACEMENT_3D ( 'NONE', #22656, #1240, #23927 ) ;
#17088=CARTESIAN_POINT ( 'NONE',  ( -7.340076801780219817, -98.99956641980976713, 17.08769940940410237 ) ) ;
#17091=CARTESIAN_POINT ( 'NONE',  ( 6.623136366559999821, -92.50000000000000000, -29.58057261400000115 ) ) ;
#17094=CARTESIAN_POINT ( 'NONE',  ( 8.553834212409999083, -94.06807348059999185, -23.81750769579999982 ) ) ;
#17100=ORIENTED_EDGE ( 'NONE', *, *, #14978, .F. ) ;
#17106=CARTESIAN_POINT ( 'NONE',  ( 12.59683198944025229, -94.65677004896708979, -20.59035092372582554 ) ) ;
#17110=CARTESIAN_POINT ( 'NONE',  ( 16.40944971170530309, -94.60237058323863835, 17.21713387757399971 ) ) ;
#17115=CARTESIAN_POINT ( 'NONE',  ( 24.10654937457443125, -94.27895761462396251, -8.513691059147493689 ) ) ;
#17120=ORIENTED_EDGE ( 'NONE', *, *, #23443, .F. ) ;
#17122=ORIENTED_EDGE ( 'NONE', *, *, #15642, .T. ) ;
#17126=CARTESIAN_POINT ( 'NONE',  ( -29.15742847839999996, -92.53610956480000027, 4.773646594879999761 ) ) ;
#17127=CARTESIAN_POINT ( 'NONE',  ( -0.6875333948397619466, -101.1962283502373623, -15.25188306018329243 ) ) ;
#17128=ORIENTED_EDGE ( 'NONE', *, *, #17487, .T. ) ;
#17131=ORIENTED_EDGE ( 'NONE', *, *, #11744, .F. ) ;
#17134=AXIS2_PLACEMENT_3D ( 'NONE', #9444, #12059, #7136 ) ;
#17137=AXIS2_PLACEMENT_3D ( 'NONE', #21541, #1597, #28100 ) ;
#17139=CARTESIAN_POINT ( 'NONE',  ( -15.61807470970000011, -101.5138947819999942, 3.547044975749999995 ) ) ;
#17142=ORIENTED_EDGE ( 'NONE', *, *, #9550, .F. ) ;
#17143=( GEOMETRIC_REPRESENTATION_CONTEXT ( 3 ) GLOBAL_UNCERTAINTY_ASSIGNED_CONTEXT ( ( #3351 ) ) GLOBAL_UNIT_ASSIGNED_CONTEXT ( ( #10188, #19512, #21429 ) ) REPRESENTATION_CONTEXT ( 'NONE', 'WORKASPACE' ) );
#17145=CARTESIAN_POINT ( 'NONE',  ( -12.55040281159999971, -101.4254868729999970, -9.874220623960001220 ) ) ;
#17147=CARTESIAN_POINT ( 'NONE',  ( -7.556190961256522343, -101.1451610289769718, 14.54526516815933590 ) ) ;
#17148=EDGE_LOOP ( 'NONE', ( #5778, #22184, #2160, #27030 ) ) ;
#17149=DIRECTION ( 'NONE',  ( 1.000000000000000000, 0.000000000000000000, 0.000000000000000000 ) ) ;
#17152=VERTEX_POINT ( 'NONE', #22032 ) ;
#17155=CIRCLE ( 'NONE', #19477, 30.50000000000000000 ) ;
#17156=CARTESIAN_POINT ( 'NONE',  ( 6.785573360597900283, -100.4872618017465840, 15.49051439867366398 ) ) ;
#17158=ORIENTED_EDGE ( 'NONE', *, *, #26589, .T. ) ;
#17165=CARTESIAN_POINT ( 'NONE',  ( 12.86597616020000068, -100.8023006570000035, -9.130347141119999677 ) ) ;
#17167=B_SPLINE_CURVE_WITH_KNOTS ( 'NONE', 5,
 ( #24989, #11108, #13765, #27182, #542, #22664 ),
 .UNSPECIFIED., .F., .F.,
 ( 6, 6 ),
 ( 0.000000000000000000, 1.000000000000000000 ),
 .UNSPECIFIED. ) ;
#17171=CARTESIAN_POINT ( 'NONE',  ( -23.48382783139999930, -92.84292833370000153, -19.25540828950000360 ) ) ;
#17173=ORIENTED_EDGE ( 'NONE', *, *, #6517, .T. ) ;
#17175=CARTESIAN_POINT ( 'NONE',  ( -13.15906405200000151, -99.57787118749999422, -11.31977148680000056 ) ) ;
#17177=CARTESIAN_POINT ( 'NONE',  ( 12.85509542230000157, -100.8455998110000138, -9.598705754820000990 ) ) ;
#17178=CARTESIAN_POINT ( 'NONE',  ( -18.69985100839999959, -93.00000000000000000, 22.78328762010000119 ) ) ;
#17179=CARTESIAN_POINT ( 'NONE',  ( 23.50847989309999875, -93.85715850779999414, -8.212858164749999190 ) ) ;
#17194=AXIS2_PLACEMENT_3D ( 'NONE', #5076, #22867, #3062 ) ;
#17197=VERTEX_POINT ( 'NONE', #26263 ) ;
#17201=EDGE_LOOP ( 'NONE', ( #21316, #20787, #6993, #18899 ) ) ;
#17202=CARTESIAN_POINT ( 'NONE',  ( -12.73050580650000008, -101.1716782170000073, -9.245982730369998848 ) ) ;
#17203=EDGE_CURVE ( 'NONE', #22807, #22871, #19313, .T. ) ;
#17205=CARTESIAN_POINT ( 'NONE',  ( -2.864434201389999934, -99.61931799660000308, -17.24218458769999884 ) ) ;
#17209=CARTESIAN_POINT ( 'NONE',  ( 12.45133382055230165, -101.6484611539999747, -10.04845847643241541 ) ) ;
#17212=CARTESIAN_POINT ( 'NONE',  ( 6.944463756510000252, -99.57787269160000676, 15.90826982280000124 ) ) ;
#17225=CARTESIAN_POINT ( 'NONE',  ( 15.07019258820000118, -101.1848541600000004, 2.542738038029999981 ) ) ;
#17230=CARTESIAN_POINT ( 'NONE',  ( 6.933748734719999973, -99.99711545080000974, 15.71060619540000047 ) ) ;
#17231=CARTESIAN_POINT ( 'NONE',  ( -15.77460418939101849, -92.56934535156428012, -24.02693241158716120 ) ) ;
#17234=CARTESIAN_POINT ( 'NONE',  ( 4.261015134245454306, -92.86276748796085201, -30.20116777978838840 ) ) ;
#17235=CARTESIAN_POINT ( 'NONE',  ( -3.215500929169999633, -94.59276292389999696, 23.57860676330000160 ) ) ;
#17236=ORIENTED_EDGE ( 'NONE', *, *, #1428, .F. ) ;
#17238=CARTESIAN_POINT ( 'NONE',  ( 7.993247198980000690, -93.67384740779999674, -24.35792768219999971 ) ) ;
#17240=EDGE_CURVE ( 'NONE', #5855, #9315, #20027, .T. ) ;
#17241=CIRCLE ( 'NONE', #18188, 7.000000000000000000 ) ;
#17243=CARTESIAN_POINT ( 'NONE',  ( 6.708131455446116220, -101.3586211801433166, 14.77255361321039118 ) ) ;
#17244=DIRECTION ( 'NONE',  ( 0.4794255386042040601, 0.000000000000000000, 0.8775825618903722036 ) ) ;
#17247=CARTESIAN_POINT ( 'NONE',  ( -12.52732263940944435, -101.0610180771033413, -10.67209290993696236 ) ) ;
#17249=CARTESIAN_POINT ( 'NONE',  ( 25.70121108570000246, -93.05538536790000137, -5.710191390220000329 ) ) ;
#17250=CARTESIAN_POINT ( 'NONE',  ( -0.8149835146670000308, -101.1716782080000030, -15.71308785760000148 ) ) ;
#17254=CARTESIAN_POINT ( 'NONE',  ( 16.02651611377384810, -94.78494200512166401, 17.25365316566084672 ) ) ;
#17256=CARTESIAN_POINT ( 'NONE',  ( 26.40471317329472711, -92.73901256243104285, 13.20493500560145073 ) ) ;
#17258=DIRECTION ( 'NONE',  ( 0.000000000000000000, -1.000000000000000000, 0.000000000000000000 ) ) ;
#17259=CARTESIAN_POINT ( 'NONE',  ( 24.43683151600445314, -93.86130746219269838, -9.930393139660877111 ) ) ;
#17265=DIRECTION ( 'NONE',  ( 0.9988549560444618391, 0.000000000000000000, 0.04784116204082212997 ) ) ;
#17273=CARTESIAN_POINT ( 'NONE',  ( -25.18134011720000132, -94.15497152599999708, -3.050188418449999883 ) ) ;
#17275=ADVANCED_FACE ( 'NONE', ( #22472 ), #25492, .F. ) ;
#17279=CARTESIAN_POINT ( 'NONE',  ( -12.29363612059999866, -101.2530993000000024, -8.928690578620001261 ) ) ;
#17284=VECTOR ( 'NONE', #4368, 1000.000000000000000 ) ;
#17289=B_SPLINE_SURFACE_WITH_KNOTS ( 'NONE', 5, 5, ( 
 ( #26600, #6643, #15505, #4014, #20038, #24414, #21788, #1844, #9684 ),
 ( #20186, #9548, #18596, #14223, #22534, #4747, #13771, #26901, #13921 ),
 ( #22822, #22673, #13626, #5185, #24997, #15952, #2576, #2865, #11425 ),
 ( #20326, #2717, #399, #9246, #261, #27192, #9100, #18004, #11281 ),
 ( #15803, #696, #11725, #24711, #4892, #18148, #11571, #27045, #20481 ),
 ( #549, #9395, #16394, #7232, #18302, #16097, #20640, #7088, #24857 ) ),
 .UNSPECIFIED., .F., .F., .F.,
 ( 6, 6 ),
 ( 6, 3, 6 ),
 ( 10.27983419550000121, 28.98451109730000042 ),
 ( 0.000000000000000000, 0.2500000000000000000, 0.5000000000000000000 ),
 .UNSPECIFIED. ) ;
#17293=CARTESIAN_POINT ( 'NONE',  ( -12.06953548060000081, -101.1411470200000053, -9.548139877839998846 ) ) ;
#17294=CARTESIAN_POINT ( 'NONE',  ( -7.522398661245357054, -101.1884902308600118, 14.52463055899669087 ) ) ;
#17295=EDGE_LOOP ( 'NONE', ( #12594, #382, #23362, #28201 ) ) ;
#17308=VERTEX_POINT ( 'NONE', #1211 ) ;
#17310=DIRECTION ( 'NONE',  ( 0.000000000000000000, -1.000000000000000000, 0.000000000000000000 ) ) ;
#17311=CARTESIAN_POINT ( 'NONE',  ( 1.631276547419999945, -94.59276292389999696, 23.74086995720000104 ) ) ;
#17316=CARTESIAN_POINT ( 'NONE',  ( -29.47186832370000076, -93.00000450890000536, -0.4149655844399999793 ) ) ;
#17317=CARTESIAN_POINT ( 'NONE',  ( -18.81974815339999907, -92.68289710869998999, -20.86662628930000096 ) ) ;
#17321=CARTESIAN_POINT ( 'NONE',  ( -20.51325115670000443, -95.66919271829999616, -9.269412113539999609 ) ) ;
#17322=CARTESIAN_POINT ( 'NONE',  ( 12.01586610120000032, -101.1700440390000040, -9.474730661679998889 ) ) ;
#17331=CARTESIAN_POINT ( 'NONE',  ( -2.664535259099999805E-15, -101.6484611540000031, 1.776356839399999804E-15 ) ) ;
#17332=CARTESIAN_POINT ( 'NONE',  ( 21.67693832783029961, -96.57210917632126268, 0.1672311650303546227 ) ) ;
#17335=CARTESIAN_POINT ( 'NONE',  ( -0.2442174124554105097, -92.66191076887825773, -30.49908852203764198 ) ) ;
#17342=CARTESIAN_POINT ( 'NONE',  ( 21.26288536570000076, -97.23151480340000319, -2.165621899160000030 ) ) ;
#17343=VERTEX_POINT ( 'NONE', #17045 ) ;
#17345=DIRECTION ( 'NONE',  ( 1.000000000000000000, 0.000000000000000000, 0.000000000000000000 ) ) ;
#17346=ORIENTED_EDGE ( 'NONE', *, *, #11744, .T. ) ;
#17347=CARTESIAN_POINT ( 'NONE',  ( -13.05440433799999944, -101.3957169669999985, -9.227549938650001948 ) ) ;
#17350=CARTESIAN_POINT ( 'NONE',  ( -0.1520325283909999825, -93.05538537019999978, 26.32746518160000093 ) ) ;
#17352=CARTESIAN_POINT ( 'NONE',  ( -30.37538215883989068, -92.92035259800012170, 2.768038011894732087 ) ) ;
#17357=CARTESIAN_POINT ( 'NONE',  ( 13.06668678909421111, -101.2021794473205603, -9.821573571294250016 ) ) ;
#17364=FACE_OUTER_BOUND ( 'NONE', #16263, .T. ) ;
#17365=CARTESIAN_POINT ( 'NONE',  ( -20.54393874204836123, -94.23729456146304528, 12.90813503536128692 ) ) ;
#17369=CARTESIAN_POINT ( 'NONE',  ( 1.057205864080000168, -100.1340845430000002, -16.60558664359999881 ) ) ;
#17377=CARTESIAN_POINT ( 'NONE',  ( 6.475617225940000665, -101.0151300849999814, 14.23442573650000043 ) ) ;
#17378=CARTESIAN_POINT ( 'NONE',  ( -16.36884634468729516, -92.53775804172235553, -23.99411788281411972 ) ) ;
#17382=CARTESIAN_POINT ( 'NONE',  ( 4.396272035099083375, -92.82529299094557018, -30.18149772317508805 ) ) ;
#17386=CARTESIAN_POINT ( 'NONE',  ( 3.408291041020000467, -92.96321827540000982, -28.95142855790000169 ) ) ;
#17387=CARTESIAN_POINT ( 'NONE',  ( 6.788846616428737768, -101.5026031440148842, 14.61257718564415242 ) ) ;
#17388=CARTESIAN_POINT ( 'NONE',  ( -6.708539788989999586, -101.2358105800000061, 13.65871639999999942 ) ) ;
#17391=CARTESIAN_POINT ( 'NONE',  ( -12.77330844608892590, -100.5798851005997676, -10.97038188722230956 ) ) ;
#17394=CARTESIAN_POINT ( 'NONE',  ( 24.71295097499999827, -93.67869433800001389, -3.805954965999999828 ) ) ;
#17396=CIRCLE ( 'NONE', #5311, 20.64285714289999873 ) ;
#17405=CARTESIAN_POINT ( 'NONE',  ( 29.52540673129999860, -93.00000000000000000, 7.168153169610000930 ) ) ;
#17406=EDGE_CURVE ( 'NONE', #15088, #24436, #11326, .T. ) ;
#17409=FACE_OUTER_BOUND ( 'NONE', #23825, .T. ) ;
#17410=CARTESIAN_POINT ( 'NONE',  ( -24.15516222759999820, -94.98812477599999227, -4.102682929219999330 ) ) ;
#17412=CARTESIAN_POINT ( 'NONE',  ( 23.69519146889223649, -94.79128788265268213, -7.184658344615285408 ) ) ;
#17415=EDGE_CURVE ( 'NONE', #10810, #4274, #3891, .T. ) ;
#17421=LINE ( 'NONE', #1983, #15778 ) ;
#17426=DIRECTION ( 'NONE',  ( 0.05900121837168382372, 0.000000000000000000, 0.9982579106777251798 ) ) ;
#17427=ORIENTED_EDGE ( 'NONE', *, *, #20155, .F. ) ;
#17434=ADVANCED_FACE ( 'NONE', ( #16488 ), #27718, .T. ) ;
#17435=CARTESIAN_POINT ( 'NONE',  ( -14.89662347129999986, -101.1848541720000014, 3.414158506610000199 ) ) ;
#17437=CARTESIAN_POINT ( 'NONE',  ( -13.16239993169999956, -100.8816835080000089, -8.729908192910000864 ) ) ;
#17438=VERTEX_POINT ( 'NONE', #25520 ) ;
#17441=CARTESIAN_POINT ( 'NONE',  ( -11.80853318720000011, -100.8815367389999977, -10.30796059140000054 ) ) ;
#17443=CARTESIAN_POINT ( 'NONE',  ( -7.762847924256437437, -100.8061861225939708, 14.73824615606121746 ) ) ;
#17445=EDGE_CURVE ( 'NONE', #2579, #5717, #12373, .T. ) ;
#17446=B_SPLINE_CURVE_WITH_KNOTS ( 'NONE', 3,
 ( #23592, #16754, #12363, #3636, #1064, #1466 ),
 .UNSPECIFIED., .F., .F.,
 ( 4, 2, 4 ),
 ( 0.000000000000000000, 0.5000000000000000000, 1.000000000000000000 ),
 .UNSPECIFIED. ) ;
#17447=DIRECTION ( 'NONE',  ( -0.000000000000000000, 1.000000000000000000, 0.000000000000000000 ) ) ;
#17449=CARTESIAN_POINT ( 'NONE',  ( -10.63276174549836917, -93.28923452009620121, -23.66442649163524337 ) ) ;
#17452=CYLINDRICAL_SURFACE ( 'NONE', #21306, 5.999999999999999112 ) ;
#17453=B_SPLINE_CURVE_WITH_KNOTS ( 'NONE', 3,
 ( #3771, #8408, #10030, #21684, #3908, #1195, #23315, #12491, #12774, #1462, #27827, #1731, #10572, #10303, #28232, #23589, #19487 ),
 .UNSPECIFIED., .F., .F.,
 ( 4, 2, 2, 1, 1, 1, 1, 1, 2, 2, 4 ),
 ( 0.000000000000000000, 0.2500000000000092149, 0.3750000000000130451, 0.4375000000000158762, 0.4687500000000175970, 0.4843750000000193179, 0.4921875000000209832, 0.4960937500000218159, 0.4980468750000214273, 0.5000000000000209832, 1.000000000000000000 ),
 .UNSPECIFIED. ) ;
#17455=CARTESIAN_POINT ( 'NONE',  ( -17.16748885897166943, -93.45279863366459949, -21.41968775130273528 ) ) ;
#17456=ORIENTED_EDGE ( 'NONE', *, *, #26258, .F. ) ;
#17457=CARTESIAN_POINT ( 'NONE',  ( 24.24773784319999947, -93.39359559929999932, 12.30290705160000009 ) ) ;
#17464=CARTESIAN_POINT ( 'NONE',  ( -20.32909851670000378, -92.54030566109999256, -20.27308962609999909 ) ) ;
#17467=CARTESIAN_POINT ( 'NONE',  ( -6.126542658125574192, -101.6174239712916432, 14.80565200955684801 ) ) ;
#17469=CARTESIAN_POINT ( 'NONE',  ( 13.64192749750000111, -100.1340845430000002, -9.526857098169999816 ) ) ;
#17471=CARTESIAN_POINT ( 'NONE',  ( -5.731166642400647326, -98.21052819054347083, -19.47007456258096170 ) ) ;
#17472=CLOSED_SHELL ( 'NONE', ( #14577, #7057, #1804, #1664, #16121, #3881, #26679, #17741, #9960, #16685, #28635, #28399, #7219, #14666, #5402, #391, #1784, #24098, #24615, #2912, #15071, #8723, #6885, #12925, #9415, #11542, #10461, #27027, #6554, #28374, #22290, #4310, #24544, #12203, #15132, #20648, #28064, #22585, #16641, #20723, #1589, #8332, #6479, #27724, #571, #10206, #28095, #1216, #21008, #9465, #18103, #28532, #7362, #11917, #1693, #8939, #10218, #5603, #23185, #16451, #5886, #13340, #20191, #21356, #8269, #12825, #9339, #1076, #4983, #22818, #26884, #24617, #17275, #5215, #25303, #19144, #9241, #21615, #2123, #21454, #3157, #8433, #23953, #25427, #3149, #5699, #12552, #27686, #16218, #27089, #12359, #772, #15226, #8347, #24970, #23612, #16784, #14913, #6143, #17693, #14164, #25854, #11883, #4542, #2452, #17522, #7788, #11708, #24651, #1564, #22009, #3613, #17812, #17044, #26723, #22483, #16499, #21642, #3125, #26079, #24137, #13308, #27758, #22168, #12107, #8233, #28334, #7846, #25231, #7998, #11463, #23792, #9231, #20336, #20618, #23821, #13535, #6302, #26748, #27808, #24507, #14612, #28126, #6828, #10751, #18041, #4851, #17434, #10498, #2420, #11378, #15809, #7675, #12797, #26223, #25475 ) ) ;
#17477=DIRECTION ( 'NONE',  ( 0.000000000000000000, 1.000000000000000000, 0.000000000000000000 ) ) ;
#17480=CARTESIAN_POINT ( 'NONE',  ( -23.91155634505533811, -92.72722989463423460, -18.93376855828962135 ) ) ;
#17485=DIRECTION ( 'NONE',  ( 0.4794255386042041156, 0.000000000000000000, 0.8775825618903722036 ) ) ;
#17486=ORIENTED_EDGE ( 'NONE', *, *, #12896, .T. ) ;
#17487=EDGE_CURVE ( 'NONE', #22409, #24426, #15997, .T. ) ;
#17488=CARTESIAN_POINT ( 'NONE',  ( 20.68906639099999722, -96.97547176279999803, -2.416818656099999796 ) ) ;
#17494=CARTESIAN_POINT ( 'NONE',  ( -15.09559145619999931, -92.94652576229999852, -23.64540529880000008 ) ) ;
#17496=CARTESIAN_POINT ( 'NONE',  ( -6.552399679369999674, -97.31350077540000143, -20.03651016279999908 ) ) ;
#17498=FACE_OUTER_BOUND ( 'NONE', #25244, .T. ) ;
#17503=CARTESIAN_POINT ( 'NONE',  ( 13.27592836724310743, -100.9570234915505154, -9.862972498476620942 ) ) ;
#17507=VERTEX_POINT ( 'NONE', #13084 ) ;
#17509=CARTESIAN_POINT ( 'NONE',  ( -14.11074263820000141, -92.49626986490000036, 25.91332334039999807 ) ) ;
#17513=CARTESIAN_POINT ( 'NONE',  ( 0.8847930891630000350, -99.97545561319999763, -16.87691942780000076 ) ) ;
#17518=VERTEX_POINT ( 'NONE', #13231 ) ;
#17520=CARTESIAN_POINT ( 'NONE',  ( -16.54020593362537639, -92.53069453552505763, -23.98110413831777521 ) ) ;
#17522=ADVANCED_FACE ( 'NONE', ( #12927 ), #28391, .F. ) ;
#17523=CARTESIAN_POINT ( 'NONE',  ( 27.89467015572686748, -92.52498922770504919, 12.33462672781183223 ) ) ;
#17524=CARTESIAN_POINT ( 'NONE',  ( 5.818223828271644749, -92.52498922770502077, -29.94000519531349624 ) ) ;
#17525=CARTESIAN_POINT ( 'NONE',  ( -5.605636395229999458, -96.73974214309998843, 20.49386430090000033 ) ) ;
#17527=CARTESIAN_POINT ( 'NONE',  ( 7.854958299419999790, -93.60790942689999383, -24.22480680409999820 ) ) ;
#17529=CARTESIAN_POINT ( 'NONE',  ( 6.838545786690161776, -101.5526869446500484, 14.54657801930438410 ) ) ;
#17530=FACE_OUTER_BOUND ( 'NONE', #1101, .T. ) ;
#17531=ORIENTED_EDGE ( 'NONE', *, *, #21224, .F. ) ;
#17532=CARTESIAN_POINT ( 'NONE',  ( 0.000000000000000000, -107.5000000000000000, 0.000000000000000000 ) ) ;
#17533=CARTESIAN_POINT ( 'NONE',  ( -12.48657657042820013, -101.1884902308936063, -10.56583077869183640 ) ) ;
#17539=CARTESIAN_POINT ( 'NONE',  ( 12.32081986847368071, -94.36683344927988060, -21.27645860062538574 ) ) ;
#17542=CARTESIAN_POINT ( 'NONE',  ( -20.95552429882483736, -92.86276748915979340, -22.16151589128406840 ) ) ;
#17543=ORIENTED_EDGE ( 'NONE', *, *, #19763, .F. ) ;
#17544=DIRECTION ( 'NONE',  ( 1.000000000000000000, 0.000000000000000000, 0.000000000000000000 ) ) ;
#17546=CARTESIAN_POINT ( 'NONE',  ( 0.000000000000000000, -101.2530993010000060, 0.000000000000000000 ) ) ;
#17547=CARTESIAN_POINT ( 'NONE',  ( -30.34790777679999962, -91.50000000000000000, 3.042119914239999723 ) ) ;
#17548=CARTESIAN_POINT ( 'NONE',  ( 13.71624454005582905, -100.2392017794815189, -10.22880014236059054 ) ) ;
#17557=CARTESIAN_POINT ( 'NONE',  ( -24.42422992060000198, -94.22485739650001335, -3.548043453489999610 ) ) ;
#17562=CARTESIAN_POINT ( 'NONE',  ( 15.78891807579999984, -101.1191090859999946, 4.067324870920000279 ) ) ;
#17564=CARTESIAN_POINT ( 'NONE',  ( -20.93804484360220641, -95.75133630109712612, -8.863926826236266265 ) ) ;
#17567=EDGE_LOOP ( 'NONE', ( #869, #5399, #12874, #20607 ) ) ;
#17575=CARTESIAN_POINT ( 'NONE',  ( -15.62855498089999884, -101.6223710729999965, 3.522773483530000416 ) ) ;
#17581=CARTESIAN_POINT ( 'NONE',  ( -1.826285548319301455, -96.92941681384529318, 21.94491567526166520 ) ) ;
#17582=CARTESIAN_POINT ( 'NONE',  ( -11.79122448039999860, -101.0403179300000005, -10.01466385380000013 ) ) ;
#17591=B_SPLINE_SURFACE_WITH_KNOTS ( 'NONE', 4, 5, ( 
 ( #23523, #7669, #18730, #3144, #27626, #14213, #16534, #27759, #25566 ),
 ( #20917, #1250, #19006, #21060, #4068, #23104, #1119, #27476, #25296 ),
 ( #12002, #21329, #18874, #25710, #7795, #14621, #9957, #14483, #28032 ),
 ( #980, #10229, #1387, #3559, #16817, #16668, #12414, #21849, #15122 ),
 ( #10743, #27886, #14345, #12146, #19143, #24031, #9822, #5600, #5739 ) ),
 .UNSPECIFIED., .F., .F., .F.,
 ( 5, 5 ),
 ( 6, 3, 6 ),
 ( 27.16653081609999987, 27.95952390849999958 ),
 ( 0.000000000000000000, 0.2500000000000000000, 0.5000000000000000000 ),
 .UNSPECIFIED. ) ;
#17594=CARTESIAN_POINT ( 'NONE',  ( 0.000000000000000000, -108.5000000000000000, 0.000000000000000000 ) ) ;
#17599=CARTESIAN_POINT ( 'NONE',  ( -13.66444693457865078, -94.27895761266917418, -21.60767336590412668 ) ) ;
#17601=CARTESIAN_POINT ( 'NONE',  ( 19.98296174609999909, -94.98812477599999227, 14.17692170709999822 ) ) ;
#17603=ORIENTED_EDGE ( 'NONE', *, *, #17837, .F. ) ;
#17604=CARTESIAN_POINT ( 'NONE',  ( 0.000000000000000000, -92.50000000000000000, 0.000000000000000000 ) ) ;
#17606=EDGE_CURVE ( 'NONE', #2738, #19454, #27188, .T. ) ;
#17607=CARTESIAN_POINT ( 'NONE',  ( 12.41938065250000101, -101.4254868729999970, -10.03851721480000059 ) ) ;
#17612=CARTESIAN_POINT ( 'NONE',  ( 13.35715127229999943, -100.8746138070000029, -9.861395958219999258 ) ) ;
#17614=CARTESIAN_POINT ( 'NONE',  ( -11.85289063449999958, -94.98812477599999227, -21.44324726029999795 ) ) ;
#17615=DIRECTION ( 'NONE',  ( 0.000000000000000000, -1.000000000000000000, 0.000000000000000000 ) ) ;
#17618=ORIENTED_EDGE ( 'NONE', *, *, #23651, .T. ) ;
#17620=DIRECTION ( 'NONE',  ( -0.000000000000000000, 1.000000000000000000, 0.000000000000000000 ) ) ;
#17623=CARTESIAN_POINT ( 'NONE',  ( -23.77551070246358478, -92.93978723897004102, -19.10432693837231000 ) ) ;
#17625=CARTESIAN_POINT ( 'NONE',  ( -0.8980256170553421180, -92.52048598157983861, -30.48678096363293477 ) ) ;
#17632=ORIENTED_EDGE ( 'NONE', *, *, #10842, .F. ) ;
#17634=CARTESIAN_POINT ( 'NONE',  ( 23.52741021270000132, -94.89420189139998740, -6.742682298520000117 ) ) ;
#17635=AXIS2_PLACEMENT_3D ( 'NONE', #16713, #10410, #14791 ) ;
#17640=CARTESIAN_POINT ( 'NONE',  ( 16.03761573839999954, -101.2306315440000049, 2.381275335019999773 ) ) ;
#17641=AXIS2_PLACEMENT_3D ( 'NONE', #8272, #11006, #10443 ) ;
#17642=EDGE_CURVE ( 'NONE', #22108, #7500, #22061, .T. ) ;
#17645=CARTESIAN_POINT ( 'NONE',  ( 0.000000000000000000, -111.0000000000000000, 0.000000000000000000 ) ) ;
#17647=CARTESIAN_POINT ( 'NONE',  ( 0.04171660379150000236, -111.0000000000000000, 21.23044528579999835 ) ) ;
#17654=CARTESIAN_POINT ( 'NONE',  ( -13.11455779531268284, -92.71346081468166744, 27.53649186493240464 ) ) ;
#17655=ORIENTED_EDGE ( 'NONE', *, *, #15676, .T. ) ;
#17657=CARTESIAN_POINT ( 'NONE',  ( -14.45392997149999914, -92.99999875040001029, 26.19394095939999900 ) ) ;
#17658=ORIENTED_EDGE ( 'NONE', *, *, #11854, .F. ) ;
#17662=CARTESIAN_POINT ( 'NONE',  ( 0.7145790383449999172, -100.7707614970000094, -15.83861793500000026 ) ) ;
#17664=CARTESIAN_POINT ( 'NONE',  ( 15.74335372269999844, -101.5369810359999860, 2.854262349850000380 ) ) ;
#17668=TOROIDAL_SURFACE ( 'NONE', #13468, 21.14285714289999873, 0.5000000000000000000 ) ;
#17671=EDGE_LOOP ( 'NONE', ( #5544, #26314, #8297, #16563, #14519, #11400 ) ) ;
#17673=CARTESIAN_POINT ( 'NONE',  ( 27.97334130874722291, -92.55017404142810733, 12.15492542743048787 ) ) ;
#17675=CARTESIAN_POINT ( 'NONE',  ( 24.60124523610000224, -92.58502644590001296, 14.64067842810000108 ) ) ;
#17676=CARTESIAN_POINT ( 'NONE',  ( 6.865158367083817659, -101.5740747342471337, 14.51578316883484199 ) ) ;
#17679=CARTESIAN_POINT ( 'NONE',  ( -12.88209131945397168, -100.4211561362087792, -11.03803975983561791 ) ) ;
#17680=ORIENTED_EDGE ( 'NONE', *, *, #18844, .T. ) ;
#17685=CARTESIAN_POINT ( 'NONE',  ( 8.660862689520000046, -98.53838189920000445, 16.57756802869999646 ) ) ;
#17688=CARTESIAN_POINT ( 'NONE',  ( -15.38256540239999914, -101.5026274779999937, 4.483298071290000131 ) ) ;
#17693=ADVANCED_FACE ( 'NONE', ( #7281 ), #26233, .T. ) ;
#17694=CARTESIAN_POINT ( 'NONE',  ( 26.58922696730754254, -92.50000267096380924, 13.46049426897001489 ) ) ;
#17697=DIRECTION ( 'NONE',  ( -0.9734759478401043831, 0.000000000000000000, -0.2287893768880245871 ) ) ;
#17698=CARTESIAN_POINT ( 'NONE',  ( 22.48686483693199278, -94.01603309715282819, 13.16869411391845546 ) ) ;
#17699=ORIENTED_EDGE ( 'NONE', *, *, #7898, .F. ) ;
#17702=EDGE_CURVE ( 'NONE', #23314, #20359, #17396, .T. ) ;
#17706=B_SPLINE_CURVE_WITH_KNOTS ( 'NONE', 3,
 ( #23700, #6209, #28078, #28494, #1708, #8532 ),
 .UNSPECIFIED., .F., .F.,
 ( 4, 2, 4 ),
 ( 0.000000000000000000, 0.5000000000000000000, 1.000000000000000000 ),
 .UNSPECIFIED. ) ;
#17709=CARTESIAN_POINT ( 'NONE',  ( -24.67624118369999664, -94.54647010790000650, -3.610732365350000084 ) ) ;
#17714=CARTESIAN_POINT ( 'NONE',  ( 16.00391739089999987, -100.1785804069999983, 4.588803089980000749 ) ) ;
#17717=LINE ( 'NONE', #28345, #24303 ) ;
#17719=CARTESIAN_POINT ( 'NONE',  ( 7.560610606073200124, -92.50638022835023833, 29.54840156989449440 ) ) ;
#17725=CARTESIAN_POINT ( 'NONE',  ( 24.37463189540000030, -92.54807930239999791, -15.31860879340000103 ) ) ;
#17728=LINE ( 'NONE', #24423, #23895 ) ;
#17730=CARTESIAN_POINT ( 'NONE',  ( -17.04099446512953975, -97.63928043689861624, 10.20266565317231411 ) ) ;
#17732=CARTESIAN_POINT ( 'NONE',  ( 11.70455088819999823, -93.00000000000000000, 8.942783294160001617 ) ) ;
#17735=CARTESIAN_POINT ( 'NONE',  ( -13.18018122016701277, -99.62767017969132155, -11.26298828346031300 ) ) ;
#17736=ORIENTED_EDGE ( 'NONE', *, *, #20752, .F. ) ;
#17741=ADVANCED_FACE ( 'NONE', ( #20692 ), #4762, .F. ) ;
#17743=CARTESIAN_POINT ( 'NONE',  ( -5.122964312370000606, -100.0012764450000020, 17.27741718500000090 ) ) ;
#17745=CARTESIAN_POINT ( 'NONE',  ( -17.63662161709793708, -94.54718950358140717, 16.06392408143854666 ) ) ;
#17746=CIRCLE ( 'NONE', #6101, 16.00000000000000000 ) ;
#17748=CARTESIAN_POINT ( 'NONE',  ( -14.43573106120380523, -94.04667188284982160, -21.62179604614098949 ) ) ;
#17752=CARTESIAN_POINT ( 'NONE',  ( -15.07208659220000158, -101.6484611540000031, 3.616933197699999880 ) ) ;
#17757=CARTESIAN_POINT ( 'NONE',  ( -18.92594650439999882, -92.98926436760000058, -21.15881086809999800 ) ) ;
#17758=CARTESIAN_POINT ( 'NONE',  ( 3.166345171159999694, -92.50000000000000000, -25.30265318609999881 ) ) ;
#17760=CARTESIAN_POINT ( 'NONE',  ( -1.526197323679999940, -100.8869817940000075, -15.59251925729999932 ) ) ;
#17764=AXIS2_PLACEMENT_3D ( 'NONE', #13140, #22053, #4118 ) ;
#17771=EDGE_CURVE ( 'NONE', #22153, #726, #3721, .T. ) ;
#17774=CARTESIAN_POINT ( 'NONE',  ( 3.129685915889999670, -92.55031878719999838, -28.46238550929999889 ) ) ;
#17776=LINE ( 'NONE', #11024, #1548 ) ;
#17781=CARTESIAN_POINT ( 'NONE',  ( 21.88853012090000050, -95.77248565319999329, -4.561213946619999682 ) ) ;
#17785=ORIENTED_EDGE ( 'NONE', *, *, #7823, .T. ) ;
#17787=CARTESIAN_POINT ( 'NONE',  ( 16.08037959500000014, -101.3150700380000018, 2.354223078750000031 ) ) ;
#17788=CARTESIAN_POINT ( 'NONE',  ( -11.17102524760000115, -94.77696045309998851, -20.89250772250000310 ) ) ;
#17791=CARTESIAN_POINT ( 'NONE',  ( -18.87705750089999768, -97.64875668899999539, 6.521983386959999685 ) ) ;
#17794=ORIENTED_EDGE ( 'NONE', *, *, #23307, .F. ) ;
#17795=CARTESIAN_POINT ( 'NONE',  ( 11.67094882200000150, -93.01584738609999192, -23.70866791699999965 ) ) ;
#17797=CARTESIAN_POINT ( 'NONE',  ( 0.000000000000000000, -94.59276292389999696, 0.000000000000000000 ) ) ;
#17798=CARTESIAN_POINT ( 'NONE',  ( -13.12698473016186895, -92.72059904818586062, 27.53057009221356921 ) ) ;
#17802=CARTESIAN_POINT ( 'NONE',  ( -14.45493179810000051, -92.91908509549999451, 26.19282653499999824 ) ) ;
#17803=CARTESIAN_POINT ( 'NONE',  ( -11.32307664120000013, -111.0000000000000000, 9.421136869679999748 ) ) ;
#17807=CARTESIAN_POINT ( 'NONE',  ( 0.6052036509410000376, -100.3063911739999980, -17.04494785839999693 ) ) ;
#17811=TOROIDAL_SURFACE ( 'NONE', #22950, 29.91857981989999971, 10.00000000000000000 ) ;
#17812=ADVANCED_FACE ( 'NONE', ( #25874 ), #10383, .F. ) ;
#17813=CARTESIAN_POINT ( 'NONE',  ( 0.000000000000000000, -90.50000000000000000, 0.000000000000000000 ) ) ;
#17814=EDGE_LOOP ( 'NONE', ( #20341, #10801, #802 ) ) ;
#17815=CARTESIAN_POINT ( 'NONE',  ( -17.49492164999999844, -94.26879627710000875, 16.77352930379999663 ) ) ;
#17819=CARTESIAN_POINT ( 'NONE',  ( 23.18113824346705698, -92.50630337894787658, -19.82174805298759424 ) ) ;
#17820=CARTESIAN_POINT ( 'NONE',  ( 18.40795691769999820, -93.85307999900000198, 16.77768149470000125 ) ) ;
#17821=CARTESIAN_POINT ( 'NONE',  ( 11.36572001294154788, -99.82487968003715650, -12.74458838826810236 ) ) ;
#17822=CARTESIAN_POINT ( 'NONE',  ( -7.380602427890000428, -101.2251655520000071, 14.44694227429999955 ) ) ;
#17825=CARTESIAN_POINT ( 'NONE',  ( -12.50561141126462950, -101.1248211534225163, -10.62038857907609746 ) ) ;
#17830=DIRECTION ( 'NONE',  ( 1.000000000000000000, 0.000000000000000000, 0.000000000000000000 ) ) ;
#17832=CARTESIAN_POINT ( 'NONE',  ( 0.7331249433679999372, -99.53431242750001218, -17.39855866090000092 ) ) ;
#17834=CARTESIAN_POINT ( 'NONE',  ( 11.14159932559999966, -101.1364147039999892, -10.55279472049999967 ) ) ;
#17836=CARTESIAN_POINT ( 'NONE',  ( 15.28191216724069612, -95.14282497074401590, 17.30484737853460686 ) ) ;
#17837=EDGE_CURVE ( 'NONE', #5717, #14760, #24852, .T. ) ;
#17838=DIRECTION ( 'NONE',  ( 0.000000000000000000, 1.000000000000000000, 0.000000000000000000 ) ) ;
#17842=CARTESIAN_POINT ( 'NONE',  ( 8.125631349740000786, -93.00000000000000000, 24.17072847820000092 ) ) ;
#17844=CARTESIAN_POINT ( 'NONE',  ( 24.64422047424358553, -93.08694455160397752, -15.44790685958040655 ) ) ;
#17845=CARTESIAN_POINT ( 'NONE',  ( 25.04472665119416419, -93.40025063799829752, 11.65239934674920796 ) ) ;
#17850=ORIENTED_EDGE ( 'NONE', *, *, #8435, .F. ) ;
#17853=CARTESIAN_POINT ( 'NONE',  ( -24.18521206880000207, -94.16309976690000383, -3.351640123200000154 ) ) ;
#17854=CARTESIAN_POINT ( 'NONE',  ( 11.86655840719999944, -111.0000000000000000, -11.10431293650000129 ) ) ;
#17855=AXIS2_PLACEMENT_3D ( 'NONE', #16766, #14302, #23478 ) ;
#17860=CARTESIAN_POINT ( 'NONE',  ( 5.750078808689999654, -92.99020741600000406, 26.05463881579999708 ) ) ;
#17864=CARTESIAN_POINT ( 'NONE',  ( 7.915433586269055688, -92.54687141712493315, 29.45498200392744437 ) ) ;
#17866=CARTESIAN_POINT ( 'NONE',  ( 7.910521386969999291, -107.1975888269999899, 14.48011227119999944 ) ) ;
#17868=AXIS2_PLACEMENT_3D ( 'NONE', #26951, #450, #27386 ) ;
#17870=CARTESIAN_POINT ( 'NONE',  ( 23.60843678869999707, -92.50000947299999154, -18.49675587200000137 ) ) ;
#17872=CARTESIAN_POINT ( 'NONE',  ( 15.60567172371994005, -96.61062824143314742, 14.39926977216421911 ) ) ;
#17873=CARTESIAN_POINT ( 'NONE',  ( -16.78971427428115604, -98.15124914739722328, 9.315172230392416708 ) ) ;
#17878=DIRECTION ( 'NONE',  ( 0.000000000000000000, -1.000000000000000000, 0.000000000000000000 ) ) ;
#17884=VERTEX_POINT ( 'NONE', #26158 ) ;
#17893=CARTESIAN_POINT ( 'NONE',  ( -26.03320226835694484, -93.98969193916619247, -2.031746379724110430 ) ) ;
#17894=CARTESIAN_POINT ( 'NONE',  ( 20.70184870579999981, -94.64125193980000006, 13.94635761189999812 ) ) ;
#17901=CARTESIAN_POINT ( 'NONE',  ( -17.80822692750000158, -93.00000000000000000, -18.25149456069999943 ) ) ;
#17903=CARTESIAN_POINT ( 'NONE',  ( -11.77049175780000034, -94.59276292120000562, -20.68200896629999974 ) ) ;
#17904=DIRECTION ( 'NONE',  ( 0.4794255386042041156, 0.000000000000000000, 0.8775825618903722036 ) ) ;
#17906=EDGE_CURVE ( 'NONE', #2020, #1715, #14171, .T. ) ;
#17907=CARTESIAN_POINT ( 'NONE',  ( -18.05096283909999855, -93.00000167610001256, -23.30076369320000040 ) ) ;
#17908=B_SPLINE_CURVE_WITH_KNOTS ( 'NONE', 3,
 ( #18354, #18494, #5382, #27387, #25206, #14265, #1041, #3203, #14122, #3070, #9879, #7723, #23295, #16590, #23849, #28356, #8121, #19064, #21382, #17010, #21526, #12889, #25898, #10700, #6356, #10286, #17443, #1301, #27948, #28502, #10423, #7985, #1443, #12614, #8388, #13047, #26185, #21665, #17147, #26035, #17294, #25765, #15219, #1582, #23707, #24135, #10143, #14807, #23992, #4171, #16878, #19341, #6216, #4027, #5794, #21805, #28217, #19196, #8251, #8538 ),
 .UNSPECIFIED., .F., .F.,
 ( 4, 2, 1, 1, 2, 2, 2, 2, 1, 1, 2, 2, 2, 2, 2, 2, 2, 1, 1, 2, 2, 2, 2, 1, 2, 2, 2, 1, 2, 2, 2, 2, 2, 4 ),
 ( 0.000000000000000000, 0.06250000000016231461, 0.09375000000024402702, 0.1093750000002796374, 0.1171875000002974010, 0.1250000000003151646, 0.1875000000004634071, 0.2187500000005324075, 0.2343750000005663525, 0.2421875000005828948, 0.2460937500005904999, 0.2500000000005981327, 0.3125000000005603296, 0.3437500000005472844, 0.3750000000005342393, 0.4375000000005085377, 0.4687500000004952150, 0.4843750000004883316, 0.4921875000004846124, 0.4960937500004830580, 0.5000000000004815037, 0.5625000000004248824, 0.5937500000003965717, 0.6093750000003884670, 0.6171875000003848033, 0.6250000000003811396, 0.6875000000003268497, 0.7187500000002994271, 0.7343750000002854383, 0.7500000000002715606, 0.8125000000002049472, 0.8437500000001668665, 0.8750000000001287859, 1.000000000000000000 ),
 .UNSPECIFIED. ) ;
#17909=CARTESIAN_POINT ( 'NONE',  ( 13.82409059959999809, -99.78393592979999482, -10.43876300910000055 ) ) ;
#17912=CARTESIAN_POINT ( 'NONE',  ( -11.71096558855141190, -94.52293547163276344, -20.87034194758490813 ) ) ;
#17920=CARTESIAN_POINT ( 'NONE',  ( -24.36269809241420958, -92.52640451560269241, -18.34963895739831941 ) ) ;
#17924=B_SPLINE_CURVE_WITH_KNOTS ( 'NONE', 5,
 ( #475, #15877, #5108, #4959, #622, #11494 ),
 .UNSPECIFIED., .F., .F.,
 ( 6, 6 ),
 ( 0.000000000000000000, 1.000000000000000000 ),
 .UNSPECIFIED. ) ;
#17936=CARTESIAN_POINT ( 'NONE',  ( 6.042832004899746146, -93.45279863444233115, -26.77704013367506519 ) ) ;
#17938=CARTESIAN_POINT ( 'NONE',  ( -19.97974828950000159, -95.94978106879999302, 10.41054471420000027 ) ) ;
#17944=CARTESIAN_POINT ( 'NONE',  ( 0.000000000000000000, -102.5000000000000000, 0.000000000000000000 ) ) ;
#17945=CARTESIAN_POINT ( 'NONE',  ( -12.92668336025674414, -92.62938374235253036, 27.62520349261831498 ) ) ;
#17946=ORIENTED_EDGE ( 'NONE', *, *, #26793, .F. ) ;
#17947=FACE_OUTER_BOUND ( 'NONE', #12737, .T. ) ;
#17948=CARTESIAN_POINT ( 'NONE',  ( -14.87798422589999880, -92.52476525819999154, 24.84728676379999968 ) ) ;
#17952=CARTESIAN_POINT ( 'NONE',  ( 1.080755419719999999, -99.91102932019998661, -16.89321760849999876 ) ) ;
#17957=DIRECTION ( 'NONE',  ( 0.000000000000000000, -1.000000000000000000, 0.000000000000000000 ) ) ;
#17959=ORIENTED_EDGE ( 'NONE', *, *, #3072, .F. ) ;
#17961=CARTESIAN_POINT ( 'NONE',  ( 15.11062958683252511, -101.1604341566294920, 2.739549772153475615 ) ) ;
#17964=CARTESIAN_POINT ( 'NONE',  ( 23.09404321033341034, -92.49999999999997158, -19.92320476265976481 ) ) ;
#17965=CARTESIAN_POINT ( 'NONE',  ( 18.38388831859999684, -93.67869433859999617, 16.94838898949999972 ) ) ;
#17966=EDGE_CURVE ( 'NONE', #20274, #21210, #28478, .T. ) ;
#17968=ORIENTED_EDGE ( 'NONE', *, *, #7540, .F. ) ;
#17970=CARTESIAN_POINT ( 'NONE',  ( -12.45338840115624990, -101.3586211803998367, -10.39906174622668189 ) ) ;
#17975=DIRECTION ( 'NONE',  ( 0.000000000000000000, 1.000000000000000000, 0.000000000000000000 ) ) ;
#17977=CARTESIAN_POINT ( 'NONE',  ( -2.004260180370000199, -97.53592492889998766, -19.96958033499999985 ) ) ;
#17978=FACE_OUTER_BOUND ( 'NONE', #12982, .T. ) ;
#17979=ORIENTED_EDGE ( 'NONE', *, *, #12413, .T. ) ;
#17980=CARTESIAN_POINT ( 'NONE',  ( 11.78180866139999949, -101.1659666750000071, -10.84551784730000001 ) ) ;
#17982=CARTESIAN_POINT ( 'NONE',  ( -19.03193910350634610, -98.07255008389248019, -7.553244766087960471 ) ) ;
#17991=CARTESIAN_POINT ( 'NONE',  ( 8.140397668380000340, -100.8869818179999953, 13.38618156149999905 ) ) ;
#17993=CARTESIAN_POINT ( 'NONE',  ( -5.873418876839999747, -111.0000000000000000, 15.15334698740000086 ) ) ;
#18000=CARTESIAN_POINT ( 'NONE',  ( 16.78330657029999884, -99.55609327400000552, 4.537757829670000298 ) ) ;
#18004=CARTESIAN_POINT ( 'NONE',  ( -19.68882303210000018, -96.97547176739999486, -6.799171120899999643 ) ) ;
#18005=ORIENTED_EDGE ( 'NONE', *, *, #17487, .F. ) ;
#18007=CARTESIAN_POINT ( 'NONE',  ( 0.4174863123245782792, -99.84800943039545018, -17.32495207964082695 ) ) ;
#18014=CARTESIAN_POINT ( 'NONE',  ( -16.14916233553648794, -99.20418361269911145, 7.582005830281769221 ) ) ;
#18017=CARTESIAN_POINT ( 'NONE',  ( -15.50938051129999984, -101.3150705480000084, 4.855933523060000034 ) ) ;
#18018=CARTESIAN_POINT ( 'NONE',  ( -3.363116624290108270, -98.28141829459690371, 19.92205903335984374 ) ) ;
#18019=CARTESIAN_POINT ( 'NONE',  ( -12.86641141129999966, -100.1981337080000003, -11.08525741000000053 ) ) ;
#18023=EDGE_CURVE ( 'NONE', #17343, #23088, #10400, .T. ) ;
#18024=CARTESIAN_POINT ( 'NONE',  ( 26.68762699244526004, -92.64884742711814170, -14.76556618572936763 ) ) ;
#18027=AXIS2_PLACEMENT_3D ( 'NONE', #21563, #16625, #6104 ) ;
#18028=CARTESIAN_POINT ( 'NONE',  ( -7.910521386969999291, -107.1975888269999899, -14.48011227119999944 ) ) ;
#18029=CARTESIAN_POINT ( 'NONE',  ( 11.26951408729999926, -92.92894616350000092, 27.60410696470000147 ) ) ;
#18034=CARTESIAN_POINT ( 'NONE',  ( -27.45034045483756913, -93.45279863387368380, 0.06712639151115551428 ) ) ;
#18035=CARTESIAN_POINT ( 'NONE',  ( 19.57843401649999748, -94.59276292120000562, 13.52682122920000118 ) ) ;
#18040=VECTOR ( 'NONE', #9207, 1000.000000000000000 ) ;
#18041=ADVANCED_FACE ( 'NONE', ( #27621 ), #25289, .T. ) ;
#18042=CARTESIAN_POINT ( 'NONE',  ( -0.7205257401510000159, -111.0000000000000000, -15.98376809950000066 ) ) ;
#18046=CARTESIAN_POINT ( 'NONE',  ( -2.876553231629999985, -100.0000000000000000, -5.265495371340000119 ) ) ;
#18051=CYLINDRICAL_SURFACE ( 'NONE', #8733, 5.000000000000000000 ) ;
#18052=CARTESIAN_POINT ( 'NONE',  ( 1.080755419719999999, -99.91102932019998661, -16.89321760849999876 ) ) ;
#18053=CARTESIAN_POINT ( 'NONE',  ( 21.75659477429999811, -93.00000000000000000, -13.30039788230000042 ) ) ;
#18058=CARTESIAN_POINT ( 'NONE',  ( 3.116266000930000057, -91.00000000000000000, 5.704286652290000426 ) ) ;
#18059=CARTESIAN_POINT ( 'NONE',  ( -23.77086693186838318, -92.96960399591381474, -19.11009903990889569 ) ) ;
#18063=AXIS2_PLACEMENT_3D ( 'NONE', #26148, #19011, #12291 ) ;
#18069=CARTESIAN_POINT ( 'NONE',  ( 14.28941763439999946, -93.00000000000000000, -3.575252188409999921 ) ) ;
#18078=DIRECTION ( 'NONE',  ( 1.000000000000000000, 0.000000000000000000, 0.000000000000000000 ) ) ;
#18079=CARTESIAN_POINT ( 'NONE',  ( -18.07120458720000045, -98.58299283580001315, 4.768611213479999833 ) ) ;
#18083=CARTESIAN_POINT ( 'NONE',  ( 8.660164454169999360, -92.99999854809999533, -27.14861362650000132 ) ) ;
#18086=ORIENTED_EDGE ( 'NONE', *, *, #21392, .T. ) ;
#18090=ORIENTED_EDGE ( 'NONE', *, *, #10305, .T. ) ;
#18095=EDGE_CURVE ( 'NONE', #11312, #18883, #5591, .T. ) ;
#18098=B_SPLINE_CURVE_WITH_KNOTS ( 'NONE', 5,
 ( #18017, #28779, #10982, #22103, #118, #15216 ),
 .UNSPECIFIED., .F., .F.,
 ( 6, 6 ),
 ( 0.000000000000000000, 1.000000000000000000 ),
 .UNSPECIFIED. ) ;
#18101=DIRECTION ( 'NONE',  ( -0.000000000000000000, 1.000000000000000000, 0.000000000000000000 ) ) ;
#18103=ADVANCED_FACE ( 'NONE', ( #3282 ), #13758, .F. ) ;
#18107=CIRCLE ( 'NONE', #15757, 11.00000000000000000 ) ;
#18110=CARTESIAN_POINT ( 'NONE',  ( 15.71723844345814669, -101.4628082233788007, 2.849527662385800575 ) ) ;
#18112=CARTESIAN_POINT ( 'NONE',  ( 8.069589370679999263, -101.0685846549999951, 13.92289990319999937 ) ) ;
#18115=CARTESIAN_POINT ( 'NONE',  ( 9.273485931230000645, -94.57749572790000059, -22.35124366870000046 ) ) ;
#18116=CARTESIAN_POINT ( 'NONE',  ( 9.872833180276398224, -95.57586223587027519, -20.31377284688967322 ) ) ;
#18124=CARTESIAN_POINT ( 'NONE',  ( -15.44795072159999982, -101.4309506800000094, 4.757508573860000034 ) ) ;
#18126=CARTESIAN_POINT ( 'NONE',  ( 12.69538180190852295, -96.41991180888999224, 17.27318304392874282 ) ) ;
#18137=CARTESIAN_POINT ( 'NONE',  ( 22.48362994130000203, -95.75647260700000629, -0.6182000987479999710 ) ) ;
#18148=CARTESIAN_POINT ( 'NONE',  ( -21.85149396670000144, -95.71128647580000859, -5.653426733619999922 ) ) ;
#18152=CARTESIAN_POINT ( 'NONE',  ( 7.457144889719999448, -101.1889999979999999, 15.05426816870000017 ) ) ;
#18160=CARTESIAN_POINT ( 'NONE',  ( -16.72707404650564200, -98.26662831810237719, 9.119458534568265051 ) ) ;
#18167=CARTESIAN_POINT ( 'NONE',  ( 15.48443774817907581, -95.52016638765006462, 17.06274023349215341 ) ) ;
#18175=CARTESIAN_POINT ( 'NONE',  ( -0.6492686798639999424, -95.71128647790000343, 22.56163718579999866 ) ) ;
#18176=CARTESIAN_POINT ( 'NONE',  ( 2.585535234560000006, -94.10359775160000595, 25.24649707500000062 ) ) ;
#18188=AXIS2_PLACEMENT_3D ( 'NONE', #14268, #1446, #14409 ) ;
#18191=CARTESIAN_POINT ( 'NONE',  ( -13.23488380210000059, -93.86380869100000268, -21.19624334839999946 ) ) ;
#18193=ORIENTED_EDGE ( 'NONE', *, *, #3226, .F. ) ;
#18203=CARTESIAN_POINT ( 'NONE',  ( -13.14594991939999957, -93.06131880550000801, -23.62747753289999864 ) ) ;
#18205=CARTESIAN_POINT ( 'NONE',  ( 23.63615965700000032, -94.63960343439998724, -2.179844538739999837 ) ) ;
#18206=DIRECTION ( 'NONE',  ( 0.3390050494208429743, 0.7071067811866730279, 0.6205445805637129775 ) ) ;
#18207=CARTESIAN_POINT ( 'NONE',  ( 15.64127366367332961, -101.5409490182698136, 3.743084204742448851 ) ) ;
#18217=CARTESIAN_POINT ( 'NONE',  ( 7.561439849066408314, -93.25520180122281033, 27.12672954078378851 ) ) ;
#18226=CARTESIAN_POINT ( 'NONE',  ( 3.258717473867890124, -93.08494709823048652, -28.91753983529492444 ) ) ;
#18227=CARTESIAN_POINT ( 'NONE',  ( -25.14533482850000112, -93.65023913320000304, -2.072137388280000270 ) ) ;
#18228=CARTESIAN_POINT ( 'NONE',  ( -17.05468887140000334, -99.57787288160000116, 3.230412712340000159 ) ) ;
#18230=VECTOR ( 'NONE', #18399, 1000.000000000000000 ) ;
#18231=CARTESIAN_POINT ( 'NONE',  ( 11.63638030983188543, -98.17436949440750027, -16.68664549751153814 ) ) ;
#18232=ORIENTED_EDGE ( 'NONE', *, *, #27023, .T. ) ;
#18235=CARTESIAN_POINT ( 'NONE',  ( -12.51597748458882187, -92.53260370674736635, 27.81370878362392673 ) ) ;
#18239=CARTESIAN_POINT ( 'NONE',  ( -14.42556421679999978, -92.50000000000000000, -2.978755036369999942 ) ) ;
#18244=CARTESIAN_POINT ( 'NONE',  ( 0.4053730124380000022, -99.88067631459999518, -17.33742933230000105 ) ) ;
#18245=CARTESIAN_POINT ( 'NONE',  ( -8.047735417340286190, -99.62767017965474281, 15.35597723112435986 ) ) ;
#18251=AXIS2_PLACEMENT_3D ( 'NONE', #6746, #11382, #13731 ) ;
#18252=ORIENTED_EDGE ( 'NONE', *, *, #11498, .T. ) ;
#18254=CARTESIAN_POINT ( 'NONE',  ( 15.74335372269999844, -101.6484611540000031, 2.854262350110000401 ) ) ;
#18255=CARTESIAN_POINT ( 'NONE',  ( 10.22067991429999978, -99.82967889459999355, 14.73214614719999815 ) ) ;
#18256=ORIENTED_EDGE ( 'NONE', *, *, #12834, .T. ) ;
#18262=CARTESIAN_POINT ( 'NONE',  ( -7.525338988669999729, -101.1976625110000043, 14.51486394580000017 ) ) ;
#18269=CARTESIAN_POINT ( 'NONE',  ( 8.435807852960000019, -99.08524068509998983, 16.22846277789999903 ) ) ;
#18272=CARTESIAN_POINT ( 'NONE',  ( -5.478138399269999681, -95.60035679220000304, -21.87686786650000315 ) ) ;
#18275=CARTESIAN_POINT ( 'NONE',  ( 11.15108561449999947, -100.9197086960000007, -10.94438850839999944 ) ) ;
#18278=CARTESIAN_POINT ( 'NONE',  ( 12.70280709945315145, -96.41616466973447075, 17.27373141714811666 ) ) ;
#18283=CARTESIAN_POINT ( 'NONE',  ( 24.72975223188596061, -93.15741110475592279, -14.44177324630790871 ) ) ;
#18289=CARTESIAN_POINT ( 'NONE',  ( 7.859829845370000179, -101.5882635180000051, 13.98896253659999900 ) ) ;
#18298=CARTESIAN_POINT ( 'NONE',  ( -11.85289063449999958, -94.98812477599999227, -21.44324726029999795 ) ) ;
#18299=CARTESIAN_POINT ( 'NONE',  ( 16.79922304909999653, -99.53431386179998697, 4.586272534879999974 ) ) ;
#18302=CARTESIAN_POINT ( 'NONE',  ( -23.85440681869999935, -94.57749834670001121, -4.067368795410000182 ) ) ;
#18304=CARTESIAN_POINT ( 'NONE',  ( 9.139220208361530595, -92.82668962667709422, 29.09853360705717407 ) ) ;
#18307=B_SPLINE_CURVE_WITH_KNOTS ( 'NONE', 5,
 ( #18357, #18205, #7142, #4944, #13825, #22730 ),
 .UNSPECIFIED., .F., .F.,
 ( 6, 6 ),
 ( 0.000000000000000000, 1.000000000000000000 ),
 .UNSPECIFIED. ) ;
#18311=CARTESIAN_POINT ( 'NONE',  ( 23.05497096699999915, -94.52419443349998573, -6.735187176270000187 ) ) ;
#18313=CARTESIAN_POINT ( 'NONE',  ( 20.68887087950000137, -111.0000000000000000, -4.764889194739999390 ) ) ;
#18315=CARTESIAN_POINT ( 'NONE',  ( -17.53890950007582461, -96.04266803764619453, 13.15491836168024342 ) ) ;
#18318=DIRECTION ( 'NONE',  ( 0.000000000000000000, -1.000000000000000000, 0.000000000000000000 ) ) ;
#18319=CARTESIAN_POINT ( 'NONE',  ( -13.14566789610000086, -99.53431386179998697, -11.42099848439999832 ) ) ;
#18320=AXIS2_PLACEMENT_3D ( 'NONE', #13805, #1021, #9865 ) ;
#18324=CARTESIAN_POINT ( 'NONE',  ( 26.43197680980085451, -92.77481473413912738, -15.21859952970796037 ) ) ;
#18330=CARTESIAN_POINT ( 'NONE',  ( 11.26907854689999944, -92.50633975910000117, 27.15731767689999998 ) ) ;
#18332=CARTESIAN_POINT ( 'NONE',  ( -25.41320261003370717, -94.27895761423600618, -2.788869183902775717 ) ) ;
#18333=CARTESIAN_POINT ( 'NONE',  ( -14.05779758289999926, -93.65023913340000661, -20.95137093579999998 ) ) ;
#18340=CARTESIAN_POINT ( 'NONE',  ( -2.995163666639999889, -99.62704707150000161, -17.08389978359999972 ) ) ;
#18345=EDGE_CURVE ( 'NONE', #5924, #24500, #159, .T. ) ;
#18348=CARTESIAN_POINT ( 'NONE',  ( 13.96614599839999826, -99.72202992580000114, -9.992871978760000218 ) ) ;
#18354=CARTESIAN_POINT ( 'NONE',  ( -7.879410208250000380, -99.92967571559999840, 15.46934584979999983 ) ) ;
#18356=CARTESIAN_POINT ( 'NONE',  ( -8.359358578160000164, -94.05619169260000945, -23.03490865379999875 ) ) ;
#18357=CARTESIAN_POINT ( 'NONE',  ( 23.70295537799999863, -94.59276292389999696, -2.111841813949999924 ) ) ;
#18359=CARTESIAN_POINT ( 'NONE',  ( 16.62043402502380118, -100.1585711159323040, 4.330280467225621877 ) ) ;
#18366=VECTOR ( 'NONE', #210, 1000.000000000000000 ) ;
#18369=CARTESIAN_POINT ( 'NONE',  ( 9.170936544316921513, -93.11246772311548625, 27.41354572203813689 ) ) ;
#18376=VERTEX_POINT ( 'NONE', #23069 ) ;
#18379=CARTESIAN_POINT ( 'NONE',  ( 7.784722820381165143, -93.99439547206506518, -24.91492963938277683 ) ) ;
#18394=CARTESIAN_POINT ( 'NONE',  ( -16.57262828550000222, -99.75088961650000385, 6.665555775249999648 ) ) ;
#18399=DIRECTION ( 'NONE',  ( 0.000000000000000000, 1.000000000000000000, 0.000000000000000000 ) ) ;
#18400=DIRECTION ( 'NONE',  ( 0.000000000000000000, 1.000000000000000000, 0.000000000000000000 ) ) ;
#18402=CARTESIAN_POINT ( 'NONE',  ( 9.119802927630001221, -98.28914429610000525, 16.69368728350000097 ) ) ;
#18407=CARTESIAN_POINT ( 'NONE',  ( 8.099918789429999322, -100.8733985849999897, 13.47813349329999966 ) ) ;
#18412=CARTESIAN_POINT ( 'NONE',  ( -13.25045755180000029, -111.0000000000000000, -10.32789304109999939 ) ) ;
#18413=CARTESIAN_POINT ( 'NONE',  ( -11.18981136662480402, -93.70622791291684450, -23.36782803959924237 ) ) ;
#18416=ORIENTED_EDGE ( 'NONE', *, *, #19311, .T. ) ;
#18419=CARTESIAN_POINT ( 'NONE',  ( -3.701677221209999757, -96.58372172920000764, -20.98007619770000076 ) ) ;
#18422=CARTESIAN_POINT ( 'NONE',  ( 11.87346201969999981, -101.4334236450000049, -10.82497022220000105 ) ) ;
#18424=CARTESIAN_POINT ( 'NONE',  ( -19.02660535542675646, -98.07566646017912149, -7.555665490820644870 ) ) ;
#18430=CARTESIAN_POINT ( 'NONE',  ( -14.81560312809999935, -101.2530993080000030, 3.374019831970000105 ) ) ;
#18433=CARTESIAN_POINT ( 'NONE',  ( 6.638698704379999427, -101.1284992150000051, 13.90181459059999902 ) ) ;
#18434=FACE_OUTER_BOUND ( 'NONE', #99, .T. ) ;
#18435=CARTESIAN_POINT ( 'NONE',  ( 8.042004129799998680, -100.9405349759999950, 13.76814388520000065 ) ) ;
#18438=CARTESIAN_POINT ( 'NONE',  ( 23.58467321619999879, -94.98812477769999418, -2.405347530869999861 ) ) ;
#18444=CARTESIAN_POINT ( 'NONE',  ( 0.4008318592790000578, -92.76843000840000286, -30.33740225879999741 ) ) ;
#18447=CARTESIAN_POINT ( 'NONE',  ( 16.24108910990000254, -99.94549701829998867, 4.679412117860000109 ) ) ;
#18451=ORIENTED_EDGE ( 'NONE', *, *, #976, .T. ) ;
#18452=CARTESIAN_POINT ( 'NONE',  ( -30.46635619948354190, -92.59033770620612813, 1.439011912417819783 ) ) ;
#18453=VERTEX_POINT ( 'NONE', #3521 ) ;
#18454=FACE_OUTER_BOUND ( 'NONE', #7507, .T. ) ;
#18455=DIRECTION ( 'NONE',  ( -0.8775825618903722036, 0.000000000000000000, 0.4794255386042041156 ) ) ;
#18460=CARTESIAN_POINT ( 'NONE',  ( 23.82963719045704920, -92.77521214511682501, -19.03680056186108160 ) ) ;
#18466=CARTESIAN_POINT ( 'NONE',  ( 15.89272830319999841, -101.5317765570000006, 2.499482219129999905 ) ) ;
#18471=B_SPLINE_CURVE_WITH_KNOTS ( 'NONE', 3,
 ( #983, #25570, #18877, #5743, #10092, #10371, #19010, #5463, #16671, #27630 ),
 .UNSPECIFIED., .F., .F.,
 ( 4, 2, 2, 2, 4 ),
 ( 0.000000000000000000, 0.2500000000000000555, 0.5000000000000001110, 0.7500000000000002220, 1.000000000000000000 ),
 .UNSPECIFIED. ) ;
#18474=CARTESIAN_POINT ( 'NONE',  ( 1.338305831620000053, -94.89419512579999605, 24.43791469299999974 ) ) ;
#18475=EDGE_CURVE ( 'NONE', #22947, #5288, #6647, .T. ) ;
#18479=DIRECTION ( 'NONE',  ( 0.000000000000000000, 1.000000000000000000, 0.000000000000000000 ) ) ;
#18481=EDGE_LOOP ( 'NONE', ( #25113, #4955, #9103, #10986 ) ) ;
#18489=CARTESIAN_POINT ( 'NONE',  ( -14.95917775459999888, -101.1625380809999939, 3.268662194040000024 ) ) ;
#18492=DIRECTION ( 'NONE',  ( 0.2116638115179449164, 0.000000000000000000, -0.9773425350887455787 ) ) ;
#18494=CARTESIAN_POINT ( 'NONE',  ( -7.891227027390866233, -99.96200787829550904, 15.43388765503441462 ) ) ;
#18495=ORIENTED_EDGE ( 'NONE', *, *, #14414, .F. ) ;
#18504=B_SPLINE_SURFACE_WITH_KNOTS ( 'NONE', 5, 5, ( 
 ( #6668, #6363, #15681, #15534, #24586, #8679, #4336, #4627, #6521 ),
 ( #2456, #13208, #11311, #20213, #28513, #12900, #10708, #19626, #9709 ),
 ( #16422, #18029, #12036, #15831, #25182, #13654, #2742, #18330, #13796 ),
 ( #5213, #284, #13949, #6969, #7404, #14244, #20507, #427, #26927 ),
 ( #4777, #9128, #4919, #11450, #22700, #7563, #22562, #27217, #578 ),
 ( #24741, #24884, #22849, #7116, #2894, #11752, #16269, #25025, #27362 ),
 ( #25331, #7259, #9277, #20358, #16125, #11599, #5359, #5057, #20665 ),
 ( #722, #2602, #18176, #3179, #9423, #27073, #15978, #14098, #18622 ),
 ( #9573, #18474, #22996, #3047, #11898, #20808, #867, #27514, #23132 ) ),
 .UNSPECIFIED., .F., .F., .F.,
 ( 6, 3, 6 ),
 ( 6, 3, 6 ),
 ( 2.722996918069999772, 8.105704033360000338, 20.61863289369999919 ),
 ( 0.000000000000000000, 0.2500000000000000000, 0.5000000000000000000 ),
 .UNSPECIFIED. ) ;
#18508=CARTESIAN_POINT ( 'NONE',  ( 3.427474320454169110, -94.10913273187073003, 25.64827485542228658 ) ) ;
#18510=ORIENTED_EDGE ( 'NONE', *, *, #28239, .F. ) ;
#18515=CARTESIAN_POINT ( 'NONE',  ( -5.641490680649999589, -101.0555477039999914, 14.43351876059999839 ) ) ;
#18516=ORIENTED_EDGE ( 'NONE', *, *, #13572, .F. ) ;
#18527=CARTESIAN_POINT ( 'NONE',  ( 12.53708103959999853, -93.63284696309999333, -21.72543968509999956 ) ) ;
#18529=DIRECTION ( 'NONE',  ( 0.000000000000000000, 1.000000000000000000, 0.000000000000000000 ) ) ;
#18536=CARTESIAN_POINT ( 'NONE',  ( -18.26810489620000055, -94.98812477769999418, 16.32728500220000001 ) ) ;
#18541=EDGE_CURVE ( 'NONE', #16504, #4122, #15959, .T. ) ;
#18549=CARTESIAN_POINT ( 'NONE',  ( 17.21463605679999986, -95.70830672179999965, 14.46803396139999975 ) ) ;
#18553=AXIS2_PLACEMENT_3D ( 'NONE', #13619, #15795, #22666 ) ;
#18554=CIRCLE ( 'NONE', #901, 5.500000000000000000 ) ;
#18556=CARTESIAN_POINT ( 'NONE',  ( 14.28941763439999946, -111.0000000000000000, -3.575252188409999921 ) ) ;
#18557=CARTESIAN_POINT ( 'NONE',  ( -10.27834059868025207, -93.94676096557853384, -23.20073146982036860 ) ) ;
#18563=EDGE_CURVE ( 'NONE', #4106, #11899, #17776, .T. ) ;
#18565=CARTESIAN_POINT ( 'NONE',  ( 11.86104730819999986, -101.2306310700000012, -11.05401091329999907 ) ) ;
#18571=CARTESIAN_POINT ( 'NONE',  ( -17.05193907084168004, -92.82668962665341894, 25.28796903711848643 ) ) ;
#18579=EDGE_CURVE ( 'NONE', #22634, #8616, #23994, .T. ) ;
#18582=CARTESIAN_POINT ( 'NONE',  ( -18.34989813179999985, -93.00000000000000000, 23.56346505449999995 ) ) ;
#18589=CARTESIAN_POINT ( 'NONE',  ( 0.2881167279619999966, -92.51542729400000553, -30.06300816579999946 ) ) ;
#18591=DIRECTION ( 'NONE',  ( 0.000000000000000000, 1.000000000000000000, 0.000000000000000000 ) ) ;
#18596=CARTESIAN_POINT ( 'NONE',  ( -15.60055607610000195, -99.82967635429999120, -8.838619376430001395 ) ) ;
#18597=ORIENTED_EDGE ( 'NONE', *, *, #17702, .F. ) ;
#18598=CARTESIAN_POINT ( 'NONE',  ( -30.42316450781055792, -92.75430643196618519, 2.164184228886041339 ) ) ;
#18599=ORIENTED_EDGE ( 'NONE', *, *, #11114, .F. ) ;
#18600=CIRCLE ( 'NONE', #23688, 16.00000000000000000 ) ;
#18602=AXIS2_PLACEMENT_3D ( 'NONE', #283, #26926, #13206 ) ;
#18603=CARTESIAN_POINT ( 'NONE',  ( 0.4681305316614765566, -101.2021794473764658, -16.33959806313605512 ) ) ;
#18609=CARTESIAN_POINT ( 'NONE',  ( 14.19394574969999923, -96.53848370309999893, -15.96642820140000296 ) ) ;
#18615=CARTESIAN_POINT ( 'NONE',  ( 13.12744653600000078, -94.59276292389999696, -19.84842857619999990 ) ) ;
#18616=ORIENTED_EDGE ( 'NONE', *, *, #14301, .T. ) ;
#18618=AXIS2_PLACEMENT_3D ( 'NONE', #10644, #19557, #24226 ) ;
#18621=CARTESIAN_POINT ( 'NONE',  ( 1.495914020609999895, -94.52293512119999264, 23.88472631159999793 ) ) ;
#18622=CARTESIAN_POINT ( 'NONE',  ( 2.842132195609999634, -93.86302664969998943, 24.60248089030000074 ) ) ;
#18628=CARTESIAN_POINT ( 'NONE',  ( 0.000000000000000000, -91.50000000000000000, 0.000000000000000000 ) ) ;
#18637=EDGE_CURVE ( 'NONE', #11899, #2616, #13199, .T. ) ;
#18639=CARTESIAN_POINT ( 'NONE',  ( -16.69495928710000143, -99.99921705949999762, 3.045998530109999880 ) ) ;
#18652=CARTESIAN_POINT ( 'NONE',  ( 16.71390024897803883, -100.0559847775274704, 4.300018913473477866 ) ) ;
#18653=CARTESIAN_POINT ( 'NONE',  ( 19.64032610941312740, -94.52419745022692155, 13.82579366131591847 ) ) ;
#18658=DIRECTION ( 'NONE',  ( 0.000000000000000000, -1.000000000000000000, 0.000000000000000000 ) ) ;
#18659=CARTESIAN_POINT ( 'NONE',  ( 1.731887814557739880, -94.79127258004355383, 24.69986651471424821 ) ) ;
#18660=TOROIDAL_SURFACE ( 'NONE', #6053, 29.91857981989999971, 10.00000000000000000 ) ;
#18667=CARTESIAN_POINT ( 'NONE',  ( -6.179359521840000369, -101.4254868690000109, 14.72527176150000017 ) ) ;
#18668=ORIENTED_EDGE ( 'NONE', *, *, #10462, .T. ) ;
#18672=CARTESIAN_POINT ( 'NONE',  ( -12.94585355959999973, -101.6484611540000031, -9.402386697720000797 ) ) ;
#18678=CARTESIAN_POINT ( 'NONE',  ( 16.79920482320000019, -99.53431242750001218, 4.586287493060000386 ) ) ;
#18682=CARTESIAN_POINT ( 'NONE',  ( 29.71503696804588657, -92.89593097428453916, 6.875073252006978386 ) ) ;
#18684=ORIENTED_EDGE ( 'NONE', *, *, #26258, .T. ) ;
#18703=CIRCLE ( 'NONE', #1050, 21.14285714289999873 ) ;
#18708=ORIENTED_EDGE ( 'NONE', *, *, #27969, .T. ) ;
#18717=FACE_OUTER_BOUND ( 'NONE', #1725, .T. ) ;
#18720=CONICAL_SURFACE ( 'NONE', #11294, 5.999999999999999112, 0.7853981633970000820 ) ;
#18727=CARTESIAN_POINT ( 'NONE',  ( 6.882913241140000693, -101.1292389600000092, 13.89502594439999861 ) ) ;
#18729=CARTESIAN_POINT ( 'NONE',  ( 7.588618361450000016, -101.1629257550000034, 13.79088284649999885 ) ) ;
#18730=CARTESIAN_POINT ( 'NONE',  ( -11.23282768690000033, -95.05242829889999712, -21.31919490279999962 ) ) ;
#18734=CARTESIAN_POINT ( 'NONE',  ( -7.639093477879999483, -98.53908914310000000, 17.11999108210000031 ) ) ;
#18736=CARTESIAN_POINT ( 'NONE',  ( -20.38264025652998512, -93.09721478938070049, -20.64447115935058719 ) ) ;
#18737=DIRECTION ( 'NONE',  ( 1.000000000000000000, 0.000000000000000000, 0.000000000000000000 ) ) ;
#18738=ORIENTED_EDGE ( 'NONE', *, *, #3723, .T. ) ;
#18745=EDGE_CURVE ( 'NONE', #6793, #25061, #3129, .T. ) ;
#18746=CARTESIAN_POINT ( 'NONE',  ( -0.1779554536940000098, -101.6484611540000031, -15.99901033990000165 ) ) ;
#18749=CARTESIAN_POINT ( 'NONE',  ( -11.76876591429999941, -94.80026553589999594, -21.40431208230000237 ) ) ;
#18752=CARTESIAN_POINT ( 'NONE',  ( 23.90217122411711159, -92.89593097429802526, -18.94561334467121938 ) ) ;
#18757=SURFACE_STYLE_FILL_AREA ( #3172 ) ;
#18758=ORIENTED_EDGE ( 'NONE', *, *, #3806, .F. ) ;
#18765=DIRECTION ( 'NONE',  ( 0.000000000000000000, 1.000000000000000000, 0.000000000000000000 ) ) ;
#18766=CARTESIAN_POINT ( 'NONE',  ( -0.7622684235660001084, -96.16784751140001219, 23.03987708760000075 ) ) ;
#18767=CARTESIAN_POINT ( 'NONE',  ( -0.7193305230537280215, -101.4628082233789002, -15.95725401771322005 ) ) ;
#18769=CARTESIAN_POINT ( 'NONE',  ( -3.841884380821040335, -98.73470582036235044, 18.09326313051193225 ) ) ;
#18770=AXIS2_PLACEMENT_3D ( 'NONE', #22625, #18400, #795 ) ;
#18772=CARTESIAN_POINT ( 'NONE',  ( -22.40618160359999678, -92.50425969839999141, -19.26308860609999840 ) ) ;
#18774=VERTEX_POINT ( 'NONE', #27340 ) ;
#18783=DIRECTION ( 'NONE',  ( 0.000000000000000000, 1.000000000000000000, 0.000000000000000000 ) ) ;
#18786=CARTESIAN_POINT ( 'NONE',  ( -15.92767415050000146, -101.0452850540000043, 3.185060022200000063 ) ) ;
#18792=CARTESIAN_POINT ( 'NONE',  ( 23.06813085299999955, -94.22763312370000222, -7.559806761219999949 ) ) ;
#18797=CARTESIAN_POINT ( 'NONE',  ( 15.85540327669583327, -101.1553309671668330, 4.123844213901046274 ) ) ;
#18803=CARTESIAN_POINT ( 'NONE',  ( 3.724765212310714446, -94.01599395605515497, 25.79154880062783306 ) ) ;
#18809=CARTESIAN_POINT ( 'NONE',  ( -5.884304964390000059, -101.1461874320000049, 15.04985543319999941 ) ) ;
#18812=CARTESIAN_POINT ( 'NONE',  ( -18.11577714932429828, -92.50000100535636705, -23.66412518367106088 ) ) ;
#18821=FACE_OUTER_BOUND ( 'NONE', #28059, .T. ) ;
#18824=CARTESIAN_POINT ( 'NONE',  ( 14.81927149150000034, -101.2530993010000060, 3.356308434120000239 ) ) ;
#18827=DIRECTION ( 'NONE',  ( 0.000000000000000000, 1.000000000000000000, 0.000000000000000000 ) ) ;
#18828=CARTESIAN_POINT ( 'NONE',  ( 11.40881661680000114, -94.59276292389999696, 20.88369873619999950 ) ) ;
#18830=DIRECTION ( 'NONE',  ( 1.000000000000000000, 0.000000000000000000, 0.000000000000000000 ) ) ;
#18831=DIRECTION ( 'NONE',  ( 0.000000000000000000, 1.000000000000000000, 0.000000000000000000 ) ) ;
#18837=VERTEX_POINT ( 'NONE', #20333 ) ;
#18844=EDGE_CURVE ( 'NONE', #3331, #21528, #9256, .T. ) ;
#18846=CARTESIAN_POINT ( 'NONE',  ( -7.878839520130000551, -100.4650220110000021, 14.87768963799999966 ) ) ;
#18853=CARTESIAN_POINT ( 'NONE',  ( -22.23129158500000102, -94.79581646409999962, -8.137667245660001214 ) ) ;
#18863=CARTESIAN_POINT ( 'NONE',  ( 11.94375585680425367, -101.6174239712916574, -10.68122429318817268 ) ) ;
#18864=CARTESIAN_POINT ( 'NONE',  ( 7.202169761539999548, -101.2530994060000040, 13.37848089600000101 ) ) ;
#18865=CARTESIAN_POINT ( 'NONE',  ( 16.01855245282755646, -96.92941831232313632, 15.11027898058047647 ) ) ;
#18872=CARTESIAN_POINT ( 'NONE',  ( 7.695130988680000783, -101.4135462429999990, 14.00070023930000040 ) ) ;
#18874=CARTESIAN_POINT ( 'NONE',  ( -11.49982146049999976, -94.92598208000001136, -21.36427486740000248 ) ) ;
#18877=CARTESIAN_POINT ( 'NONE',  ( 26.54817965250783018, -93.04141874247987687, -10.31287963464188451 ) ) ;
#18878=CARTESIAN_POINT ( 'NONE',  ( -20.59500362320578049, -93.08384138314025336, -20.57120710345400383 ) ) ;
#18879=EDGE_CURVE ( 'NONE', #10296, #20072, #14585, .T. ) ;
#18881=CARTESIAN_POINT ( 'NONE',  ( -1.283023294879999998, -111.0000000000000000, -16.20107482390000087 ) ) ;
#18883=VERTEX_POINT ( 'NONE', #6023 ) ;
#18885=ORIENTED_EDGE ( 'NONE', *, *, #12503, .T. ) ;
#18886=CARTESIAN_POINT ( 'NONE',  ( 0.5233167930302693449, -100.1585711159247722, -17.16730309748452399 ) ) ;
#18889=AXIS2_PLACEMENT_3D ( 'NONE', #2200, #11356, #18078 ) ;
#18890=CARTESIAN_POINT ( 'NONE',  ( 13.16431709405246764, -92.87422005961725802, 27.51274203059175605 ) ) ;
#18891=CARTESIAN_POINT ( 'NONE',  ( -13.24982249700000025, -93.87552273890000265, -20.99014450399999987 ) ) ;
#18894=CARTESIAN_POINT ( 'NONE',  ( -18.48852190589999722, -96.16769445330000110, 13.76947523039999943 ) ) ;
#18899=ORIENTED_EDGE ( 'NONE', *, *, #12805, .F. ) ;
#18905=FACE_OUTER_BOUND ( 'NONE', #19543, .T. ) ;
#18907=CARTESIAN_POINT ( 'NONE',  ( -0.6915678686394176600, -101.1604341566293925, -15.34138172876354389 ) ) ;
#18908=CARTESIAN_POINT ( 'NONE',  ( -11.23277242420000022, -95.05245081340000013, -21.31917440760000204 ) ) ;
#18912=CIRCLE ( 'NONE', #16086, 20.64285714289999873 ) ;
#18915=CARTESIAN_POINT ( 'NONE',  ( 26.33711340400000367, -92.75885938639999040, -7.868255112059999945 ) ) ;
#18916=APPLICATION_CONTEXT ( 'automotive_design' ) ;
#18918=ORIENTED_EDGE ( 'NONE', *, *, #28313, .T. ) ;
#18919=CARTESIAN_POINT ( 'NONE',  ( -14.80203930059999884, -101.0554840979999938, 4.588568860439999675 ) ) ;
#18920=CARTESIAN_POINT ( 'NONE',  ( -16.12855232609999945, -100.3665383609999964, 2.616550526240000174 ) ) ;
#18924=EDGE_CURVE ( 'NONE', #17438, #11909, #28127, .T. ) ;
#18928=CARTESIAN_POINT ( 'NONE',  ( 23.85918062689999886, -92.51331408429999215, -17.09634816450000017 ) ) ;
#18936=LINE ( 'NONE', #23578, #20872 ) ;
#18938=CARTESIAN_POINT ( 'NONE',  ( -18.22105428487606460, -98.38508418248619591, 5.014634119382404442 ) ) ;
#18939=EDGE_CURVE ( 'NONE', #17051, #21547, #4356, .T. ) ;
#18941=DIRECTION ( 'NONE',  ( 0.000000000000000000, 1.000000000000000000, 0.000000000000000000 ) ) ;
#18942=CARTESIAN_POINT ( 'NONE',  ( -5.973279726580000393, -101.5317765570000006, 14.93807730569999848 ) ) ;
#18944=CARTESIAN_POINT ( 'NONE',  ( 13.31770606849999972, -100.4792519539999915, -9.213118301410000655 ) ) ;
#18947=CARTESIAN_POINT ( 'NONE',  ( -13.15875165482993303, -101.5703832412493455, -9.204769674458903594 ) ) ;
#18953=EDGE_CURVE ( 'NONE', #19757, #22747, #21120, .T. ) ;
#18954=CARTESIAN_POINT ( 'NONE',  ( 14.82033914870000046, -101.2010924020000004, 3.644636806539999885 ) ) ;
#18955=ORIENTED_EDGE ( 'NONE', *, *, #8574, .F. ) ;
#18961=CARTESIAN_POINT ( 'NONE',  ( 6.054273664322402659, -92.50000267096280027, 29.18077564220382314 ) ) ;
#18963=EDGE_CURVE ( 'NONE', #24336, #22763, #1359, .T. ) ;
#18965=AXIS2_PLACEMENT_3D ( 'NONE', #4489, #15994, #6831 ) ;
#18974=CARTESIAN_POINT ( 'NONE',  ( -13.19529713839999907, -101.1659666750000071, -9.073059359340000185 ) ) ;
#18975=B_SPLINE_SURFACE_WITH_KNOTS ( 'NONE', 5, 5, ( 
 ( #28739, #13006, #24094, #8775, #15328, #19721, #4132, #25619, #21917 ),
 ( #1968, #16723, #5648, #14526, #10811, #24245, #8638, #19055, #15478 ),
 ( #6461, #4282, #21242, #13155, #10947, #26576, #23433, #17688, #16867 ),
 ( #1292, #1166, #18919, #3469, #10136, #25756, #12334, #7977, #14669 ),
 ( #23563, #11091, #7205, #374, #15776, #27167, #6770, #9217, #18124 ),
 ( #11401, #13447, #20455, #16072, #11253, #27312, #24974, #15631, #24529 ) ),
 .UNSPECIFIED., .F., .F., .F.,
 ( 6, 6 ),
 ( 6, 3, 6 ),
 ( 5.000411456039999258, 6.439463439139999856 ),
 ( 0.000000000000000000, 0.2500000000000000000, 0.5000000000000000000 ),
 .UNSPECIFIED. ) ;
#18978=CARTESIAN_POINT ( 'NONE',  ( 14.28941763439999946, -92.50000000000000000, -3.575252188409999921 ) ) ;
#18981=ORIENTED_EDGE ( 'NONE', *, *, #1308, .T. ) ;
#18986=DIRECTION ( 'NONE',  ( 1.000000000000000000, 0.000000000000000000, 0.000000000000000000 ) ) ;
#18993=EDGE_CURVE ( 'NONE', #19454, #15088, #25715, .T. ) ;
#18995=AXIS2_PLACEMENT_3D ( 'NONE', #11021, #4362, #9 ) ;
#18996=CARTESIAN_POINT ( 'NONE',  ( -0.02543935853460000188, -101.2530993010000060, -15.19457030269999898 ) ) ;
#18998=CARTESIAN_POINT ( 'NONE',  ( 15.52047986989999906, -100.9763228559999959, 2.247276725389999896 ) ) ;
#19000=CARTESIAN_POINT ( 'NONE',  ( 19.98296175649999995, -94.98812477599999227, 14.17692170039999944 ) ) ;
#19003=CARTESIAN_POINT ( 'NONE',  ( 6.775498823059999509, -101.2927714249999980, 14.55524442019999931 ) ) ;
#19006=CARTESIAN_POINT ( 'NONE',  ( -11.36607352380000080, -94.98911577330000000, -21.34235610950000250 ) ) ;
#19010=CARTESIAN_POINT ( 'NONE',  ( 25.00739163952697908, -93.86980009079698561, -5.047071168415053322 ) ) ;
#19011=DIRECTION ( 'NONE',  ( 0.000000000000000000, 1.000000000000000000, 0.000000000000000000 ) ) ;
#19015=ORIENTED_EDGE ( 'NONE', *, *, #19493, .F. ) ;
#19020=CARTESIAN_POINT ( 'NONE',  ( 0.4922916842733655596, -101.1553309671229357, -16.37551687936611344 ) ) ;
#19022=CARTESIAN_POINT ( 'NONE',  ( 13.75150794455260161, -92.56772982772069724, 27.22406583199860108 ) ) ;
#19026=EDGE_CURVE ( 'NONE', #25651, #8949, #23581, .T. ) ;
#19027=AXIS2_PLACEMENT_3D ( 'NONE', #28469, #15634, #22208 ) ;
#19037=CARTESIAN_POINT ( 'NONE',  ( -12.61948338259999858, -101.6484611540000031, -9.836088610590000059 ) ) ;
#19038=CIRCLE ( 'NONE', #13443, 20.64285714289999873 ) ;
#19039=CARTESIAN_POINT ( 'NONE',  ( -28.04810641310000108, -92.68289710869998999, 1.703742907849999932 ) ) ;
#19043=FACE_OUTER_BOUND ( 'NONE', #13719, .T. ) ;
#19049=DIRECTION ( 'NONE',  ( 1.000000000000000000, 0.000000000000000000, 0.000000000000000000 ) ) ;
#19053=CARTESIAN_POINT ( 'NONE',  ( -12.94585355959999973, -111.0000000000000000, -9.402386697720000797 ) ) ;
#19054=ORIENTED_EDGE ( 'NONE', *, *, #26039, .F. ) ;
#19055=CARTESIAN_POINT ( 'NONE',  ( -15.39251811099999934, -101.5369809019999963, 4.368436383219999719 ) ) ;
#19057=CARTESIAN_POINT ( 'NONE',  ( -16.75827440639999821, -100.1995464040000030, 3.211019438220000133 ) ) ;
#19059=VERTEX_POINT ( 'NONE', #7508 ) ;
#19060=DIRECTION ( 'NONE',  ( 0.000000000000000000, -1.000000000000000000, 0.000000000000000000 ) ) ;
#19064=CARTESIAN_POINT ( 'NONE',  ( -7.895689786979841251, -100.4166221067068960, 15.01891590590622627 ) ) ;
#19071=VERTEX_POINT ( 'NONE', #20302 ) ;
#19073=CARTESIAN_POINT ( 'NONE',  ( 7.059056192828962573, -100.0559847774587183, 15.74847134990731767 ) ) ;
#19075=VERTEX_POINT ( 'NONE', #16070 ) ;
#19080=CARTESIAN_POINT ( 'NONE',  ( -5.854053644989999583, -101.0685849509999912, 14.98984533339999992 ) ) ;
#19092=CARTESIAN_POINT ( 'NONE',  ( 1.375225265779999928, -94.98812079580000045, 24.46248543800000164 ) ) ;
#19093=CARTESIAN_POINT ( 'NONE',  ( 24.08726961439999670, -93.01125874769999768, -11.28467891660000078 ) ) ;
#19095=CARTESIAN_POINT ( 'NONE',  ( 29.75248106235870793, -92.74292563049040439, 6.711207100695092187 ) ) ;
#19097=ORIENTED_EDGE ( 'NONE', *, *, #17906, .F. ) ;
#19103=AXIS2_PLACEMENT_3D ( 'NONE', #23117, #1136, #25587 ) ;
#19107=B_SPLINE_CURVE_WITH_KNOTS ( 'NONE', 5,
 ( #4165, #28495, #8533, #17437, #26325, #6350, #15214, #24129, #13041 ),
 .UNSPECIFIED., .F., .F.,
 ( 6, 3, 6 ),
 ( 0.000000000000000000, 0.5000000000000000000, 1.000000000000000000 ),
 .UNSPECIFIED. ) ;
#19108=EDGE_LOOP ( 'NONE', ( #25263, #6673, #20093, #25617, #411 ) ) ;
#19113=VERTEX_POINT ( 'NONE', #24829 ) ;
#19114=CARTESIAN_POINT ( 'NONE',  ( -12.45166847509999997, -101.1411470200000053, -9.043467198420000130 ) ) ;
#19115=CARTESIAN_POINT ( 'NONE',  ( -18.06179280869999815, -92.68584241069999052, -23.36148935179999953 ) ) ;
#19116=CARTESIAN_POINT ( 'NONE',  ( -1.449827971759999778, -100.8733978449999995, -15.65780246259999764 ) ) ;
#19118=ORIENTED_EDGE ( 'NONE', *, *, #13450, .T. ) ;
#19120=CARTESIAN_POINT ( 'NONE',  ( 13.19211279289052641, -101.0610180772251709, -9.838472424427759933 ) ) ;
#19122=CARTESIAN_POINT ( 'NONE',  ( -25.71127254079999958, -93.01584738799999741, -6.102658843190000404 ) ) ;
#19123=CARTESIAN_POINT ( 'NONE',  ( 11.70579551850000044, -99.56347590750000620, -13.08273371679999997 ) ) ;
#19127=CARTESIAN_POINT ( 'NONE',  ( 11.38410404060000047, -101.1848541600000004, -10.19697977679999923 ) ) ;
#19129=CARTESIAN_POINT ( 'NONE',  ( -18.11956189529999861, -94.23919442010000580, 17.23487956379999630 ) ) ;
#19130=DIRECTION ( 'NONE',  ( 0.000000000000000000, 1.000000000000000000, 0.000000000000000000 ) ) ;
#19135=CARTESIAN_POINT ( 'NONE',  ( 15.81799604060000064, -101.3350617309999961, 2.549317426419999588 ) ) ;
#19138=CARTESIAN_POINT ( 'NONE',  ( 6.188549911610000009, -100.4808658609999981, 14.99463308189999999 ) ) ;
#19139=CARTESIAN_POINT ( 'NONE',  ( -13.09441083470000144, -92.84549618469999643, -23.96915825600000005 ) ) ;
#19141=CIRCLE ( 'NONE', #1479, 21.14285714289999873 ) ;
#19142=AXIS2_PLACEMENT_3D ( 'NONE', #21219, #1271, #10110 ) ;
#19143=CARTESIAN_POINT ( 'NONE',  ( -11.69298240589999871, -94.57749834670001121, -21.18608921030000047 ) ) ;
#19144=ADVANCED_FACE ( 'NONE', ( #17978 ), #373, .F. ) ;
#19146=CARTESIAN_POINT ( 'NONE',  ( 4.486712595243870005, -92.80045754838597816, -30.16820788345101434 ) ) ;
#19147=CARTESIAN_POINT ( 'NONE',  ( -7.446447301520000117, -98.65110728930000050, 17.10060481960000089 ) ) ;
#19149=CARTESIAN_POINT ( 'NONE',  ( 8.098514114769999495, -93.99830544889998407, -24.56325495060000108 ) ) ;
#19152=CARTESIAN_POINT ( 'NONE',  ( -6.580578580030000957, -111.0000000000000000, 15.40319725099999992 ) ) ;
#19155=CARTESIAN_POINT ( 'NONE',  ( -5.884304964390000059, -101.1461874320000049, 15.04985543319999941 ) ) ;
#19159=CARTESIAN_POINT ( 'NONE',  ( -0.8378492781409999646, -101.1292389529999980, -15.48430704140000103 ) ) ;
#19162=AXIS2_PLACEMENT_3D ( 'NONE', #12471, #28084, #24432 ) ;
#19165=CARTESIAN_POINT ( 'NONE',  ( -15.42268928922951865, -101.5369814700000148, 4.259183639765225848 ) ) ;
#19168=CARTESIAN_POINT ( 'NONE',  ( -12.61948338259999858, -101.1889999979999999, -9.836088610590000059 ) ) ;
#19172=CARTESIAN_POINT ( 'NONE',  ( -14.62235247615832456, -101.2530994837961487, 4.129102802680486128 ) ) ;
#19175=CARTESIAN_POINT ( 'NONE',  ( -29.57792341260000057, -92.63555401869999173, 6.374619421190000246 ) ) ;
#19178=EDGE_CURVE ( 'NONE', #11758, #17518, #21182, .T. ) ;
#19185=CARTESIAN_POINT ( 'NONE',  ( -7.593125501599999438, -94.98812477769999418, -22.45811160230000070 ) ) ;
#19186=CARTESIAN_POINT ( 'NONE',  ( -22.23129158500000102, -94.79581646409999962, -8.137667245660001214 ) ) ;
#19187=CARTESIAN_POINT ( 'NONE',  ( -15.35318355849999961, -101.1568446010000031, 3.495320071769999704 ) ) ;
#19190=CIRCLE ( 'NONE', #16871, 18.14285714289999873 ) ;
#19193=CARTESIAN_POINT ( 'NONE',  ( -12.47640054220000039, -101.1976625110000043, -10.56652411019999960 ) ) ;
#19196=CARTESIAN_POINT ( 'NONE',  ( -6.942134205095888078, -101.6297509123139662, 14.43170307226528593 ) ) ;
#19204=CARTESIAN_POINT ( 'NONE',  ( 6.817137268750544266, -100.4211561361777285, 15.53426013567950825 ) ) ;
#19206=ORIENTED_EDGE ( 'NONE', *, *, #11163, .F. ) ;
#19208=CARTESIAN_POINT ( 'NONE',  ( -17.32209284807034422, -99.34292914276410613, 3.453906795064102031 ) ) ;
#19209=AXIS2_PLACEMENT_3D ( 'NONE', #12357, #3632, #26207 ) ;
#19214=EDGE_CURVE ( 'NONE', #20556, #19071, #180, .T. ) ;
#19224=CARTESIAN_POINT ( 'NONE',  ( -22.23129207539999896, -94.79581469870001342, -8.137668203089999608 ) ) ;
#19225=CARTESIAN_POINT ( 'NONE',  ( 13.20150262729999824, -100.5717442099999914, -9.613817315349999504 ) ) ;
#19226=CARTESIAN_POINT ( 'NONE',  ( -20.41946551879999561, -93.96465009399999246, 14.25054530959999965 ) ) ;
#19227=CARTESIAN_POINT ( 'NONE',  ( 24.01103065379999890, -94.15497152590000951, -8.177649200119999406 ) ) ;
#19232=ORIENTED_EDGE ( 'NONE', *, *, #6843, .F. ) ;
#19234=FACE_OUTER_BOUND ( 'NONE', #27261, .T. ) ;
#19247=CARTESIAN_POINT ( 'NONE',  ( 19.57844007279999943, -94.59276583650000703, 13.52683266610000068 ) ) ;
#19250=CARTESIAN_POINT ( 'NONE',  ( 10.49903398999999915, -97.54012249449999672, 17.04265490439999908 ) ) ;
#19251=CARTESIAN_POINT ( 'NONE',  ( -15.08165013250000008, -92.59475633059999211, -24.08137820129999795 ) ) ;
#19252=CARTESIAN_POINT ( 'NONE',  ( -2.770815202149999656, -99.67742714719999242, -17.41576461069999837 ) ) ;
#19253=CARTESIAN_POINT ( 'NONE',  ( -7.593125501599999438, -94.98812477769999418, -22.45811160230000070 ) ) ;
#19256=DIRECTION ( 'NONE',  ( 1.000000000000000000, 0.000000000000000000, 0.000000000000000000 ) ) ;
#19258=CARTESIAN_POINT ( 'NONE',  ( 13.13687359478633532, -101.1248211535440760, -9.828810838103104075 ) ) ;
#19259=CARTESIAN_POINT ( 'NONE',  ( -27.33231135720000182, -92.65509162889999573, -4.521837785309999802 ) ) ;
#19261=CARTESIAN_POINT ( 'NONE',  ( -15.58411797090000128, -101.6484611620000038, 3.625951500279999795 ) ) ;
#19272=CIRCLE ( 'NONE', #22064, 21.14285714289999873 ) ;
#19273=CARTESIAN_POINT ( 'NONE',  ( -0.09996363298640001394, -101.1716782170000073, -15.73370943089999763 ) ) ;
#19275=CARTESIAN_POINT ( 'NONE',  ( 15.91666809940000071, -101.0685849509999912, 2.371725914449999806 ) ) ;
#19279=CARTESIAN_POINT ( 'NONE',  ( 6.166664293190000201, -100.8815367389999977, 14.41068211719999859 ) ) ;
#19280=CARTESIAN_POINT ( 'NONE',  ( 15.16640347679999934, -101.0151300849999814, 3.812177866399999893 ) ) ;
#19287=DIRECTION ( 'NONE',  ( 1.000000000000000000, 0.000000000000000000, 0.000000000000000000 ) ) ;
#19289=CARTESIAN_POINT ( 'NONE',  ( 6.330503061179999946, -92.97898997910000674, -25.99767272040000066 ) ) ;
#19294=CIRCLE ( 'NONE', #1171, 30.50000000000000000 ) ;
#19297=ORIENTED_EDGE ( 'NONE', *, *, #1831, .F. ) ;
#19299=CARTESIAN_POINT ( 'NONE',  ( -0.9785950990579999065, -101.1045726949999874, -15.50412976750000205 ) ) ;
#19301=CARTESIAN_POINT ( 'NONE',  ( -13.10652098802392373, -92.87497309988854965, -23.83816252673762293 ) ) ;
#19308=CARTESIAN_POINT ( 'NONE',  ( 23.84064839501263933, -94.60934249635550941, -7.609331551989225950 ) ) ;
#19310=ORIENTED_EDGE ( 'NONE', *, *, #2149, .T. ) ;
#19311=EDGE_CURVE ( 'NONE', #4465, #26488, #19398, .T. ) ;
#19313=CIRCLE ( 'NONE', #12316, 21.14285714289999873 ) ;
#19321=DIRECTION ( 'NONE',  ( 0.000000000000000000, 1.000000000000000000, 0.000000000000000000 ) ) ;
#19325=CARTESIAN_POINT ( 'NONE',  ( 15.51959124780000110, -100.8455998110000138, 4.065823162090000054 ) ) ;
#19328=CARTESIAN_POINT ( 'NONE',  ( -18.58472001550576991, -97.05288880472299695, -9.904339515219520607 ) ) ;
#19330=ORIENTED_EDGE ( 'NONE', *, *, #22180, .F. ) ;
#19332=CARTESIAN_POINT ( 'NONE',  ( -7.384731607069999981, -94.63960343449998902, -22.55849074379999664 ) ) ;
#19337=CARTESIAN_POINT ( 'NONE',  ( 19.90443298253104842, -98.49786007137258537, -0.8521435990548464900 ) ) ;
#19338=CARTESIAN_POINT ( 'NONE',  ( -12.48549849059999950, -101.5964542560000012, -10.07002115010000054 ) ) ;
#19340=CARTESIAN_POINT ( 'NONE',  ( 17.27104901786038837, -94.65677004888377155, 16.86278722961666077 ) ) ;
#19341=CARTESIAN_POINT ( 'NONE',  ( -7.233742488672582738, -101.4728631013542497, 14.42332162610310853 ) ) ;
#19342=ORIENTED_EDGE ( 'NONE', *, *, #17415, .F. ) ;
#19349=CARTESIAN_POINT ( 'NONE',  ( 6.802592131508781392, -100.4507315472249331, 15.51479369704953371 ) ) ;
#19352=EDGE_LOOP ( 'NONE', ( #21841, #19558, #9279, #4207 ) ) ;
#19362=CARTESIAN_POINT ( 'NONE',  ( -23.42541176010000115, -92.63555401869999173, -19.15044151010000206 ) ) ;
#19364=EDGE_LOOP ( 'NONE', ( #9612, #697, #25204, #23223 ) ) ;
#19366=CARTESIAN_POINT ( 'NONE',  ( 13.56595000559999953, -100.1785804069999983, -9.651294529659999455 ) ) ;
#19367=CARTESIAN_POINT ( 'NONE',  ( -19.58183770029999948, -93.00000000000000000, 20.70264511730000123 ) ) ;
#19368=CARTESIAN_POINT ( 'NONE',  ( 24.19872769330000040, -92.53610956480000027, -16.95184105959999954 ) ) ;
#19369=EDGE_CURVE ( 'NONE', #14137, #27440, #7657, .T. ) ;
#19373=EDGE_CURVE ( 'NONE', #15723, #9549, #17706, .T. ) ;
#19386=ORIENTED_EDGE ( 'NONE', *, *, #18345, .F. ) ;
#19387=CARTESIAN_POINT ( 'NONE',  ( 9.335817441729998833, -98.58684426249999433, 16.46450815360000064 ) ) ;
#19389=CARTESIAN_POINT ( 'NONE',  ( 1.908610474560000103, -93.01085527740001169, 27.31676936940000289 ) ) ;
#19393=CARTESIAN_POINT ( 'NONE',  ( 13.67589891821544867, -100.3266728693051704, -10.16527262647603891 ) ) ;
#19396=CARTESIAN_POINT ( 'NONE',  ( 9.374859430949999961, -94.98812769030000425, -22.63661719490000124 ) ) ;
#19397=ORIENTED_EDGE ( 'NONE', *, *, #25295, .T. ) ;
#19398=LINE ( 'NONE', #3957, #12254 ) ;
#19407=CARTESIAN_POINT ( 'NONE',  ( 0.1181328008709999905, -101.0956037589999994, -15.54443271709999941 ) ) ;
#19408=CARTESIAN_POINT ( 'NONE',  ( 26.97200738714188617, -92.55389105862651888, -12.40203756692639558 ) ) ;
#19414=CARTESIAN_POINT ( 'NONE',  ( 6.390608560400000471, -100.1785804069999983, 15.37343838830000031 ) ) ;
#19415=CARTESIAN_POINT ( 'NONE',  ( 15.58330902049999978, -101.3852859389999992, 3.598700821059999999 ) ) ;
#19420=CARTESIAN_POINT ( 'NONE',  ( 8.893989049490000909, -94.22485739640001157, -23.02234954029999869 ) ) ;
#19421=TOROIDAL_SURFACE ( 'NONE', #2684, 18.14285714289999873, 0.5000000000000000000 ) ;
#19428=CARTESIAN_POINT ( 'NONE',  ( -12.48293756425525913, -101.2021794472807130, -10.55357194642999907 ) ) ;
#19430=CARTESIAN_POINT ( 'NONE',  ( -1.179661616630000021, -101.0555477039999914, -15.45190212829999865 ) ) ;
#19432=CARTESIAN_POINT ( 'NONE',  ( 0.000000000000000000, -94.59276292389999696, 0.000000000000000000 ) ) ;
#19438=CARTESIAN_POINT ( 'NONE',  ( -14.64568814080000081, -101.2530993010000060, 4.044604232330000215 ) ) ;
#19443=CARTESIAN_POINT ( 'NONE',  ( 6.114061450890000415, -93.00000000000000000, -13.40104985119999981 ) ) ;
#19445=ORIENTED_EDGE ( 'NONE', *, *, #8998, .T. ) ;
#19449=CARTESIAN_POINT ( 'NONE',  ( -28.96583554960000129, -92.87863185420000889, 3.120909019039999954 ) ) ;
#19452=EDGE_CURVE ( 'NONE', #7443, #24926, #286, .T. ) ;
#19453=CARTESIAN_POINT ( 'NONE',  ( 15.53901966880000174, -100.4731125450000064, 4.587699026339999264 ) ) ;
#19454=VERTEX_POINT ( 'NONE', #22544 ) ;
#19458=CARTESIAN_POINT ( 'NONE',  ( 7.939780906490000234, -111.0000000000000000, 14.74863990870000130 ) ) ;
#19459=CIRCLE ( 'NONE', #17134, 30.50000000000000000 ) ;
#19466=CARTESIAN_POINT ( 'NONE',  ( -12.41979737689999830, -101.2927714249999980, -10.17404332349999940 ) ) ;
#19468=PLANE ( 'NONE',  #19162 ) ;
#19470=VECTOR ( 'NONE', #15752, 1000.000000000000000 ) ;
#19471=CARTESIAN_POINT ( 'NONE',  ( -1.022274391844619545, -101.5620304352384977, -16.03241640329728668 ) ) ;
#19477=AXIS2_PLACEMENT_3D ( 'NONE', #9969, #14490, #23251 ) ;
#19478=CARTESIAN_POINT ( 'NONE',  ( 11.44042105559999989, -101.2530993000000024, -9.998588429619998053 ) ) ;
#19479=ORIENTED_EDGE ( 'NONE', *, *, #18924, .F. ) ;
#19480=CARTESIAN_POINT ( 'NONE',  ( 5.798028723799999791E-12, -111.0000000000000000, -1.541933247750000003E-12 ) ) ;
#19484=CARTESIAN_POINT ( 'NONE',  ( 2.842132195609999634, -93.86302664969998943, 24.60248089030000074 ) ) ;
#19487=CARTESIAN_POINT ( 'NONE',  ( 0.3872056760440000245, -99.92967571559999840, -17.35614698070000017 ) ) ;
#19491=ORIENTED_EDGE ( 'NONE', *, *, #6512, .T. ) ;
#19493=EDGE_CURVE ( 'NONE', #4465, #18453, #14147, .T. ) ;
#19494=CARTESIAN_POINT ( 'NONE',  ( -20.44249130340000065, -92.65997669530000280, -20.57397485069999732 ) ) ;
#19499=AXIS2_PLACEMENT_3D ( 'NONE', #27128, #15593, #2070 ) ;
#19500=CARTESIAN_POINT ( 'NONE',  ( -22.29269750809999806, -94.98812477769999418, -8.065862959109999508 ) ) ;
#19501=CARTESIAN_POINT ( 'NONE',  ( 13.30722393669999981, -100.8088109309999965, -9.838500919220001251 ) ) ;
#19502=CARTESIAN_POINT ( 'NONE',  ( -18.69985100839999959, -92.84292036730001030, 22.78328762010000119 ) ) ;
#19508=DIRECTION ( 'NONE',  ( 0.4280775881279951789, 0.000000000000000000, 0.9037419867099893978 ) ) ;
#19511=CARTESIAN_POINT ( 'NONE',  ( 0.01062020221023751362, -92.80442066019506342, -30.50000543598749303 ) ) ;
#19512=( NAMED_UNIT ( * ) PLANE_ANGLE_UNIT ( ) SI_UNIT ( $, .RADIAN. ) );
#19516=VERTEX_POINT ( 'NONE', #12168 ) ;
#19522=CARTESIAN_POINT ( 'NONE',  ( 10.53835156000000062, -97.58469692710001198, 16.95036598099999736 ) ) ;
#19523=EDGE_CURVE ( 'NONE', #2955, #11758, #25315, .T. ) ;
#19526=VERTEX_POINT ( 'NONE', #27647 ) ;
#19527=CARTESIAN_POINT ( 'NONE',  ( 3.834560414579999854, -92.51556042380001088, 28.49273814280000039 ) ) ;
#19530=CARTESIAN_POINT ( 'NONE',  ( -29.48581804101084458, -92.50630337894774868, 7.800858964961374653 ) ) ;
#19533=CARTESIAN_POINT ( 'NONE',  ( 13.38876965537391150, -100.8061861237962376, -9.910527470073281719 ) ) ;
#19536=CARTESIAN_POINT ( 'NONE',  ( -16.03654356910000089, -101.2023582690000012, 3.165913905190000044 ) ) ;
#19542=CARTESIAN_POINT ( 'NONE',  ( 24.80237074776847805, -93.63284908648850546, -3.743708313212612104 ) ) ;
#19543=EDGE_LOOP ( 'NONE', ( #19638, #25054, #15886, #4927 ) ) ;
#19545=CARTESIAN_POINT ( 'NONE',  ( -0.04280064135489999866, -101.1848541609999899, -15.28253261989999956 ) ) ;
#19551=CARTESIAN_POINT ( 'NONE',  ( 6.997443162680000661, -100.0994409990000094, 15.73777937049999842 ) ) ;
#19552=CARTESIAN_POINT ( 'NONE',  ( 14.90889165870000177, -101.1848541609999899, 3.358955891889999990 ) ) ;
#19557=DIRECTION ( 'NONE',  ( 0.000000000000000000, 1.000000000000000000, 0.000000000000000000 ) ) ;
#19558=ORIENTED_EDGE ( 'NONE', *, *, #22780, .F. ) ;
#19559=AXIS2_PLACEMENT_3D ( 'NONE', #5412, #3101, #23191 ) ;
#19560=CARTESIAN_POINT ( 'NONE',  ( 1.834176908449999921, -92.53610956480000027, -29.48862716980000087 ) ) ;
#19565=CARTESIAN_POINT ( 'NONE',  ( -6.741828608569999659, -101.3256027139999986, 14.40730483740000167 ) ) ;
#19568=CARTESIAN_POINT ( 'NONE',  ( -12.47973093158265634, -101.2145573445022251, -10.54238648815402257 ) ) ;
#19572=CARTESIAN_POINT ( 'NONE',  ( 24.59449300740000055, -93.85307999839999127, -3.931206936640000205 ) ) ;
#19574=CARTESIAN_POINT ( 'NONE',  ( -0.9146590393339999459, -101.2995922080000071, -15.89573683670000115 ) ) ;
#19580=LINE ( 'NONE', #17547, #3452 ) ;
#19583=CARTESIAN_POINT ( 'NONE',  ( 23.54313657600000198, -94.98812477599999227, -6.784142512209999865 ) ) ;
#19584=DIRECTION ( 'NONE',  ( 0.000000000000000000, -1.000000000000000000, 0.000000000000000000 ) ) ;
#19591=B_SPLINE_CURVE_WITH_KNOTS ( 'NONE', 3,
 ( #11234, #20141, #17961, #2095, #351, #22046, #19837, #18110, #28717, #18254 ),
 .UNSPECIFIED., .F., .F.,
 ( 4, 2, 2, 2, 4 ),
 ( 0.000000000000000000, 0.2500000000000006106, 0.5000000000000012212, 0.7500000000000017764, 1.000000000000000000 ),
 .UNSPECIFIED. ) ;
#19593=CARTESIAN_POINT ( 'NONE',  ( -23.55553543979999986, -94.54719310899999130, -3.773174522320000168 ) ) ;
#19598=CARTESIAN_POINT ( 'NONE',  ( 15.16019776770000149, -100.8023006570000035, 4.366346884840000442 ) ) ;
#19600=CARTESIAN_POINT ( 'NONE',  ( 14.34373124439999891, -92.50000000000000000, 26.25602392650000283 ) ) ;
#19601=FACE_OUTER_BOUND ( 'NONE', #15801, .T. ) ;
#19602=ORIENTED_EDGE ( 'NONE', *, *, #13863, .T. ) ;
#19615=CARTESIAN_POINT ( 'NONE',  ( -12.31038953760000076, -100.5717442099999914, -10.73123778619999946 ) ) ;
#19620=CARTESIAN_POINT ( 'NONE',  ( -1.120268941615737646, -101.5019029709670377, -16.07166635754587958 ) ) ;
#19624=FACE_OUTER_BOUND ( 'NONE', #5397, .T. ) ;
#19625=CARTESIAN_POINT ( 'NONE',  ( -5.145393133449999823, -99.91547912669999221, 17.23229113919999733 ) ) ;
#19626=CARTESIAN_POINT ( 'NONE',  ( 12.02340861999999966, -92.49786325860000602, 27.16485054520000020 ) ) ;
#19628=CARTESIAN_POINT ( 'NONE',  ( -16.59215593114620191, -93.55106866339940552, -21.49707546704379624 ) ) ;
#19632=ORIENTED_EDGE ( 'NONE', *, *, #9769, .T. ) ;
#19636=CARTESIAN_POINT ( 'NONE',  ( -23.49132538869999820, -93.00000902169999506, -19.26888042029999681 ) ) ;
#19638=ORIENTED_EDGE ( 'NONE', *, *, #11507, .F. ) ;
#19639=CARTESIAN_POINT ( 'NONE',  ( -6.035167374697340215, -101.5620304352239600, 14.88825629219373603 ) ) ;
#19640=CARTESIAN_POINT ( 'NONE',  ( 12.82869130110000100, -100.7833805400000102, -9.414914349620000067 ) ) ;
#19641=CARTESIAN_POINT ( 'NONE',  ( -19.01557598040000130, -92.50000000000000000, 22.91712379000000155 ) ) ;
#19642=CARTESIAN_POINT ( 'NONE',  ( -5.574503815731460143, -98.30555344503575554, -19.38668258828887048 ) ) ;
#19644=CARTESIAN_POINT ( 'NONE',  ( 4.824585175810001050E-12, -111.0000000000000000, 3.574029960870000059E-12 ) ) ;
#19651=CARTESIAN_POINT ( 'NONE',  ( 0.07669151669536446170, -92.87422005960708304, -30.49990716389019241 ) ) ;
#19653=TOROIDAL_SURFACE ( 'NONE', #19209, 29.91857981989999971, 10.00000000000000000 ) ;
#19654=EDGE_CURVE ( 'NONE', #26053, #10170, #19272, .T. ) ;
#19659=CARTESIAN_POINT ( 'NONE',  ( 19.45476613419999978, -98.30614355080000166, -0.3720397164350000563 ) ) ;
#19664=DIRECTION ( 'NONE',  ( 0.000000000000000000, 1.000000000000000000, 0.000000000000000000 ) ) ;
#19667=CARTESIAN_POINT ( 'NONE',  ( -13.09441259049999928, -92.84550468730000716, -23.96917219330000037 ) ) ;
#19668=CARTESIAN_POINT ( 'NONE',  ( -8.799882794190001079, -96.11313168749998681, -20.83764462659999950 ) ) ;
#19670=CARTESIAN_POINT ( 'NONE',  ( 7.653117467020000397, -101.1929016639999901, 13.21760603179999904 ) ) ;
#19673=CARTESIAN_POINT ( 'NONE',  ( -29.60150005379874827, -92.56772982772959324, 7.348804374798064920 ) ) ;
#19675=ORIENTED_EDGE ( 'NONE', *, *, #9736, .T. ) ;
#19680=ORIENTED_EDGE ( 'NONE', *, *, #14950, .T. ) ;
#19683=CARTESIAN_POINT ( 'NONE',  ( -15.90615684040000133, -92.85195831059998284, 23.95936788750000090 ) ) ;
#19684=CARTESIAN_POINT ( 'NONE',  ( 23.70295537799999863, -94.59276292389999696, -2.111841813949999924 ) ) ;
#19687=CARTESIAN_POINT ( 'NONE',  ( 0.6048686566590000258, -100.8088109309999965, -16.53821160670000268 ) ) ;
#19695=FACE_OUTER_BOUND ( 'NONE', #15775, .T. ) ;
#19701=LINE ( 'NONE', #4697, #18366 ) ;
#19703=CARTESIAN_POINT ( 'NONE',  ( -5.679728865570000451, -96.65227117000000590, 20.49066625190000224 ) ) ;
#19706=CARTESIAN_POINT ( 'NONE',  ( 6.195449712719999447, -93.01125874769999768, -25.86806793289999717 ) ) ;
#19707=CARTESIAN_POINT ( 'NONE',  ( 6.825713544544626643, -101.5409490182170487, 14.56261500540370868 ) ) ;
#19708=FACE_OUTER_BOUND ( 'NONE', #9750, .T. ) ;
#19710=CARTESIAN_POINT ( 'NONE',  ( -13.02449431219020681, -100.2392017796373977, -11.09622749139835918 ) ) ;
#19714=CARTESIAN_POINT ( 'NONE',  ( -1.449832362199999780, -100.8733988930000010, -15.65780151839999945 ) ) ;
#19715=AXIS2_PLACEMENT_3D ( 'NONE', #7887, #10045, #18830 ) ;
#19718=CIRCLE ( 'NONE', #20686, 23.79684788999999867 ) ;
#19719=CARTESIAN_POINT ( 'NONE',  ( -20.85581432803203938, -92.82529299097140552, -22.25499991766502106 ) ) ;
#19721=CARTESIAN_POINT ( 'NONE',  ( -15.33274302080000062, -101.3256032150000010, 4.234343774090000068 ) ) ;
#19727=CARTESIAN_POINT ( 'NONE',  ( 24.59924222825820905, -93.48480241513080102, 11.95794408568441547 ) ) ;
#19731=EDGE_CURVE ( 'NONE', #25778, #24455, #19580, .T. ) ;
#19739=CARTESIAN_POINT ( 'NONE',  ( -21.63521261336145685, -95.36087494562657696, -8.478298660255941144 ) ) ;
#19741=ORIENTED_EDGE ( 'NONE', *, *, #5975, .F. ) ;
#19748=CARTESIAN_POINT ( 'NONE',  ( -15.07824091630000041, -101.1292389600000092, 3.618410085480000316 ) ) ;
#19750=CARTESIAN_POINT ( 'NONE',  ( -17.60046531049869145, -95.43638356959962721, 14.34842257852166192 ) ) ;
#19751=ORIENTED_EDGE ( 'NONE', *, *, #12896, .F. ) ;
#19753=LINE ( 'NONE', #28499, #25087 ) ;
#19754=CARTESIAN_POINT ( 'NONE',  ( -12.21977202059999890, -101.0678230150000019, -10.05267167180000065 ) ) ;
#19755=CARTESIAN_POINT ( 'NONE',  ( 6.888451955769999913, -99.53431386179998697, 15.99365555089999802 ) ) ;
#19757=VERTEX_POINT ( 'NONE', #26875 ) ;
#19763=EDGE_CURVE ( 'NONE', #19516, #5855, #19718, .T. ) ;
#19765=B_SPLINE_CURVE_WITH_KNOTS ( 'NONE', 5,
 ( #8149, #17760, #11010, #24456, #8565, #15397, #13366, #26500, #22269 ),
 .UNSPECIFIED., .F., .F.,
 ( 6, 3, 6 ),
 ( 0.000000000000000000, 0.5000000000000000000, 1.000000000000000000 ),
 .UNSPECIFIED. ) ;
#19771=CARTESIAN_POINT ( 'NONE',  ( 23.99168239580000161, -92.99570708089999016, 12.03585351179999918 ) ) ;
#19778=CARTESIAN_POINT ( 'NONE',  ( -18.94669760780000090, -93.16461275559998967, -21.17240009389999855 ) ) ;
#19782=CARTESIAN_POINT ( 'NONE',  ( 12.68262372769999935, -101.2927714249999980, -9.844469503889998307 ) ) ;
#19784=CARTESIAN_POINT ( 'NONE',  ( -11.73664924843507507, -94.54719627006902272, -20.76900799921979512 ) ) ;
#19790=EDGE_CURVE ( 'NONE', #8453, #25599, #28741, .T. ) ;
#19796=CARTESIAN_POINT ( 'NONE',  ( -0.4792089288136882064, -92.59055325466957242, -30.49623656381675119 ) ) ;
#19797=AXIS2_PLACEMENT_3D ( 'NONE', #28327, #17258, #6180 ) ;
#19799=VERTEX_POINT ( 'NONE', #4431 ) ;
#19800=CARTESIAN_POINT ( 'NONE',  ( -11.32307664120000013, -92.50000000000000000, 9.421136869679999748 ) ) ;
#19806=CARTESIAN_POINT ( 'NONE',  ( 15.04572477429999822, -95.61314413700000614, 17.10854321069999884 ) ) ;
#19810=CARTESIAN_POINT ( 'NONE',  ( -8.929965488379998817, -95.98352844290000974, -20.19091974539999867 ) ) ;
#19813=CARTESIAN_POINT ( 'NONE',  ( -29.52744277902158032, -92.52249206703173456, 7.640708811399515632 ) ) ;
#19814=CARTESIAN_POINT ( 'NONE',  ( 11.79516146510218455, -98.68740020586984940, -15.74753716043547591 ) ) ;
#19815=VERTEX_POINT ( 'NONE', #22285 ) ;
#19816=CARTESIAN_POINT ( 'NONE',  ( 7.292763125380000488, -92.50000467790000869, -29.01615471190000051 ) ) ;
#19819=CARTESIAN_POINT ( 'NONE',  ( 9.396869795909999823, -94.80026829410000744, -22.54657044670000232 ) ) ;
#19824=CARTESIAN_POINT ( 'NONE',  ( -13.52403886319999948, -92.76842119879999871, 27.15914155860000179 ) ) ;
#19828=CARTESIAN_POINT ( 'NONE',  ( 1.014918664000000081, -100.4731125450000064, -16.17028307509999863 ) ) ;
#19832=ORIENTED_EDGE ( 'NONE', *, *, #6406, .F. ) ;
#19835=VERTEX_POINT ( 'NONE', #20539 ) ;
#19837=CARTESIAN_POINT ( 'NONE',  ( 15.62053000518932855, -101.3051320416605563, 2.831994469588900110 ) ) ;
#19838=DIRECTION ( 'NONE',  ( 0.000000000000000000, -1.000000000000000000, 0.000000000000000000 ) ) ;
#19839=CARTESIAN_POINT ( 'NONE',  ( -18.00123211990801764, -98.93440139940453548, 5.015526314420251985 ) ) ;
#19842=CARTESIAN_POINT ( 'NONE',  ( -6.439729480049999566, -101.2530993010000060, 13.76171823350000167 ) ) ;
#19845=CARTESIAN_POINT ( 'NONE',  ( -12.49917433268771738, -101.1451610290395848, -10.60336746766995475 ) ) ;
#19847=CARTESIAN_POINT ( 'NONE',  ( 12.39757656149999931, -111.0000000000000000, -10.11435096289999969 ) ) ;
#19850=CARTESIAN_POINT ( 'NONE',  ( -0.6982943267950000310, -101.1292389600000092, -15.49059797790000026 ) ) ;
#19854=CARTESIAN_POINT ( 'NONE',  ( -20.47543134015453248, -92.69183043850887316, -22.60564142679350397 ) ) ;
#19866=CARTESIAN_POINT ( 'NONE',  ( 25.52931313223885823, -93.31462968146665560, 11.30597120268183531 ) ) ;
#19873=CARTESIAN_POINT ( 'NONE',  ( -12.94585355959999973, -101.1889999979999999, -9.402386697720000797 ) ) ;
#19875=DIRECTION ( 'NONE',  ( 0.4740167705367959727, 0.000000000000000000, 0.8805158154456209640 ) ) ;
#19877=CARTESIAN_POINT ( 'NONE',  ( 16.07378973510000009, -100.2511768809999921, 4.474534493000001056 ) ) ;
#19883=CARTESIAN_POINT ( 'NONE',  ( 7.409335217021491005, -92.49999999999998579, 29.58651093924895292 ) ) ;
#19886=B_SPLINE_CURVE_WITH_KNOTS ( 'NONE', 5,
 ( #16476, #8146, #27572, #23465, #17032, #12495, #7612, #10307, #25379 ),
 .UNSPECIFIED., .F., .F.,
 ( 6, 3, 6 ),
 ( 0.000000000000000000, 0.5000000000000000000, 1.000000000000000000 ),
 .UNSPECIFIED. ) ;
#19890=CARTESIAN_POINT ( 'NONE',  ( 24.83973459609999779, -92.98926436760000058, -13.74315515600000026 ) ) ;
#19895=CARTESIAN_POINT ( 'NONE',  ( -16.82739518109305266, -98.07939314455124702, 9.438034146772373845 ) ) ;
#19898=DIRECTION ( 'NONE',  ( 0.9999792992113792911, 0.000000000000000000, 0.006434372441722923698 ) ) ;
#19899=CARTESIAN_POINT ( 'NONE',  ( -12.54055638390000027, -100.2511768809999921, -11.00557226859999993 ) ) ;
#19902=VERTEX_POINT ( 'NONE', #27248 ) ;
#19905=ORIENTED_EDGE ( 'NONE', *, *, #26126, .T. ) ;
#19906=CARTESIAN_POINT ( 'NONE',  ( -5.298189715349999496, -100.9197081840000010, 14.69882786429999832 ) ) ;
#19908=EDGE_LOOP ( 'NONE', ( #16414, #17850, #18005, #5653 ) ) ;
#19910=CARTESIAN_POINT ( 'NONE',  ( -19.98504873792455072, -95.82120799309100789, 9.689515792764227697 ) ) ;
#19918=ORIENTED_EDGE ( 'NONE', *, *, #16687, .T. ) ;
#19922=CARTESIAN_POINT ( 'NONE',  ( -23.46882160569999698, -92.76843000840000286, -19.22844388999999765 ) ) ;
#19923=CARTESIAN_POINT ( 'NONE',  ( 7.635702898730000854, -101.6454117330000031, 14.06304778130000166 ) ) ;
#19926=DIRECTION ( 'NONE',  ( 0.000000000000000000, 1.000000000000000000, 0.000000000000000000 ) ) ;
#19929=CARTESIAN_POINT ( 'NONE',  ( -3.830277821634817226, -99.42096436988184394, -18.32509845586109876 ) ) ;
#19930=CARTESIAN_POINT ( 'NONE',  ( 8.125631349740000786, -101.1889999979999999, 24.17072847820000092 ) ) ;
#19937=CARTESIAN_POINT ( 'NONE',  ( -23.91929231898793162, -92.72059904819356291, -18.92399198549271588 ) ) ;
#19939=CARTESIAN_POINT ( 'NONE',  ( -0.02603423451098885524, -92.77521214511344283, -30.50001158162930892 ) ) ;
#19948=EDGE_LOOP ( 'NONE', ( #6401, #24035, #3737, #9853 ) ) ;
#19949=CARTESIAN_POINT ( 'NONE',  ( 15.09235194470000074, -95.70964358299998764, 17.10662658029999861 ) ) ;
#19956=CARTESIAN_POINT ( 'NONE',  ( -4.610939809759999619, -98.36043306160000554, -18.57959422089999890 ) ) ;
#19957=CARTESIAN_POINT ( 'NONE',  ( 5.787273401498926440, -93.40025063785100201, -27.00970585107326372 ) ) ;
#19959=CARTESIAN_POINT ( 'NONE',  ( -19.63026485099999618, -96.58392759020000540, 8.276969169350000044 ) ) ;
#19960=CARTESIAN_POINT ( 'NONE',  ( -29.71162786834675629, -92.72722989462940291, 6.889795938524829744 ) ) ;
#19962=EDGE_LOOP ( 'NONE', ( #8636, #12013, #4748, #17699 ) ) ;
#19969=B_SPLINE_CURVE_WITH_KNOTS ( 'NONE', 5,
 ( #28175, #22052, #21754, #15030, #2099, #28724 ),
 .UNSPECIFIED., .F., .F.,
 ( 6, 6 ),
 ( 0.000000000000000000, 1.000000000000000000 ),
 .UNSPECIFIED. ) ;
#19971=CARTESIAN_POINT ( 'NONE',  ( -13.55845395200000070, -92.92146065570000246, 27.19007895920000095 ) ) ;
#19975=CARTESIAN_POINT ( 'NONE',  ( 0.3686832740489999760, -101.0640712160000021, -16.09543371239999843 ) ) ;
#19979=AXIS2_PLACEMENT_3D ( 'NONE', #15498, #2418, #24408 ) ;
#19985=VERTEX_POINT ( 'NONE', #9153 ) ;
#19988=CARTESIAN_POINT ( 'NONE',  ( -4.317742246239999915, -95.94970068790001960, 22.11177757589999970 ) ) ;
#19991=CARTESIAN_POINT ( 'NONE',  ( 9.108757905360000962, -94.52419443349998573, -22.22442264740000084 ) ) ;
#19994=CARTESIAN_POINT ( 'NONE',  ( -7.243334595760000383, -101.4829589650000088, 14.41017875130000014 ) ) ;
#19997=CARTESIAN_POINT ( 'NONE',  ( -13.32816333360000094, -99.92967571559999840, -11.12411022969999941 ) ) ;
#19999=CIRCLE ( 'NONE', #22411, 0.4999999999999983347 ) ;
#20006=CARTESIAN_POINT ( 'NONE',  ( -20.84286287520331271, -92.82044061134170931, -22.26713171995569240 ) ) ;
#20007=VERTEX_POINT ( 'NONE', #22591 ) ;
#20016=CARTESIAN_POINT ( 'NONE',  ( 25.12718488642092396, -93.38554229052554945, 11.59376715993274942 ) ) ;
#20027=B_SPLINE_CURVE_WITH_KNOTS ( 'NONE', 5,
 ( #13566, #27283, #14012, #26992, #4978, #22621 ),
 .UNSPECIFIED., .F., .F.,
 ( 6, 6 ),
 ( 0.000000000000000000, 1.000000000000000000 ),
 .UNSPECIFIED. ) ;
#20029=CARTESIAN_POINT ( 'NONE',  ( -27.11354574210000123, -93.21603264559999502, -0.5572048120379999858 ) ) ;
#20032=CARTESIAN_POINT ( 'NONE',  ( -22.27191869549999836, -94.59276292389999696, -8.381623179300000004 ) ) ;
#20034=CARTESIAN_POINT ( 'NONE',  ( 16.77193911569999685, -99.58396362730000817, 4.490484942109999267 ) ) ;
#20035=ORIENTED_EDGE ( 'NONE', *, *, #19523, .F. ) ;
#20038=CARTESIAN_POINT ( 'NONE',  ( -13.21936810159999887, -100.9405345029999950, -8.915376394229999946 ) ) ;
#20047=CARTESIAN_POINT ( 'NONE',  ( 24.12141425730000321, -92.50732182800000203, -16.93547630009999949 ) ) ;
#20049=AXIS2_PLACEMENT_3D ( 'NONE', #11397, #16366, #2394 ) ;
#20052=CARTESIAN_POINT ( 'NONE',  ( -16.09526080732491948, -99.28256948951555216, 7.457957185716643345 ) ) ;
#20056=CARTESIAN_POINT ( 'NONE',  ( -12.64324746780000019, -99.97545561319999763, -11.21434624260000135 ) ) ;
#20058=DIRECTION ( 'NONE',  ( 0.000000000000000000, 1.000000000000000000, 0.000000000000000000 ) ) ;
#20060=ORIENTED_EDGE ( 'NONE', *, *, #18637, .T. ) ;
#20065=DIRECTION ( 'NONE',  ( 0.8775825618903722036, 0.000000000000000000, -0.4794255386042041156 ) ) ;
#20067=CARTESIAN_POINT ( 'NONE',  ( 12.04737265770000043, -101.6484611540000031, -10.52904611289999970 ) ) ;
#20072=VERTEX_POINT ( 'NONE', #20981 ) ;
#20073=CARTESIAN_POINT ( 'NONE',  ( -26.60615435977595311, -93.74885976973425272, -1.266735793207066862 ) ) ;
#20074=CARTESIAN_POINT ( 'NONE',  ( 21.43458377180000340, -94.34470043860000033, 13.67121948690000011 ) ) ;
#20081=CARTESIAN_POINT ( 'NONE',  ( -13.24613574540000016, -93.92589062410000622, -21.39339146240000034 ) ) ;
#20084=CARTESIAN_POINT ( 'NONE',  ( -6.191817604487320104, -101.6407018583229416, 14.75961303763012644 ) ) ;
#20085=CARTESIAN_POINT ( 'NONE',  ( 13.81100082510000071, -99.92967571559999840, -10.51865128849999920 ) ) ;
#20093=ORIENTED_EDGE ( 'NONE', *, *, #13481, .F. ) ;
#20094=CARTESIAN_POINT ( 'NONE',  ( -8.508623865889999749, -94.26884736950000843, -22.81720901600000317 ) ) ;
#20095=DIRECTION ( 'NONE',  ( 0.9037419867099890647, 0.000000000000000000, -0.4280775881279956785 ) ) ;
#20096=CYLINDRICAL_SURFACE ( 'NONE', #10326, 18.64285714290000939 ) ;
#20099=CARTESIAN_POINT ( 'NONE',  ( -14.65554054705737741, -101.0953223671037335, 4.722896106945597694 ) ) ;
#20104=EDGE_CURVE ( 'NONE', #24926, #20274, #11388, .T. ) ;
#20106=CARTESIAN_POINT ( 'NONE',  ( 21.34096039099999942, -97.41042626319999442, -2.228915448369999996 ) ) ;
#20111=CARTESIAN_POINT ( 'NONE',  ( 15.00024946600000142, -95.51664469100001043, 17.13920226819999826 ) ) ;
#20113=CARTESIAN_POINT ( 'NONE',  ( 7.773738738802946635, -93.98969193916553877, -24.92838943285665465 ) ) ;
#20116=CARTESIAN_POINT ( 'NONE',  ( -29.64623384722952082, -92.61393927536423121, 7.166097978304951432 ) ) ;
#20124=CARTESIAN_POINT ( 'NONE',  ( -15.24159474039999829, -92.86430477140000050, 25.11115096520000378 ) ) ;
#20129=CARTESIAN_POINT ( 'NONE',  ( 0.2072563983730000281, -101.2063419769999939, -15.98545391140000049 ) ) ;
#20134=EDGE_CURVE ( 'NONE', #22535, #19113, #10001, .T. ) ;
#20140=CARTESIAN_POINT ( 'NONE',  ( -14.34979093519999971, -92.51572464539999885, 25.42969430229999972 ) ) ;
#20141=CARTESIAN_POINT ( 'NONE',  ( 15.02247708185264941, -101.1962283502375470, 2.723567765951154129 ) ) ;
#20143=CARTESIAN_POINT ( 'NONE',  ( 17.21337473110000005, -95.77248627129999647, 14.26927196279999954 ) ) ;
#20146=CARTESIAN_POINT ( 'NONE',  ( 22.66360973360000131, -92.65509162899999751, 15.93308052109999906 ) ) ;
#20150=CARTESIAN_POINT ( 'NONE',  ( -12.47284051790895809, -101.5526869446301106, -10.13888011385641441 ) ) ;
#20155=EDGE_CURVE ( 'NONE', #1013, #27440, #15821, .T. ) ;
#20161=CARTESIAN_POINT ( 'NONE',  ( -18.85761467144973835, -98.17436949385547962, -7.631504019717256782 ) ) ;
#20169=EDGE_LOOP ( 'NONE', ( #18252, #27752, #23449, #20638 ) ) ;
#20170=CARTESIAN_POINT ( 'NONE',  ( 29.70835240799999966, -93.00000000000000000, 6.903897247299999762 ) ) ;
#20172=CARTESIAN_POINT ( 'NONE',  ( 7.933291312079999713, -100.9679265919999978, 13.53917068360000009 ) ) ;
#20175=ORIENTED_EDGE ( 'NONE', *, *, #19178, .F. ) ;
#20179=CARTESIAN_POINT ( 'NONE',  ( 25.07905384420000061, -92.81180274260000829, 10.93373002890000123 ) ) ;
#20181=VECTOR ( 'NONE', #14713, 1000.000000000000000 ) ;
#20184=AXIS2_PLACEMENT_3D ( 'NONE', #1437, #5917, #12748 ) ;
#20186=CARTESIAN_POINT ( 'NONE',  ( -15.70426946210000096, -100.0012764439999984, -8.839107909470000024 ) ) ;
#20191=ADVANCED_FACE ( 'NONE', ( #9254 ), #3291, .F. ) ;
#20196=CARTESIAN_POINT ( 'NONE',  ( 23.42162764450000267, -94.71481161159999829, -6.692249091959999063 ) ) ;
#20199=CARTESIAN_POINT ( 'NONE',  ( -17.54841868506949965, -95.98267023370895856, 13.27123176511321567 ) ) ;
#20203=EDGE_CURVE ( 'NONE', #20359, #16528, #15659, .T. ) ;
#20208=CARTESIAN_POINT ( 'NONE',  ( 26.16626699304385895, -92.92035259805699354, -15.67330046223513307 ) ) ;
#20213=CARTESIAN_POINT ( 'NONE',  ( 12.03366421969999855, -92.76454730689999906, 27.55075615510000020 ) ) ;
#20218=CARTESIAN_POINT ( 'NONE',  ( -27.15213039292447306, -93.55106866394891085, -0.4309374578557728097 ) ) ;
#20219=CARTESIAN_POINT ( 'NONE',  ( 20.57006820339999820, -94.36515600330000098, 13.91199895070000103 ) ) ;
#20222=DIRECTION ( 'NONE',  ( 1.000000000000000000, 0.000000000000000000, 0.000000000000000000 ) ) ;
#20227=CARTESIAN_POINT ( 'NONE',  ( -16.31262492385664231, -92.99999871998110734, -23.61087909523048012 ) ) ;
#20228=DIRECTION ( 'NONE',  ( 0.000000000000000000, 1.000000000000000000, 0.000000000000000000 ) ) ;
#20235=CARTESIAN_POINT ( 'NONE',  ( -7.548138925033555324, -97.11304554415646351, -20.42630931065637867 ) ) ;
#20237=CARTESIAN_POINT ( 'NONE',  ( 0.000000000000000000, -102.5000000000000000, 0.000000000000000000 ) ) ;
#20241=VERTEX_POINT ( 'NONE', #20332 ) ;
#20242=EDGE_CURVE ( 'NONE', #5855, #19985, #4439, .T. ) ;
#20243=CARTESIAN_POINT ( 'NONE',  ( -10.77550730630000153, -93.62972879769999679, -23.34803025570000301 ) ) ;
#20246=CARTESIAN_POINT ( 'NONE',  ( -24.25983842336477991, -92.54938211481912447, -18.48561634559768763 ) ) ;
#20253=CARTESIAN_POINT ( 'NONE',  ( 17.40083768629999739, -99.57131247590000100, 0.8327783396669999894 ) ) ;
#20254=ORIENTED_EDGE ( 'NONE', *, *, #6207, .F. ) ;
#20255=CARTESIAN_POINT ( 'NONE',  ( -13.46646228700000059, -101.1889999979999999, -9.098096927170001180 ) ) ;
#20259=CARTESIAN_POINT ( 'NONE',  ( 3.798704319269398333, -93.12686943395723915, -28.56536997530774613 ) ) ;
#20266=CARTESIAN_POINT ( 'NONE',  ( 7.003396616829999921, -92.68584525839999344, -28.68693272650000026 ) ) ;
#20269=CARTESIAN_POINT ( 'NONE',  ( -13.28370414271439870, -92.84927079009484885, 27.45529598729390841 ) ) ;
#20270=EDGE_LOOP ( 'NONE', ( #26710, #2288, #2931, #19054 ) ) ;
#20272=CARTESIAN_POINT ( 'NONE',  ( -17.14516425180000070, -93.38171818049998762, 19.21619453270000122 ) ) ;
#20274=VERTEX_POINT ( 'NONE', #8957 ) ;
#20276=CARTESIAN_POINT ( 'NONE',  ( -17.74113198119999879, -94.52293239269999958, 16.06143229570000130 ) ) ;
#20277=CARTESIAN_POINT ( 'NONE',  ( 0.4170640806890000274, -101.3090757639999993, -16.25756418510000145 ) ) ;
#20284=CARTESIAN_POINT ( 'NONE',  ( 27.70978180510000044, -92.50000000000000000, 12.74433177200000067 ) ) ;
#20286=CARTESIAN_POINT ( 'NONE',  ( 19.94074162929999972, -94.89420189139998740, 14.19047635519999950 ) ) ;
#20292=CARTESIAN_POINT ( 'NONE',  ( -7.122560077160000169, -101.2063419769999939, 14.31247113230000068 ) ) ;
#20296=CARTESIAN_POINT ( 'NONE',  ( 7.610177731959999470, -101.4231532209999926, 14.04048934709999941 ) ) ;
#20298=CARTESIAN_POINT ( 'NONE',  ( -0.6881950023909999548, -101.1848541609999899, -15.26655981750000102 ) ) ;
#20301=CARTESIAN_POINT ( 'NONE',  ( -7.498698696109999062, -94.79581469870001342, -22.45487717610000189 ) ) ;
#20302=CARTESIAN_POINT ( 'NONE',  ( -14.62247892739999955, -90.50000000000000000, -26.76626813769999913 ) ) ;
#20304=CARTESIAN_POINT ( 'NONE',  ( -7.120447010050000358, -101.1889999979999999, 15.21641332169999927 ) ) ;
#20305=CARTESIAN_POINT ( 'NONE',  ( 13.00155415721168772, -96.26579376197079796, 17.29370665404819718 ) ) ;
#20308=CARTESIAN_POINT ( 'NONE',  ( 24.01307781190000057, -93.00000000000000000, -18.61462211579999959 ) ) ;
#20311=ORIENTED_EDGE ( 'NONE', *, *, #25728, .F. ) ;
#20313=CARTESIAN_POINT ( 'NONE',  ( 7.790027027709999885, -101.0397073060000110, 13.52566268780000058 ) ) ;
#20319=CARTESIAN_POINT ( 'NONE',  ( 28.54521250490000028, -92.50425970539998843, 7.633765891700000417 ) ) ;
#20322=CARTESIAN_POINT ( 'NONE',  ( 16.25689483720000084, -99.97545561319999763, 4.618077352500000288 ) ) ;
#20326=CARTESIAN_POINT ( 'NONE',  ( -20.19463108470000279, -97.41042626780000546, -7.251312267670000367 ) ) ;
#20328=CARTESIAN_POINT ( 'NONE',  ( -30.48054257754459329, -92.53708507728566701, 1.089948664374644105 ) ) ;
#20329=EDGE_LOOP ( 'NONE', ( #878, #3529, #23070, #7855 ) ) ;
#20331=CARTESIAN_POINT ( 'NONE',  ( 0.000000000000000000, -90.50000000000000000, 0.000000000000000000 ) ) ;
#20332=CARTESIAN_POINT ( 'NONE',  ( -3.355978770230000130, -90.50000000000000000, -6.143077933229999843 ) ) ;
#20333=CARTESIAN_POINT ( 'NONE',  ( -7.333297298759998917, -94.59276292389999696, -22.63874378639999563 ) ) ;
#20336=ADVANCED_FACE ( 'NONE', ( #16834 ), #3163, .T. ) ;
#20339=FACE_OUTER_BOUND ( 'NONE', #2804, .T. ) ;
#20341=ORIENTED_EDGE ( 'NONE', *, *, #6545, .F. ) ;
#20343=B_SPLINE_CURVE_WITH_KNOTS ( 'NONE', 5,
 ( #17311, #19484, #17026, #17860, #8406, #24007, #6937, #26757, #26204 ),
 .UNSPECIFIED., .F., .F.,
 ( 6, 3, 6 ),
 ( 0.000000000000000000, 0.6992167742671963060, 1.000000000000000000 ),
 .UNSPECIFIED. ) ;
#20345=CARTESIAN_POINT ( 'NONE',  ( -3.183996595813977315, -98.12113812247983446, 20.16279650972818871 ) ) ;
#20346=CARTESIAN_POINT ( 'NONE',  ( -13.30220213780000016, -99.88067631459999518, -11.12664376240000053 ) ) ;
#20347=CARTESIAN_POINT ( 'NONE',  ( -12.41793182790000039, -101.2530993039999885, -8.757551688899999576 ) ) ;
#20351=CARTESIAN_POINT ( 'NONE',  ( 26.59508290546112264, -92.69183043814645373, -14.93184108318626357 ) ) ;
#20357=CARTESIAN_POINT ( 'NONE',  ( 1.563021348000000144, -94.54719592040000009, 23.80457129850000086 ) ) ;
#20358=CARTESIAN_POINT ( 'NONE',  ( 4.026022453159999515, -93.52727151969999397, 25.97757116140000022 ) ) ;
#20359=VERTEX_POINT ( 'NONE', #8083 ) ;
#20364=EDGE_CURVE ( 'NONE', #25380, #7420, #14843, .T. ) ;
#20368=TOROIDAL_SURFACE ( 'NONE', #6395, 15.50000000000000000, 0.5000000000000000000 ) ;
#20370=CARTESIAN_POINT ( 'NONE',  ( -11.85289062220000034, -94.98812477599999227, -21.44324726179999985 ) ) ;
#20373=CARTESIAN_POINT ( 'NONE',  ( -22.27191869549999836, -94.59276292389999696, -8.381623179300000004 ) ) ;
#20374=FACE_OUTER_BOUND ( 'NONE', #21718, .T. ) ;
#20380=CARTESIAN_POINT ( 'NONE',  ( 1.131980963049999955, -100.1275643909999928, -16.60892386949999988 ) ) ;
#20382=ORIENTED_EDGE ( 'NONE', *, *, #14568, .T. ) ;
#20383=DIRECTION ( 'NONE',  ( 0.000000000000000000, 1.000000000000000000, 0.000000000000000000 ) ) ;
#20386=CARTESIAN_POINT ( 'NONE',  ( 16.09612372445523931, -100.8061861225251477, 4.288648819865870543 ) ) ;
#20388=EDGE_LOOP ( 'NONE', ( #26420, #273, #11053, #19297 ) ) ;
#20396=CARTESIAN_POINT ( 'NONE',  ( 4.243840698532188149, -93.86127438317009819, 26.03392588043698908 ) ) ;
#20400=ORIENTED_EDGE ( 'NONE', *, *, #27187, .T. ) ;
#20405=ORIENTED_EDGE ( 'NONE', *, *, #13761, .F. ) ;
#20408=CARTESIAN_POINT ( 'NONE',  ( 3.331242539846007933, -93.08996811584388809, -28.87175727731148811 ) ) ;
#20409=CARTESIAN_POINT ( 'NONE',  ( -28.91420642530000151, -92.51331408429999215, 5.051166948289999681 ) ) ;
#20410=CARTESIAN_POINT ( 'NONE',  ( -17.97710455780000061, -98.83662759129998676, 4.969895303470000414 ) ) ;
#20411=CARTESIAN_POINT ( 'NONE',  ( 17.05053095294056575, -99.82487967928406647, 0.9399568373772333452 ) ) ;
#20413=ORIENTED_EDGE ( 'NONE', *, *, #1987, .F. ) ;
#20414=CIRCLE ( 'NONE', #3663, 20.64285714290000229 ) ;
#20415=CARTESIAN_POINT ( 'NONE',  ( 11.30811551740000098, -93.49005502370000897, -23.61965843710000001 ) ) ;
#20421=CARTESIAN_POINT ( 'NONE',  ( 7.312846564840000063, -92.50000000000000000, 29.61034067890000188 ) ) ;
#20422=VERTEX_POINT ( 'NONE', #12572 ) ;
#20423=CARTESIAN_POINT ( 'NONE',  ( -18.27191206690000058, -94.89419905399999777, 16.28310417119999798 ) ) ;
#20429=CARTESIAN_POINT ( 'NONE',  ( 8.125631349740000786, -92.50000000000000000, 24.17072847820000092 ) ) ;
#20435=EDGE_LOOP ( 'NONE', ( #9928, #21875, #8197, #1632 ) ) ;
#20439=CARTESIAN_POINT ( 'NONE',  ( 10.31391047600000022, -100.0012789650000116, 14.77758590519999871 ) ) ;
#20446=CARTESIAN_POINT ( 'NONE',  ( -12.45041691581901411, -101.4241070620317657, -10.32313517531819791 ) ) ;
#20448=FACE_OUTER_BOUND ( 'NONE', #26491, .T. ) ;
#20450=CARTESIAN_POINT ( 'NONE',  ( -0.7085401579220000912, -101.1716782170000073, -15.71788616779999970 ) ) ;
#20454=DIRECTION ( 'NONE',  ( 0.000000000000000000, -1.000000000000000000, 0.000000000000000000 ) ) ;
#20455=CARTESIAN_POINT ( 'NONE',  ( -14.94260916130000005, -100.8733989949999881, 4.897671729189999823 ) ) ;
#20460=DIRECTION ( 'NONE',  ( 0.000000000000000000, -1.000000000000000000, 0.000000000000000000 ) ) ;
#20462=DIRECTION ( 'NONE',  ( 1.000000000000000000, 0.000000000000000000, 0.000000000000000000 ) ) ;
#20463=DIRECTION ( 'NONE',  ( 1.000000000000000000, 0.000000000000000000, 0.000000000000000000 ) ) ;
#20465=ORIENTED_EDGE ( 'NONE', *, *, #25458, .F. ) ;
#20474=CARTESIAN_POINT ( 'NONE',  ( -19.93842487378145378, -95.91648618845204055, 9.502657547810732908 ) ) ;
#20477=AXIS2_PLACEMENT_3D ( 'NONE', #20901, #11851, #25129 ) ;
#20481=CARTESIAN_POINT ( 'NONE',  ( -21.69992076209999965, -95.77248565549999171, -5.387565530199999841 ) ) ;
#20483=CARTESIAN_POINT ( 'NONE',  ( 8.732396249151028300, -92.71525149955749612, 29.22337735326396313 ) ) ;
#20491=CARTESIAN_POINT ( 'NONE',  ( 14.12869155539999966, -98.65110728930000050, -12.17622016660000028 ) ) ;
#20492=ORIENTED_EDGE ( 'NONE', *, *, #20842, .F. ) ;
#20494=CARTESIAN_POINT ( 'NONE',  ( -4.178487457639150193, -99.07183862851897516, 18.71548091470333830 ) ) ;
#20495=CARTESIAN_POINT ( 'NONE',  ( 7.867248475934297325, -101.5674482532140956, 14.00205404261702569 ) ) ;
#20496=CARTESIAN_POINT ( 'NONE',  ( 0.000000000000000000, -101.1889999979999999, 0.000000000000000000 ) ) ;
#20501=CARTESIAN_POINT ( 'NONE',  ( 26.54754530181849859, -92.71525149907830610, -15.01627006387875696 ) ) ;
#20502=ORIENTED_EDGE ( 'NONE', *, *, #5663, .T. ) ;
#20506=CARTESIAN_POINT ( 'NONE',  ( 1.631254085230000150, -94.59276583650000703, 23.74088304550000217 ) ) ;
#20507=CARTESIAN_POINT ( 'NONE',  ( 10.51495134820000033, -92.53777738559999477, 27.19433521669999720 ) ) ;
#20508=ORIENTED_EDGE ( 'NONE', *, *, #18023, .F. ) ;
#20509=CARTESIAN_POINT ( 'NONE',  ( -5.298192075760000286, -100.9197081840000010, 14.69882727599999939 ) ) ;
#20511=CARTESIAN_POINT ( 'NONE',  ( -24.15516222759999820, -94.98812477599999227, -4.102682929219999330 ) ) ;
#20512=CARTESIAN_POINT ( 'NONE',  ( 3.787197165510000296, -111.0000000000000000, -30.26395773239999798 ) ) ;
#20514=ORIENTED_EDGE ( 'NONE', *, *, #7665, .F. ) ;
#20527=CARTESIAN_POINT ( 'NONE',  ( -16.86580049039999807, -99.83341253780000102, 3.169051538790000233 ) ) ;
#20530=ORIENTED_EDGE ( 'NONE', *, *, #3226, .T. ) ;
#20532=CARTESIAN_POINT ( 'NONE',  ( 0.7792231278100000269, -100.9137139110000021, -15.61347424839999931 ) ) ;
#20535=CARTESIAN_POINT ( 'NONE',  ( -10.63275893859999854, -93.28923078690000636, -23.66443698309999633 ) ) ;
#20538=CARTESIAN_POINT ( 'NONE',  ( 16.54913656973435110, -100.2392017793862209, 4.346239228624037665 ) ) ;
#20539=CARTESIAN_POINT ( 'NONE',  ( 2.876553231629999985, -108.5000000000000000, 5.265495371340000119 ) ) ;
#20543=DIRECTION ( 'NONE',  ( 0.000000000000000000, -1.000000000000000000, 0.000000000000000000 ) ) ;
#20544=VECTOR ( 'NONE', #7598, 1000.000000000000000 ) ;
#20550=CARTESIAN_POINT ( 'NONE',  ( 5.383412395290363861, -93.59823626961022569, 26.48305322804162643 ) ) ;
#20554=CARTESIAN_POINT ( 'NONE',  ( -18.80176912509999809, -92.50000000000000000, 23.77750384849999676 ) ) ;
#20556=VERTEX_POINT ( 'NONE', #15043 ) ;
#20558=CARTESIAN_POINT ( 'NONE',  ( -23.97049805334309269, -93.63284908740131129, -7.388380719408825570 ) ) ;
#20563=CARTESIAN_POINT ( 'NONE',  ( 6.744238910220000882, -101.2530993010000060, 13.61507422070000040 ) ) ;
#20566=CIRCLE ( 'NONE', #10293, 5.000000000000000888 ) ;
#20567=CARTESIAN_POINT ( 'NONE',  ( 12.26087422500000024, -93.85307999859999484, -21.67981636209999863 ) ) ;
#20570=CARTESIAN_POINT ( 'NONE',  ( 15.04861839279999991, -100.9137139110000021, 4.234011249179999936 ) ) ;
#20571=ORIENTED_EDGE ( 'NONE', *, *, #3500, .F. ) ;
#20576=EDGE_CURVE ( 'NONE', #24926, #22634, #1019, .T. ) ;
#20577=CARTESIAN_POINT ( 'NONE',  ( -17.83242922020000165, -95.72983087210000974, 13.58044602250000032 ) ) ;
#20585=AXIS2_PLACEMENT_3D ( 'NONE', #6600, #15458, #24369 ) ;
#20588=CARTESIAN_POINT ( 'NONE',  ( 6.296318341739999269, -102.8486084350000027, 11.52533341650000054 ) ) ;
#20591=CARTESIAN_POINT ( 'NONE',  ( 10.16789867219999977, -99.55619336450000390, 14.22101452250000087 ) ) ;
#20593=CARTESIAN_POINT ( 'NONE',  ( 23.34442203075309763, -92.53260370675270963, -19.62880660521832255 ) ) ;
#20594=CARTESIAN_POINT ( 'NONE',  ( 16.44117558850000194, -94.63960343439998724, 17.12038290500000315 ) ) ;
#20595=B_SPLINE_SURFACE_WITH_KNOTS ( 'NONE', 5, 5, ( 
 ( #652, #15760, #25112, #18112, #9199, #2378, #18407, #11529, #7490 ),
 ( #20439, #27445, #18255, #11678, #508, #22781, #20591, #20745, #2673 ),
 ( #24666, #9353, #27005, #801, #27151, #7190, #13875, #2819, #4699 ),
 ( #27296, #2972, #11236, #211, #16199, #13580, #5142, #15910, #24816 ),
 ( #14023, #22933, #24514, #11829, #9642, #4549, #18549, #4854, #20143 ),
 ( #9058, #20286, #353, #5429, #5703, #7902, #8036, #16352, #19247 ) ),
 .UNSPECIFIED., .F., .F., .F.,
 ( 6, 6 ),
 ( 6, 3, 6 ),
 ( 2.189016167100000132, 20.89370282910000043 ),
 ( 0.000000000000000000, 0.2500000000000000000, 0.5000000000000000000 ),
 .UNSPECIFIED. ) ;
#20596=CARTESIAN_POINT ( 'NONE',  ( 11.15108825559999950, -100.9197081840000010, -10.94438638200000113 ) ) ;
#20597=CARTESIAN_POINT ( 'NONE',  ( -7.473273236689999877, -100.7833805400000102, 14.04870527269999947 ) ) ;
#20599=CARTESIAN_POINT ( 'NONE',  ( -13.18688177930000016, -93.32822605769999313, -23.58441486170000090 ) ) ;
#20601=CARTESIAN_POINT ( 'NONE',  ( 7.358959778060000012, -101.1389411659999951, 13.51882459459999986 ) ) ;
#20604=AXIS2_PLACEMENT_3D ( 'NONE', #11120, #6199, #15066 ) ;
#20606=CARTESIAN_POINT ( 'NONE',  ( -2.080064695970000432, -97.58045781630001159, -19.90313438229999932 ) ) ;
#20607=ORIENTED_EDGE ( 'NONE', *, *, #13143, .T. ) ;
#20609=EDGE_CURVE ( 'NONE', #21973, #28309, #26559, .T. ) ;
#20610=CARTESIAN_POINT ( 'NONE',  ( 14.84965784370000108, -101.2530993010000060, 3.216001622850000352 ) ) ;
#20613=CARTESIAN_POINT ( 'NONE',  ( -16.86287214755321884, -99.33527508455092914, -8.386193468194429457 ) ) ;
#20616=B_SPLINE_CURVE_WITH_KNOTS ( 'NONE', 5,
 ( #22852, #25184, #724, #5361, #12040, #25465, #18908, #22998, #27667 ),
 .UNSPECIFIED., .F., .F.,
 ( 6, 3, 6 ),
 ( 0.000000000000000000, 0.4999899763738472891, 1.000000000000000000 ),
 .UNSPECIFIED. ) ;
#20618=ADVANCED_FACE ( 'NONE', ( #9213 ), #7025, .F. ) ;
#20620=CARTESIAN_POINT ( 'NONE',  ( 0.000000000000000000, -101.1889999979999999, 0.000000000000000000 ) ) ;
#20624=CARTESIAN_POINT ( 'NONE',  ( 6.997793179249999440, -101.3256027139999986, 14.28490435800000036 ) ) ;
#20626=FACE_OUTER_BOUND ( 'NONE', #8685, .T. ) ;
#20630=AXIS2_PLACEMENT_3D ( 'NONE', #12114, #16356, #23211 ) ;
#20633=DIRECTION ( 'NONE',  ( 0.000000000000000000, 1.000000000000000000, 0.000000000000000000 ) ) ;
#20634=CARTESIAN_POINT ( 'NONE',  ( -17.59047486835680019, -93.38817447856811782, -21.35100961780407403 ) ) ;
#20635=CARTESIAN_POINT ( 'NONE',  ( -16.86249289530055151, -97.53591929645045866, -10.88383259781367940 ) ) ;
#20638=ORIENTED_EDGE ( 'NONE', *, *, #7324, .F. ) ;
#20639=CARTESIAN_POINT ( 'NONE',  ( 8.099920077730001111, -100.8733989549999990, 13.47813240850000049 ) ) ;
#20640=CARTESIAN_POINT ( 'NONE',  ( -23.61875854070000003, -94.52293512109999085, -3.856443273130000016 ) ) ;
#20646=DIRECTION ( 'NONE',  ( 0.000000000000000000, 1.000000000000000000, 0.000000000000000000 ) ) ;
#20648=ADVANCED_FACE ( 'NONE', ( #13748 ), #7593, .T. ) ;
#20651=CARTESIAN_POINT ( 'NONE',  ( 23.91589042248623187, -92.93978723899958538, -18.92829633725156313 ) ) ;
#20658=CARTESIAN_POINT ( 'NONE',  ( 15.44884930899999986, -100.9728541479999961, 2.166274872270000262 ) ) ;
#20665=CARTESIAN_POINT ( 'NONE',  ( 4.226834115039999951, -93.34497626389999425, 25.39917024580000060 ) ) ;
#20668=CARTESIAN_POINT ( 'NONE',  ( -25.97364739661740174, -94.01603309698641908, -2.107898430554720370 ) ) ;
#20671=ORIENTED_EDGE ( 'NONE', *, *, #23007, .T. ) ;
#20674=DIRECTION ( 'NONE',  ( 1.000000000000000000, 0.000000000000000000, 0.000000000000000000 ) ) ;
#20677=FACE_OUTER_BOUND ( 'NONE', #20388, .T. ) ;
#20681=EDGE_CURVE ( 'NONE', #10004, #23975, #21442, .T. ) ;
#20683=CARTESIAN_POINT ( 'NONE',  ( -15.21470405170000006, -101.0782545459999966, 3.282628937979999773 ) ) ;
#20685=ORIENTED_EDGE ( 'NONE', *, *, #27219, .T. ) ;
#20686=AXIS2_PLACEMENT_3D ( 'NONE', #1822, #17838, #15782 ) ;
#20690=CARTESIAN_POINT ( 'NONE',  ( 23.55423057129999975, -93.65023913340000661, -9.043220619339999544 ) ) ;
#20692=FACE_OUTER_BOUND ( 'NONE', #4941, .T. ) ;
#20694=LINE ( 'NONE', #18058, #22247 ) ;
#20695=CARTESIAN_POINT ( 'NONE',  ( 15.65734951540625630, -101.5026031440680470, 3.803058839663215451 ) ) ;
#20699=STYLED_ITEM ( 'NONE', ( #25456 ), #25670 ) ;
#20703=DIRECTION ( 'NONE',  ( 0.000000000000000000, 1.000000000000000000, 0.000000000000000000 ) ) ;
#20704=CARTESIAN_POINT ( 'NONE',  ( 2.725557285477327341, -94.35872894872866823, 25.28257344816310948 ) ) ;
#20708=ORIENTED_EDGE ( 'NONE', *, *, #2251, .T. ) ;
#20711=B_SPLINE_CURVE_WITH_KNOTS ( 'NONE', 5,
 ( #10989, #8546, #17449, #20773, #3285, #7521 ),
 .UNSPECIFIED., .F., .F.,
 ( 6, 6 ),
 ( 0.000000000000000000, 1.000000000000000000 ),
 .UNSPECIFIED. ) ;
#20712=CARTESIAN_POINT ( 'NONE',  ( -6.085662280650000255, -101.5026188610000020, 14.82188091429999943 ) ) ;
#20713=ORIENTED_EDGE ( 'NONE', *, *, #24180, .T. ) ;
#20723=ADVANCED_FACE ( 'NONE', ( #27866 ), #358, .F. ) ;
#20729=CARTESIAN_POINT ( 'NONE',  ( -12.54588562670000051, -101.3256027139999986, -9.778723817850000444 ) ) ;
#20731=EDGE_LOOP ( 'NONE', ( #23997, #26434, #24076, #23678, #6257 ) ) ;
#20733=CIRCLE ( 'NONE', #16518, 5.499999999999998224 ) ;
#20745=CARTESIAN_POINT ( 'NONE',  ( 10.19815034219999994, -99.57131501109998339, 14.12374920210000084 ) ) ;
#20748=CARTESIAN_POINT ( 'NONE',  ( -17.08206735869999804, -92.57197946150000689, -23.65181049579999950 ) ) ;
#20750=DIRECTION ( 'NONE',  ( 0.000000000000000000, -1.000000000000000000, 0.000000000000000000 ) ) ;
#20752=EDGE_CURVE ( 'NONE', #25380, #9289, #6497, .T. ) ;
#20758=CARTESIAN_POINT ( 'NONE',  ( 11.83146454849999962, -101.1461869959999973, -11.00634589319999890 ) ) ;
#20761=CARTESIAN_POINT ( 'NONE',  ( 11.84697068120000019, -101.1716782170000073, -10.35390073449999981 ) ) ;
#20763=CARTESIAN_POINT ( 'NONE',  ( -17.97738387593933140, -98.68740020288944947, -7.995275462725576432 ) ) ;
#20768=CARTESIAN_POINT ( 'NONE',  ( 13.47882164853999676, -98.28141959653622450, 15.05059098890579961 ) ) ;
#20771=B_SPLINE_CURVE_WITH_KNOTS ( 'NONE', 3,
 ( #3548, #5859, #5310, #25697, #14606, #14471, #821, #16804, #14740, #3411, #25837, #3136, #12132, #9663, #27462, #28019, #9946, #7511, #20903, #21048, #7919, #23367, #23511, #23227, #12403, #16372, #18571, #25284, #23639, #1108 ),
 .UNSPECIFIED., .F., .F.,
 ( 4, 1, 1, 1, 1, 2, 2, 1, 1, 1, 1, 2, 2, 2, 1, 1, 1, 1, 2, 2, 4 ),
 ( 0.000000000000000000, 0.1250000000000265898, 0.1875000000000392464, 0.2187500000000447142, 0.2343750000000459632, 0.2421875000000486833, 0.2500000000000514033, 0.3750000000001049161, 0.4375000000001317280, 0.4687500000001439959, 0.4843750000001532663, 0.4921875000001595390, 0.5000000000001657563, 0.6250000000001812994, 0.6875000000001900702, 0.7187500000001965095, 0.7343750000001981748, 0.7421875000001975087, 0.7460937500001967315, 0.7500000000001958433, 1.000000000000000000 ),
 .UNSPECIFIED. ) ;
#20772=CARTESIAN_POINT ( 'NONE',  ( 6.830934818989999435, -101.1411470200000053, 13.79009341090000085 ) ) ;
#20773=CARTESIAN_POINT ( 'NONE',  ( -9.465086699151784799, -93.62676972709405732, -23.38439031276536539 ) ) ;
#20774=CARTESIAN_POINT ( 'NONE',  ( 7.661042932279999995, -101.3151549749999987, 13.94743070049999822 ) ) ;
#20781=CARTESIAN_POINT ( 'NONE',  ( 0.4184155325020000316, -93.00000902169999506, -30.38020818910000287 ) ) ;
#20785=CARTESIAN_POINT ( 'NONE',  ( 8.042004129799998680, -100.9405349759999950, 13.76814388520000065 ) ) ;
#20786=CARTESIAN_POINT ( 'NONE',  ( -20.41940881060000024, -94.07621218059999535, 14.28684394100000077 ) ) ;
#20787=ORIENTED_EDGE ( 'NONE', *, *, #4571, .T. ) ;
#20788=EDGE_CURVE ( 'NONE', #21750, #16528, #21772, .T. ) ;
#20789=CARTESIAN_POINT ( 'NONE',  ( 9.047106472501580399, -92.80045754867209951, 29.12732774022750704 ) ) ;
#20791=CARTESIAN_POINT ( 'NONE',  ( 0.4730157680896098227, -100.0559847773881330, -17.25169209895160805 ) ) ;
#20797=CARTESIAN_POINT ( 'NONE',  ( -16.70219504179999959, -100.0012196380000091, 6.767083061890000195 ) ) ;
#20800=CARTESIAN_POINT ( 'NONE',  ( 1.375225265779999928, -94.98812079580000045, 24.46248543800000164 ) ) ;
#20803=CARTESIAN_POINT ( 'NONE',  ( 15.94609587029999886, -101.3399913430000083, 2.448433415369999810 ) ) ;
#20804=VERTEX_POINT ( 'NONE', #4392 ) ;
#20805=ORIENTED_EDGE ( 'NONE', *, *, #7898, .T. ) ;
#20807=DIRECTION ( 'NONE',  ( -0.6685326369589543738, 0.000000000000000000, -0.7436828042389492799 ) ) ;
#20808=CARTESIAN_POINT ( 'NONE',  ( 1.436120303979999902, -94.52419051769999214, 23.97566470769999825 ) ) ;
#20816=ORIENTED_EDGE ( 'NONE', *, *, #397, .F. ) ;
#20817=CARTESIAN_POINT ( 'NONE',  ( -18.69985100839999959, -93.00000000000000000, 22.78328762010000119 ) ) ;
#20821=CARTESIAN_POINT ( 'NONE',  ( 0.2284267155709999997, -93.00000000000000000, -29.91770779450000362 ) ) ;
#20822=CARTESIAN_POINT ( 'NONE',  ( -15.74135051609999714, -100.8503292370000111, 3.071429158959999572 ) ) ;
#20831=ORIENTED_EDGE ( 'NONE', *, *, #11670, .T. ) ;
#20833=B_SPLINE_CURVE_WITH_KNOTS ( 'NONE', 3,
 ( #20511, #24446, #27222, #15540, #18332, #7262, #16127, #11755, #20668, #2305, #11155, #17893, #727, #20073, #15685, #20218, #289, #18034, #26932, #20958, #3459, #27365, #9576, #25186, #23421, #3050, #7706, #14246, #16858, #14102, #16571, #1015, #14389, #7409, #5362, #3322, #16426 ),
 .UNSPECIFIED., .F., .F.,
 ( 4, 2, 2, 1, 1, 1, 2, 2, 2, 2, 1, 1, 1, 2, 2, 2, 2, 1, 1, 1, 2, 2, 4 ),
 ( 0.000000000000000000, 0.1249999999999996114, 0.1875000000000000278, 0.2187500000000002220, 0.2343750000000005551, 0.2421875000000005551, 0.2460937500000005274, 0.2500000000000005551, 0.3749999999999905076, 0.4374999999999858447, 0.4687499999999831801, 0.4843749999999818479, 0.4921874999999809597, 0.4960937499999809597, 0.4999999999999809597, 0.6249999999999820144, 0.6874999999999825695, 0.7187499999999829026, 0.7343749999999827915, 0.7421874999999827915, 0.7460937499999830136, 0.7499999999999832356, 1.000000000000000000 ),
 .UNSPECIFIED. ) ;
#20837=CARTESIAN_POINT ( 'NONE',  ( 16.62650357984983174, -100.1517898586434114, 4.328685068564946725 ) ) ;
#20842=EDGE_CURVE ( 'NONE', #10004, #27670, #16197, .T. ) ;
#20844=CARTESIAN_POINT ( 'NONE',  ( 3.262018583601672184, -94.16479847359984490, 25.56489855335652805 ) ) ;
#20848=CIRCLE ( 'NONE', #1754, 0.8000000000000003775 ) ;
#20853=CARTESIAN_POINT ( 'NONE',  ( -5.676692421769999441, -101.1516803200000112, 14.23663479639999885 ) ) ;
#20854=ORIENTED_EDGE ( 'NONE', *, *, #26485, .F. ) ;
#20860=CARTESIAN_POINT ( 'NONE',  ( 0.3059185938709999553, -93.00000000000000000, 14.72672055670000013 ) ) ;
#20865=CARTESIAN_POINT ( 'NONE',  ( -20.61424083620000047, -93.67870248599999172, 14.15158961350000055 ) ) ;
#20872=VECTOR ( 'NONE', #27957, 1000.000000000000114 ) ;
#20873=CARTESIAN_POINT ( 'NONE',  ( -16.68089843889999813, -99.91542228490000355, 6.721411764870000027 ) ) ;
#20882=CARTESIAN_POINT ( 'NONE',  ( 7.609796875110000691, -99.12021627820000447, 16.26535001459999918 ) ) ;
#20883=EDGE_CURVE ( 'NONE', #1115, #18376, #8860, .T. ) ;
#20890=CARTESIAN_POINT ( 'NONE',  ( -11.31667057079999950, -95.23931402160000914, -21.36056405359999744 ) ) ;
#20891=AXIS2_PLACEMENT_3D ( 'NONE', #6695, #17615, #15556 ) ;
#20894=CARTESIAN_POINT ( 'NONE',  ( 7.540036301439999811, -101.3256028509999993, 14.00608922950000057 ) ) ;
#20897=CARTESIAN_POINT ( 'NONE',  ( -28.75283265410000055, -92.49999846069999876, -2.687056279340000131 ) ) ;
#20898=CARTESIAN_POINT ( 'NONE',  ( 11.40265797640000045, -97.01677120260001175, -17.81044358870000011 ) ) ;
#20899=ORIENTED_EDGE ( 'NONE', *, *, #1043, .F. ) ;
#20901=CARTESIAN_POINT ( 'NONE',  ( 0.000000000000000000, -92.50000000000000000, 0.000000000000000000 ) ) ;
#20903=CARTESIAN_POINT ( 'NONE',  ( -17.40319643073701883, -92.71525149976336877, 25.04774006126359964 ) ) ;
#20904=B_SPLINE_CURVE_WITH_KNOTS ( 'NONE', 3,
 ( #82, #17694, #13009, #17256, #6471, #8932 ),
 .UNSPECIFIED., .F., .F.,
 ( 4, 2, 4 ),
 ( 0.000000000000000000, 0.5000000000000000000, 1.000000000000000000 ),
 .UNSPECIFIED. ) ;
#20907=CARTESIAN_POINT ( 'NONE',  ( 11.98259099005113804, -101.6407018583229274, -10.61142287496397074 ) ) ;
#20909=CARTESIAN_POINT ( 'NONE',  ( 11.55429050816779224, -99.33527484956252351, 14.87222534504054039 ) ) ;
#20912=TOROIDAL_SURFACE ( 'NONE', #21813, 18.14285714289999873, 0.5000000000000000000 ) ;
#20915=DIRECTION ( 'NONE',  ( 0.000000000000000000, -1.000000000000000000, 0.000000000000000000 ) ) ;
#20917=CARTESIAN_POINT ( 'NONE',  ( -11.44999862350000086, -95.17624356449999823, -21.38312836629999936 ) ) ;
#20920=CARTESIAN_POINT ( 'NONE',  ( -7.539005773070000416, -98.58303758080000989, 17.10172281030000008 ) ) ;
#20921=CARTESIAN_POINT ( 'NONE',  ( 11.44042105559999989, -101.2530993000000024, -9.998588429619998053 ) ) ;
#20922=CARTESIAN_POINT ( 'NONE',  ( -0.1779554536940000098, -101.1889999979999999, -15.99901033990000165 ) ) ;
#20925=AXIS2_PLACEMENT_3D ( 'NONE', #23138, #3184, #5220 ) ;
#20933=CARTESIAN_POINT ( 'NONE',  ( -0.09292153041354569987, -101.6484611540000174, -15.99995616405717413 ) ) ;
#20938=CARTESIAN_POINT ( 'NONE',  ( 23.88061036455241748, -92.84927079009761997, -18.97278372083326659 ) ) ;
#20939=EDGE_CURVE ( 'NONE', #8616, #15112, #24193, .T. ) ;
#20947=ORIENTED_EDGE ( 'NONE', *, *, #27516, .F. ) ;
#20948=EDGE_CURVE ( 'NONE', #19815, #21547, #22858, .T. ) ;
#20954=CARTESIAN_POINT ( 'NONE',  ( 1.436102896439999999, -94.52419709919999491, 23.97566704719999819 ) ) ;
#20958=CARTESIAN_POINT ( 'NONE',  ( -27.62030561685637409, -93.40025063768234759, 0.3680505982496029005 ) ) ;
#20960=CARTESIAN_POINT ( 'NONE',  ( 5.115190889397799978, -93.00000166546709579, 28.53538671473107513 ) ) ;
#20970=DIRECTION ( 'NONE',  ( 0.000000000000000000, 1.000000000000000000, 0.000000000000000000 ) ) ;
#20971=CARTESIAN_POINT ( 'NONE',  ( -15.59466818890000006, -100.7754213330000113, 2.827888207719999603 ) ) ;
#20980=CARTESIAN_POINT ( 'NONE',  ( 15.70469996677716829, -101.4085864807012882, 3.915613578189586441 ) ) ;
#20981=CARTESIAN_POINT ( 'NONE',  ( 6.308882621499999566, -111.0000000000000000, -29.19167084780000110 ) ) ;
#20987=CARTESIAN_POINT ( 'NONE',  ( 5.988381294080164174, -93.48478527242041025, 26.68815097859544849 ) ) ;
#20994=CARTESIAN_POINT ( 'NONE',  ( -5.459548099580000091, -101.1364147039999892, 14.34189828759999941 ) ) ;
#21002=ORIENTED_EDGE ( 'NONE', *, *, #4915, .F. ) ;
#21008=ADVANCED_FACE ( 'NONE', ( #7618 ), #27601, .T. ) ;
#21025=ORIENTED_EDGE ( 'NONE', *, *, #19731, .F. ) ;
#21026=AXIS2_PLACEMENT_3D ( 'NONE', #25437, #16673, #9965 ) ;
#21042=DIRECTION ( 'NONE',  ( 0.000000000000000000, 1.000000000000000000, 0.000000000000000000 ) ) ;
#21043=CARTESIAN_POINT ( 'NONE',  ( 10.91527628520000093, -97.01506441390000646, -17.67900200189999893 ) ) ;
#21046=CARTESIAN_POINT ( 'NONE',  ( 11.51147269610000023, -101.1045726949999874, -10.43176325379999980 ) ) ;
#21048=CARTESIAN_POINT ( 'NONE',  ( -17.27650544376518482, -92.75430643285494625, 25.13513460670969124 ) ) ;
#21049=EDGE_CURVE ( 'NONE', #23834, #12597, #7955, .T. ) ;
#21051=VECTOR ( 'NONE', #24195, 1000.000000000000000 ) ;
#21052=DIRECTION ( 'NONE',  ( 0.000000000000000000, -1.000000000000000000, 0.000000000000000000 ) ) ;
#21054=CARTESIAN_POINT ( 'NONE',  ( 13.30637309069069119, -98.37418017201852649, 15.04202739120032639 ) ) ;
#21058=CARTESIAN_POINT ( 'NONE',  ( 13.74596177532710151, -96.89152198108462244, -16.22606708551202459 ) ) ;
#21059=CARTESIAN_POINT ( 'NONE',  ( 7.405704750090000843, -101.1273033739999931, 13.62605079230000094 ) ) ;
#21060=CARTESIAN_POINT ( 'NONE',  ( -11.33452548760000056, -94.90396370949999039, -21.28272403569999938 ) ) ;
#21063=CARTESIAN_POINT ( 'NONE',  ( -29.41500720700000215, -92.50000000000000000, 8.062713625770001613 ) ) ;
#21074=CARTESIAN_POINT ( 'NONE',  ( 0.4632353614598325175, -101.2111896145273988, -16.33269620291778423 ) ) ;
#21077=CARTESIAN_POINT ( 'NONE',  ( 13.20251034797960799, -92.82709422631791085, 27.49443084435448981 ) ) ;
#21079=DIRECTION ( 'NONE',  ( 0.000000000000000000, -1.000000000000000000, 0.000000000000000000 ) ) ;
#21080=EDGE_CURVE ( 'NONE', #19454, #8492, #23767, .T. ) ;
#21083=CARTESIAN_POINT ( 'NONE',  ( 12.94735060620000056, -94.70873613630000420, -19.84317021230000222 ) ) ;
#21085=CARTESIAN_POINT ( 'NONE',  ( -6.665307709260000379, -93.00000000000000000, -13.13558364449999871 ) ) ;
#21089=ORIENTED_EDGE ( 'NONE', *, *, #1151, .F. ) ;
#21090=CARTESIAN_POINT ( 'NONE',  ( 9.173959622430000849, -111.0000000000000000, -19.14607041020000011 ) ) ;
#21093=EDGE_LOOP ( 'NONE', ( #27234, #6805, #3484, #2074 ) ) ;
#21097=CARTESIAN_POINT ( 'NONE',  ( 9.396870180011182683, -94.80026864434297806, -22.54656979151466345 ) ) ;
#21100=AXIS2_PLACEMENT_3D ( 'NONE', #12377, #12516, #1344 ) ;
#21102=EDGE_CURVE ( 'NONE', #19985, #1588, #977, .T. ) ;
#21105=LINE ( 'NONE', #12328, #7625 ) ;
#21110=DIRECTION ( 'NONE',  ( -0.5423995371861327630, 0.000000000000000000, 0.8401206711302066088 ) ) ;
#21112=CARTESIAN_POINT ( 'NONE',  ( -15.74743825989999912, -100.6638977829999959, 2.772596425819999766 ) ) ;
#21118=CARTESIAN_POINT ( 'NONE',  ( 24.21290647080000369, -92.68283714880000446, -13.91082074250000034 ) ) ;
#21119=EDGE_LOOP ( 'NONE', ( #8586, #25792, #19330, #22959 ) ) ;
#21120=CIRCLE ( 'NONE', #23886, 0.8000000000000003775 ) ;
#21123=CARTESIAN_POINT ( 'NONE',  ( 19.58569043503641893, -94.54719627015504102, 13.61988836429140903 ) ) ;
#21128=ORIENTED_EDGE ( 'NONE', *, *, #81, .F. ) ;
#21130=CARTESIAN_POINT ( 'NONE',  ( -17.81659886998984987, -98.83160744532767694, 4.274644831898003261 ) ) ;
#21133=CARTESIAN_POINT ( 'NONE',  ( -5.832419616270000162, -101.1848541600000004, 14.12653895319999897 ) ) ;
#21138=AXIS2_PLACEMENT_3D ( 'NONE', #1552, #1688, #3999 ) ;
#21141=CARTESIAN_POINT ( 'NONE',  ( 23.48647081097517741, -94.80026864429605382, -6.710787388611177740 ) ) ;
#21148=CARTESIAN_POINT ( 'NONE',  ( 7.292753731799999528, -92.50000000000000000, -29.01615345709999971 ) ) ;
#21149=CARTESIAN_POINT ( 'NONE',  ( -20.22326673870000135, -94.79581125309999834, 12.30737463699999878 ) ) ;
#21153=CARTESIAN_POINT ( 'NONE',  ( 14.31067154247732098, -98.53908159006914502, -12.11011490584104600 ) ) ;
#21158=CARTESIAN_POINT ( 'NONE',  ( 19.51011835330500688, -98.16872834563331196, 2.367675478629094332 ) ) ;
#21167=AXIS2_PLACEMENT_3D ( 'NONE', #22658, #11554, #20463 ) ;
#21174=CARTESIAN_POINT ( 'NONE',  ( 7.466414723079999760, -101.1716783170000014, 13.84943005919999948 ) ) ;
#21178=PLANE ( 'NONE',  #3328 ) ;
#21182=LINE ( 'NONE', #28151, #11309 ) ;
#21183=CARTESIAN_POINT ( 'NONE',  ( 11.77685286379999852, -101.1716782080000030, -10.43412980439999949 ) ) ;
#21187=CARTESIAN_POINT ( 'NONE',  ( -7.879410208250000380, -101.1889999979999999, 15.46934584979999983 ) ) ;
#21194=CARTESIAN_POINT ( 'NONE',  ( 13.86691431120587126, -97.38870237776961858, -15.27021487312774717 ) ) ;
#21201=DIRECTION ( 'NONE',  ( 0.000000000000000000, 1.000000000000000000, 0.000000000000000000 ) ) ;
#21202=EDGE_CURVE ( 'NONE', #22268, #1488, #12598, .T. ) ;
#21207=CARTESIAN_POINT ( 'NONE',  ( -17.00715350810000004, -99.92967601899998442, 3.484608414699999823 ) ) ;
#21210=VERTEX_POINT ( 'NONE', #17405 ) ;
#21211=CARTESIAN_POINT ( 'NONE',  ( 0.2236201771617485901, -101.5026031439579839, -16.11104727832875483 ) ) ;
#21215=CARTESIAN_POINT ( 'NONE',  ( -13.16778131023122000, -93.19477818465753671, -23.58326779864327705 ) ) ;
#21218=CARTESIAN_POINT ( 'NONE',  ( 11.15108825559999950, -100.9197081840000010, -10.94438638200000113 ) ) ;
#21219=CARTESIAN_POINT ( 'NONE',  ( 13.01745538959999848, -101.1889999979999999, -10.62006851110000127 ) ) ;
#21224=EDGE_CURVE ( 'NONE', #11679, #21931, #3024, .T. ) ;
#21227=CARTESIAN_POINT ( 'NONE',  ( -28.30453570960000320, -92.90721294769998906, 1.613063908820000059 ) ) ;
#21228=CARTESIAN_POINT ( 'NONE',  ( 8.831064126840001194, -94.59276292389999696, -22.09756266850000017 ) ) ;
#21230=EDGE_CURVE ( 'NONE', #7597, #5628, #25952, .T. ) ;
#21239=CARTESIAN_POINT ( 'NONE',  ( 24.58039951800000011, -93.96464232159999597, -3.979621713999999866 ) ) ;
#21240=CARTESIAN_POINT ( 'NONE',  ( -7.593125501599999438, -94.98812477769999418, -22.45811160230000070 ) ) ;
#21242=CARTESIAN_POINT ( 'NONE',  ( -14.77962994559999999, -101.1130182370000057, 4.416924883319999218 ) ) ;
#21243=CARTESIAN_POINT ( 'NONE',  ( -15.53707292570000043, -101.0215274990000012, 3.216537776050000019 ) ) ;
#21246=B_SPLINE_SURFACE_WITH_KNOTS ( 'NONE', 5, 5, ( 
 ( #14008, #2953, #11816, #20729, #788, #5274, #14161, #8386, #28355 ),
 ( #3749, #14940, #17145, #22105, #12612, #26470, #17293, #10421, #21802 ),
 ( #23846, #28082, #15217, #14805, #24281, #24132, #4168, #13195, #23990 ),
 ( #19338, #1858, #6061, #23705, #13045, #10550, #21956, #2004, #8536 ),
 ( #26182, #10845, #19466, #28640, #19754, #6213, #12886, #17582, #1580 ),
 ( #8249, #8118, #21523, #6506, #28214, #26033, #15367, #17441, #4322 ),
 ( #19193, #17007, #3887, #10284, #6354, #25896, #15082, #5921, #28500 ),
 ( #1712, #12752, #21664, #4025, #19615, #26328, #15670, #13335, #24573 ),
 ( #6657, #276, #22397, #6957, #19899, #26777, #15520, #4613, #8817 ),
 ( #13488, #11297, #18019, #2443, #15819, #20056, #11137, #13937, #9118 ),
 ( #7247, #26917, #24731, #4766, #2593, #24430, #13641, #8971, #2145 ),
 ( #22549, #20346, #415, #9265, #4468, #7106, #22688, #15968, #18319 ) ),
 .UNSPECIFIED., .F., .F., .F.,
 ( 6, 3, 3, 6 ),
 ( 6, 3, 6 ),
 ( 3.852920539469999905, 4.834764074420000668, 6.134713715050000182, 8.383984506250000024 ),
 ( 0.000000000000000000, 0.2500000000000000000, 0.5000000000000000000 ),
 .UNSPECIFIED. ) ;
#21258=CARTESIAN_POINT ( 'NONE',  ( 6.729516044911419748, -100.6338045028395953, 15.38746398300566298 ) ) ;
#21263=CARTESIAN_POINT ( 'NONE',  ( 27.47009838660000014, -93.04780275979999260, 9.761662582170000491 ) ) ;
#21264=CARTESIAN_POINT ( 'NONE',  ( -5.991572043530000613, -101.1499348409999897, 14.56695843900000042 ) ) ;
#21265=ORIENTED_EDGE ( 'NONE', *, *, #25295, .F. ) ;
#21268=B_SPLINE_CURVE_WITH_KNOTS ( 'NONE', 3,
 ( #24899, #20227, #4930, #24754 ),
 .UNSPECIFIED., .F., .F.,
 ( 4, 4 ),
 ( 0.000000000000000000, 1.000000000000000000 ),
 .UNSPECIFIED. ) ;
#21275=CARTESIAN_POINT ( 'NONE',  ( -20.31500103569999993, -92.75885976620000406, 18.51637639279999803 ) ) ;
#21276=CARTESIAN_POINT ( 'NONE',  ( 24.26460669609999954, -92.67327634539999792, -13.69605124519999961 ) ) ;
#21277=ORIENTED_EDGE ( 'NONE', *, *, #7324, .T. ) ;
#21284=FACE_OUTER_BOUND ( 'NONE', #4823, .T. ) ;
#21286=EDGE_CURVE ( 'NONE', #28264, #3937, #20771, .T. ) ;
#21293=ORIENTED_EDGE ( 'NONE', *, *, #25177, .T. ) ;
#21299=CARTESIAN_POINT ( 'NONE',  ( -12.57997069900000042, -101.2141467319999890, -8.613800160570001196 ) ) ;
#21302=CARTESIAN_POINT ( 'NONE',  ( -3.134349037060000231, -94.63960343439998724, 23.52861282910000185 ) ) ;
#21304=DIRECTION ( 'NONE',  ( 1.000000000000000000, 0.000000000000000000, 0.000000000000000000 ) ) ;
#21305=ORIENTED_EDGE ( 'NONE', *, *, #17702, .T. ) ;
#21306=AXIS2_PLACEMENT_3D ( 'NONE', #17594, #26483, #15379 ) ;
#21307=CARTESIAN_POINT ( 'NONE',  ( 13.27284362584146216, -100.9609609850291747, -9.861926373179022320 ) ) ;
#21309=CARTESIAN_POINT ( 'NONE',  ( 12.03933649750000079, -99.75094652210000845, -13.19595464940000085 ) ) ;
#21310=ORIENTED_EDGE ( 'NONE', *, *, #21102, .F. ) ;
#21316=ORIENTED_EDGE ( 'NONE', *, *, #4317, .T. ) ;
#21318=CARTESIAN_POINT ( 'NONE',  ( -0.1050716136000000023, -101.4254868729999970, -15.96877589609999681 ) ) ;
#21320=CARTESIAN_POINT ( 'NONE',  ( 15.25351091960000005, -101.0848057460000007, 2.208595176079999778 ) ) ;
#21325=CARTESIAN_POINT ( 'NONE',  ( 6.723571926760000039, -99.77922884479998800, 15.77121833869999890 ) ) ;
#21326=CARTESIAN_POINT ( 'NONE',  ( 15.37735894870000131, -101.1716782170000073, 3.330286249999999892 ) ) ;
#21329=CARTESIAN_POINT ( 'NONE',  ( -11.53977386519999904, -95.01967132979999064, -21.39764275870000176 ) ) ;
#21331=CARTESIAN_POINT ( 'NONE',  ( 5.625522035772098306, -92.55017404143156057, -29.97671659717093817 ) ) ;
#21334=CARTESIAN_POINT ( 'NONE',  ( -8.107793959220000346, -99.57787118740000665, 15.34802496579999875 ) ) ;
#21336=CARTESIAN_POINT ( 'NONE',  ( 0.2284307630869999717, -92.50000942380000879, -29.91770856260000144 ) ) ;
#21339=CARTESIAN_POINT ( 'NONE',  ( -5.750261582500000301, -100.9405348700000076, 14.87178911969999895 ) ) ;
#21343=CARTESIAN_POINT ( 'NONE',  ( 0.5497266010686944204, -101.0147714271427617, -16.48405362120961470 ) ) ;
#21349=VECTOR ( 'NONE', #15316, 1000.000000000000000 ) ;
#21353=CARTESIAN_POINT ( 'NONE',  ( 24.31603054292643051, -94.01603309709156520, -9.370392387943658363 ) ) ;
#21355=ORIENTED_EDGE ( 'NONE', *, *, #7780, .F. ) ;
#21356=ADVANCED_FACE ( 'NONE', ( #18717 ), #3785, .F. ) ;
#21359=EDGE_CURVE ( 'NONE', #9504, #11556, #12275, .T. ) ;
#21361=AXIS2_PLACEMENT_3D ( 'NONE', #22326, #2373, #11228 ) ;
#21371=ORIENTED_EDGE ( 'NONE', *, *, #13509, .T. ) ;
#21373=CARTESIAN_POINT ( 'NONE',  ( -6.285925807789999986, -111.0000000000000000, 14.71350185169999847 ) ) ;
#21374=CARTESIAN_POINT ( 'NONE',  ( -22.22671645450000000, -94.70873790529999781, -8.207211804499998209 ) ) ;
#21375=CARTESIAN_POINT ( 'NONE',  ( -15.58411797090000128, -101.6484611620000038, 3.625951500279999795 ) ) ;
#21379=CARTESIAN_POINT ( 'NONE',  ( 20.30130924245990087, -98.17436949284241621, -1.306264829020119755 ) ) ;
#21382=CARTESIAN_POINT ( 'NONE',  ( -7.894758065967145022, -100.4211561361303922, 15.01530531104792310 ) ) ;
#21384=CIRCLE ( 'NONE', #2316, 29.91857981989999971 ) ;
#21387=EDGE_CURVE ( 'NONE', #1710, #22634, #7850, .T. ) ;
#21388=DIRECTION ( 'NONE',  ( 0.07620182022913774000, 0.000000000000000000, 0.9970924142694930215 ) ) ;
#21392=EDGE_CURVE ( 'NONE', #22268, #21973, #5640, .T. ) ;
#21394=CARTESIAN_POINT ( 'NONE',  ( 6.693983694146544039, -100.7538407678108854, 15.29886744127561471 ) ) ;
#21399=CARTESIAN_POINT ( 'NONE',  ( 29.51280632209999766, -92.84292833370000153, 7.159272379339999937 ) ) ;
#21403=CARTESIAN_POINT ( 'NONE',  ( 11.77298154309999845, -101.2530993010000060, -9.604785791470000333 ) ) ;
#21405=VECTOR ( 'NONE', #21857, 1000.000000000000000 ) ;
#21413=CARTESIAN_POINT ( 'NONE',  ( 18.35308676840000075, -98.83667233820000320, 3.322316128729999818 ) ) ;
#21414=CARTESIAN_POINT ( 'NONE',  ( -20.34964369559999753, -94.63959812639998859, 12.21932103440000006 ) ) ;
#21415=CARTESIAN_POINT ( 'NONE',  ( 23.64032483880000157, -93.61368346399999041, -9.011411803559999711 ) ) ;
#21417=DIRECTION ( 'NONE',  ( 1.000000000000000000, 0.000000000000000000, 0.000000000000000000 ) ) ;
#21421=EDGE_CURVE ( 'NONE', #9768, #26053, #26943, .T. ) ;
#21422=DIRECTION ( 'NONE',  ( 0.000000000000000000, 1.000000000000000000, 0.000000000000000000 ) ) ;
#21423=CARTESIAN_POINT ( 'NONE',  ( 20.52188441893875392, -97.43430234772971232, 1.382123642611622572 ) ) ;
#21426=VECTOR ( 'NONE', #24561, 1000.000000000000000 ) ;
#21429=( NAMED_UNIT ( * ) SI_UNIT ( $, .STERADIAN. ) SOLID_ANGLE_UNIT ( ) );
#21433=ORIENTED_EDGE ( 'NONE', *, *, #16252, .F. ) ;
#21437=CARTESIAN_POINT ( 'NONE',  ( -12.79312068399999980, -101.1716782080000030, -9.159770265490001506 ) ) ;
#21442=CIRCLE ( 'NONE', #9333, 18.64285714289999873 ) ;
#21449=CARTESIAN_POINT ( 'NONE',  ( -22.22671645450000000, -94.70873790529999781, -8.207211804499998209 ) ) ;
#21454=ADVANCED_FACE ( 'NONE', ( #4246 ), #7970, .F. ) ;
#21458=VERTEX_POINT ( 'NONE', #6583 ) ;
#21460=CARTESIAN_POINT ( 'NONE',  ( 0.08412725538310000806, -101.1700440390000040, -15.30178034989999958 ) ) ;
#21462=CARTESIAN_POINT ( 'NONE',  ( 15.50925565250000027, -100.9197086960000007, 1.894555174519999996 ) ) ;
#21466=CARTESIAN_POINT ( 'NONE',  ( 6.252384452659999425, -100.1340845430000002, 15.41982103239999979 ) ) ;
#21467=CARTESIAN_POINT ( 'NONE',  ( 15.58391247289999981, -101.4121386959999995, 3.523358517780000199 ) ) ;
#21470=CARTESIAN_POINT ( 'NONE',  ( 23.00372540730000281, -92.50000000000000000, -20.02694728079999820 ) ) ;
#21471=CARTESIAN_POINT ( 'NONE',  ( 5.046652419183167204, -92.65976904077027143, -30.07958860648908583 ) ) ;
#21473=CARTESIAN_POINT ( 'NONE',  ( 1.955333439440000154, -92.99999932709999939, -29.74887251719999881 ) ) ;
#21483=CARTESIAN_POINT ( 'NONE',  ( -0.8955242351559999925, -101.2530993039999885, -15.16897421750000063 ) ) ;
#21486=CARTESIAN_POINT ( 'NONE',  ( 13.53859855288502878, -92.62938374250892082, 27.33052066698929750 ) ) ;
#21492=CARTESIAN_POINT ( 'NONE',  ( -12.84485488516277840, -101.3051320416489176, -9.329032816835999498 ) ) ;
#21493=DIRECTION ( 'NONE',  ( 0.000000000000000000, 1.000000000000000000, 0.000000000000000000 ) ) ;
#21501=AXIS2_PLACEMENT_3D ( 'NONE', #19458, #8527, #23980 ) ;
#21503=CARTESIAN_POINT ( 'NONE',  ( -0.1868532263790000092, -101.1889999979999999, -16.79896085689999907 ) ) ;
#21505=CARTESIAN_POINT ( 'NONE',  ( -0.6998919996272167099, -101.1416252791453161, -15.52603992147200174 ) ) ;
#21511=DIRECTION ( 'NONE',  ( 0.000000000000000000, 1.000000000000000000, 0.000000000000000000 ) ) ;
#21522=CARTESIAN_POINT ( 'NONE',  ( 21.80109759570151340, -96.92941680763301804, -3.102706385432779879 ) ) ;
#21523=CARTESIAN_POINT ( 'NONE',  ( -12.40996983109999974, -101.1412505549999992, -10.36257240380000155 ) ) ;
#21524=AXIS2_PLACEMENT_3D ( 'NONE', #16783, #16927, #1635 ) ;
#21525=CARTESIAN_POINT ( 'NONE',  ( 19.53781279187136022, -93.86980009075321618, 16.40476867545000417 ) ) ;
#21526=CARTESIAN_POINT ( 'NONE',  ( -7.880236046065482114, -100.4872618029792619, 14.96335263205392963 ) ) ;
#21527=B_SPLINE_CURVE_WITH_KNOTS ( 'NONE', 3,
 ( #12045, #20960, #23001, #11757, #1017, #27521, #25335, #3052, #11905, #874 ),
 .UNSPECIFIED., .F., .F.,
 ( 4, 2, 2, 2, 4 ),
 ( 0.000000000000000000, 0.2500000000000000000, 0.5000000000000000000, 0.7500000000000000000, 1.000000000000000000 ),
 .UNSPECIFIED. ) ;
#21528=VERTEX_POINT ( 'NONE', #15741 ) ;
#21530=DIRECTION ( 'NONE',  ( 0.5193452265677850344, 0.000000000000000000, 0.8545645298286467240 ) ) ;
#21535=CARTESIAN_POINT ( 'NONE',  ( 6.660738224123119444, -101.1451610293114243, 14.97649247838033304 ) ) ;
#21536=CARTESIAN_POINT ( 'NONE',  ( 11.89948051634188531, -101.2404586421460380, -10.39979277174668759 ) ) ;
#21541=CARTESIAN_POINT ( 'NONE',  ( 21.75659477429999811, -111.0000000000000000, -13.30039788230000042 ) ) ;
#21544=CARTESIAN_POINT ( 'NONE',  ( 11.97048044210000128, -101.2358105800000061, -9.395351924210000760 ) ) ;
#21545=EDGE_CURVE ( 'NONE', #4293, #17438, #13053, .T. ) ;
#21547=VERTEX_POINT ( 'NONE', #194 ) ;
#21551=ORIENTED_EDGE ( 'NONE', *, *, #6811, .T. ) ;
#21553=CARTESIAN_POINT ( 'NONE',  ( -18.76759046260000119, -96.83679385039999943, -9.979844675380000751 ) ) ;
#21554=CARTESIAN_POINT ( 'NONE',  ( 13.53079842320000026, -100.4071172650000108, -9.942387125549998927 ) ) ;
#21556=CARTESIAN_POINT ( 'NONE',  ( 23.53303068880000026, -92.50000942380000879, -18.47479182160000022 ) ) ;
#21563=CARTESIAN_POINT ( 'NONE',  ( 0.3059185938709999553, -92.50000000000000000, 14.72672055670000013 ) ) ;
#21564=DIRECTION ( 'NONE',  ( 0.5762746169049438594, 0.000000000000000000, -0.8172561201429208166 ) ) ;
#21568=EDGE_CURVE ( 'NONE', #6448, #23842, #11680, .T. ) ;
#21569=ORIENTED_EDGE ( 'NONE', *, *, #1308, .F. ) ;
#21577=CARTESIAN_POINT ( 'NONE',  ( -12.47452166779999949, -101.1848541600000004, -8.829639320900001920 ) ) ;
#21580=CARTESIAN_POINT ( 'NONE',  ( -7.925865731170000039, -99.78393592979999482, 15.40304860989999902 ) ) ;
#21581=DIRECTION ( 'NONE',  ( 1.000000000000000000, 0.000000000000000000, 0.000000000000000000 ) ) ;
#21583=AXIS2_PLACEMENT_3D ( 'NONE', #2952, #25245, #13562 ) ;
#21586=CARTESIAN_POINT ( 'NONE',  ( 13.55253169098114263, -100.5550990433908538, -10.02507008700657920 ) ) ;
#21589=CARTESIAN_POINT ( 'NONE',  ( 7.132709192110000096, -99.83167692499999646, 15.78738634319999967 ) ) ;
#21590=ORIENTED_EDGE ( 'NONE', *, *, #5663, .F. ) ;
#21593=CARTESIAN_POINT ( 'NONE',  ( -17.65264067069999854, -93.65249602680000862, 18.18801510169999958 ) ) ;
#21594=CARTESIAN_POINT ( 'NONE',  ( -20.62076907760296507, -93.14879094580942365, 16.44113247062627181 ) ) ;
#21597=DIRECTION ( 'NONE',  ( 1.000000000000000000, 0.000000000000000000, 0.000000000000000000 ) ) ;
#21600=CARTESIAN_POINT ( 'NONE',  ( -0.1779554536940000098, -101.6484611540000031, -15.99901033990000165 ) ) ;
#21602=CARTESIAN_POINT ( 'NONE',  ( 15.33316675979999921, -101.1045726949999874, 2.495933759240000160 ) ) ;
#21606=EDGE_CURVE ( 'NONE', #1588, #7139, #25214, .T. ) ;
#21607=CARTESIAN_POINT ( 'NONE',  ( 6.895355905279999753, -99.94751438429999268, 15.70952527899999929 ) ) ;
#21608=CARTESIAN_POINT ( 'NONE',  ( 15.13453645979999962, -101.1292389600000092, 3.376594308710000103 ) ) ;
#21615=ADVANCED_FACE ( 'NONE', ( #13564 ), #26694, .T. ) ;
#21618=CARTESIAN_POINT ( 'NONE',  ( 4.474575075100000632, -92.65715406910000240, -27.57907939949999943 ) ) ;
#21620=CARTESIAN_POINT ( 'NONE',  ( -6.592280350930000310, -101.1848541609999899, 13.78765661559999955 ) ) ;
#21621=VERTEX_POINT ( 'NONE', #20421 ) ;
#21624=CARTESIAN_POINT ( 'NONE',  ( -12.54500315030344382, -101.0147714269334074, -10.70743288971485363 ) ) ;
#21629=CARTESIAN_POINT ( 'NONE',  ( 4.794255386040000566, -107.5000000000000000, 8.775825618900000791 ) ) ;
#21631=CARTESIAN_POINT ( 'NONE',  ( 16.19501884596224883, -94.70448199252453492, 17.23845109483602656 ) ) ;
#21638=ORIENTED_EDGE ( 'NONE', *, *, #18095, .T. ) ;
#21642=ADVANCED_FACE ( 'NONE', ( #16042 ), #2362, .F. ) ;
#21643=EDGE_CURVE ( 'NONE', #15494, #21689, #5212, .T. ) ;
#21646=CARTESIAN_POINT ( 'NONE',  ( -29.08067107640000160, -92.50732182800000203, 4.792447498680000528 ) ) ;
#21650=CARTESIAN_POINT ( 'NONE',  ( 15.66940200309999831, -100.9678331089999972, 4.038298765579999561 ) ) ;
#21654=EDGE_LOOP ( 'NONE', ( #20492, #26568, #3903, #18510 ) ) ;
#21659=CARTESIAN_POINT ( 'NONE',  ( -14.86016661329999877, -101.1848541609999899, 3.566077570999999669 ) ) ;
#21664=CARTESIAN_POINT ( 'NONE',  ( -12.50546161790000177, -100.7430069139999915, -10.75263243640000077 ) ) ;
#21665=CARTESIAN_POINT ( 'NONE',  ( -7.571352933129060325, -101.1248211533539205, 14.55532840934864147 ) ) ;
#21667=CARTESIAN_POINT ( 'NONE',  ( -1.007768741648868760, -101.5703832412493739, -16.02700633418644216 ) ) ;
#21672=CARTESIAN_POINT ( 'NONE',  ( 6.669130659221032431, -101.2111896145234340, 14.91624109844728707 ) ) ;
#21678=CARTESIAN_POINT ( 'NONE',  ( -20.42407875355905134, -94.65351867482938530, 12.05937522786372185 ) ) ;
#21680=CARTESIAN_POINT ( 'NONE',  ( 28.56790285990000200, -92.99999932720000118, 8.526057022789998996 ) ) ;
#21681=CARTESIAN_POINT ( 'NONE',  ( 3.166345171159999694, -101.1889999979999999, -25.30265318609999881 ) ) ;
#21684=CARTESIAN_POINT ( 'NONE',  ( -5.025833696325614497, -96.36359510987577437, -21.36185927323176159 ) ) ;
#21689=VERTEX_POINT ( 'NONE', #18828 ) ;
#21690=CARTESIAN_POINT ( 'NONE',  ( -22.22671705529999997, -94.70873613630000420, -8.207212726500001665 ) ) ;
#21691=CARTESIAN_POINT ( 'NONE',  ( 12.38290840660000036, -101.0875971110000080, -9.170880648609999852 ) ) ;
#21693=CARTESIAN_POINT ( 'NONE',  ( 23.79916314309999947, -94.54647010780000471, -7.453462340879999815 ) ) ;
#21695=CARTESIAN_POINT ( 'NONE',  ( 29.97548914054884506, -92.50000000000001421, 5.633735048817801072 ) ) ;
#21699=CARTESIAN_POINT ( 'NONE',  ( -18.80176912509999809, -93.00000000000000000, 23.77750384849999676 ) ) ;
#21702=CARTESIAN_POINT ( 'NONE',  ( 0.05579740145615928043, -92.84927079008861028, -30.49995016637035761 ) ) ;
#21709=DIRECTION ( 'NONE',  ( 1.000000000000000000, 0.000000000000000000, 0.000000000000000000 ) ) ;
#21715=CARTESIAN_POINT ( 'NONE',  ( -12.96301527429999823, -100.9938510739999913, -8.551186485709999729 ) ) ;
#21717=CARTESIAN_POINT ( 'NONE',  ( -8.209463909749999289, -99.53431386179998697, 15.35748980570000022 ) ) ;
#21718=EDGE_LOOP ( 'NONE', ( #25490, #20530, #9786, #11743 ) ) ;
#21719=CARTESIAN_POINT ( 'NONE',  ( -2.903042209430000131, -94.98812656900000206, 23.52859605189999925 ) ) ;
#21723=VERTEX_POINT ( 'NONE', #10043 ) ;
#21724=CARTESIAN_POINT ( 'NONE',  ( 13.00837423133404158, -101.2637735886917625, -9.819042233897015137 ) ) ;
#21727=CARTESIAN_POINT ( 'NONE',  ( -15.62855498089999884, -101.6223710729999965, 3.522773483530000416 ) ) ;
#21738=CARTESIAN_POINT ( 'NONE',  ( 26.73328265790000202, -93.00000450890000536, -12.41349335419999989 ) ) ;
#21739=CARTESIAN_POINT ( 'NONE',  ( 15.14237901210000103, -101.1411470200000053, 2.745305927470000018 ) ) ;
#21744=CARTESIAN_POINT ( 'NONE',  ( 6.612443239639999248, -100.9678331089999972, 14.76866989470000213 ) ) ;
#21745=CARTESIAN_POINT ( 'NONE',  ( 14.89070032189999893, -101.0875971110000080, 3.963397078339999879 ) ) ;
#21748=CARTESIAN_POINT ( 'NONE',  ( 5.025650632445116450, -92.66455718074428205, -30.08309967992143896 ) ) ;
#21750=VERTEX_POINT ( 'NONE', #5416 ) ;
#21751=CARTESIAN_POINT ( 'NONE',  ( 1.798767253769999908, -92.50732182800000203, -29.41797783070000349 ) ) ;
#21754=CARTESIAN_POINT ( 'NONE',  ( -1.108943289259999965, -101.2141467319999890, -15.20603369630000046 ) ) ;
#21758=CARTESIAN_POINT ( 'NONE',  ( -12.59800300965208208, -100.8945630382227989, -10.79107909087879769 ) ) ;
#21760=CARTESIAN_POINT ( 'NONE',  ( 23.56050310359999855, -94.79581646409999962, -2.314011072670000058 ) ) ;
#21762=CARTESIAN_POINT ( 'NONE',  ( -1.325730538359999988, -100.9728541479999961, -15.54355591019999849 ) ) ;
#21766=CARTESIAN_POINT ( 'NONE',  ( 12.82422237299999956, -94.98812477769999418, -19.93894812050000098 ) ) ;
#21770=CARTESIAN_POINT ( 'NONE',  ( 15.04861839279999991, -100.9137139110000021, 4.234011249179999936 ) ) ;
#21772=B_SPLINE_CURVE_WITH_KNOTS ( 'NONE', 5,
 ( #28148, #19261, #21727, #1777, #10620, #19536, #26391, #26255, #6278, #12960, #1507, #6420 ),
 .UNSPECIFIED., .F., .F.,
 ( 6, 3, 3, 6 ),
 ( 0.000000000000000000, 0.2661689441622204222, 0.5687008854760363663, 1.000000000000000000 ),
 .UNSPECIFIED. ) ;
#21773=CARTESIAN_POINT ( 'NONE',  ( -12.78693177215897236, -101.2404586421391173, -9.286964095330146662 ) ) ;
#21774=CARTESIAN_POINT ( 'NONE',  ( 13.76083776420598248, -100.1240332945478144, -10.32414654847229762 ) ) ;
#21783=CARTESIAN_POINT ( 'NONE',  ( -26.99515064810000098, -93.07154530319999708, -0.5147607136670000472 ) ) ;
#21785=CYLINDRICAL_SURFACE ( 'NONE', #23413, 16.00000000000000000 ) ;
#21787=CARTESIAN_POINT ( 'NONE',  ( -17.89732362545216660, -97.43022994619724386, -10.14686946726538608 ) ) ;
#21788=CARTESIAN_POINT ( 'NONE',  ( -13.14571738459999928, -100.8733984769999950, -8.628956128260000469 ) ) ;
#21802=CARTESIAN_POINT ( 'NONE',  ( -11.89545460579999947, -101.2530993010000060, -9.453770335970000716 ) ) ;
#21805=CARTESIAN_POINT ( 'NONE',  ( -7.068540044037536774, -101.5740747342563850, 14.41783971523548047 ) ) ;
#21809=FACE_OUTER_BOUND ( 'NONE', #9443, .T. ) ;
#21813=AXIS2_PLACEMENT_3D ( 'NONE', #21085, #21493, #3578 ) ;
#21815=CIRCLE ( 'NONE', #457, 21.14285714289999873 ) ;
#21817=CARTESIAN_POINT ( 'NONE',  ( -5.487412872479999315, -100.8733984769999950, 14.73625018059999903 ) ) ;
#21820=CARTESIAN_POINT ( 'NONE',  ( -15.59829199139345413, -93.74885976911515684, -21.59132595434880031 ) ) ;
#21828=CARTESIAN_POINT ( 'NONE',  ( -20.51427898140000394, -93.04780269089999933, -20.71378216980000175 ) ) ;
#21830=EDGE_LOOP ( 'NONE', ( #13414, #5095, #23063, #25322, #5276, #5139 ) ) ;
#21835=CARTESIAN_POINT ( 'NONE',  ( 12.43657857140000011, -101.0151300849999814, -9.480717691399998870 ) ) ;
#21839=CARTESIAN_POINT ( 'NONE',  ( 29.92224321301734946, -92.52048598158077652, 5.908436733558301235 ) ) ;
#21841=ORIENTED_EDGE ( 'NONE', *, *, #11193, .T. ) ;
#21848=SHAPE_DEFINITION_REPRESENTATION ( #5706, #10908 ) ;
#21849=CARTESIAN_POINT ( 'NONE',  ( -11.60601438770000016, -94.60987696080000831, -20.74983651260000173 ) ) ;
#21852=ORIENTED_EDGE ( 'NONE', *, *, #1888, .T. ) ;
#21857=DIRECTION ( 'NONE',  ( 0.000000000000000000, -1.000000000000000000, 0.000000000000000000 ) ) ;
#21859=CARTESIAN_POINT ( 'NONE',  ( -12.94585355969999974, -101.5369810359999860, -9.402386697489999889 ) ) ;
#21861=DIRECTION ( 'NONE',  ( 0.000000000000000000, 1.000000000000000000, 0.000000000000000000 ) ) ;
#21862=VERTEX_POINT ( 'NONE', #9914 ) ;
#21863=CARTESIAN_POINT ( 'NONE',  ( -1.640146184310000033, -93.85307999910000376, 24.85263355689999898 ) ) ;
#21865=CARTESIAN_POINT ( 'NONE',  ( -30.40361236680223200, -92.82334897394798645, 2.422884163522351919 ) ) ;
#21871=CARTESIAN_POINT ( 'NONE',  ( 13.63023407945182619, -100.4166221066929836, -10.10576425320335048 ) ) ;
#21875=ORIENTED_EDGE ( 'NONE', *, *, #22419, .T. ) ;
#21878=CARTESIAN_POINT ( 'NONE',  ( -17.23516852259999865, -93.34894302420001111, 19.23197678129999844 ) ) ;
#21879=CARTESIAN_POINT ( 'NONE',  ( -20.53595003809872566, -92.95311892457516478, 17.44055191160039797 ) ) ;
#21882=EDGE_CURVE ( 'NONE', #19526, #3430, #14975, .T. ) ;
#21884=CARTESIAN_POINT ( 'NONE',  ( 0.6097187718590001415, -100.7430069139999915, -16.48132026290000240 ) ) ;
#21886=CARTESIAN_POINT ( 'NONE',  ( 15.25760145080000107, -101.1292389600000092, 2.766195699469999436 ) ) ;
#21891=CARTESIAN_POINT ( 'NONE',  ( 6.435168149109999902, -100.5717442099999914, 15.00978900200000155 ) ) ;
#21892=CARTESIAN_POINT ( 'NONE',  ( -15.60056067142878788, -92.58043237596167785, -24.03344884106981993 ) ) ;
#21893=CARTESIAN_POINT ( 'NONE',  ( -17.19936155160000268, -93.49273751280000511, 18.87523342240000090 ) ) ;
#21894=CARTESIAN_POINT ( 'NONE',  ( 5.095278765311285873, -92.64884742706659893, -30.07140691049922410 ) ) ;
#21897=CARTESIAN_POINT ( 'NONE',  ( 6.262252868900000102, -92.98481302140000082, -25.92940123820000053 ) ) ;
#21899=CIRCLE ( 'NONE', #3743, 0.4999999999999990563 ) ;
#21902=CARTESIAN_POINT ( 'NONE',  ( -6.929612297000000254, -101.5216621940000152, 14.43317662559999981 ) ) ;
#21905=B_SPLINE_CURVE_WITH_KNOTS ( 'NONE', 3,
 ( #7925, #1113, #27319, #20909, #9813, #10081, #12136, #21054, #20768, #5594, #16526, #14475, #5455, #9951, #7359, #18865, #23372, #19000 ),
 .UNSPECIFIED., .F., .F.,
 ( 4, 2, 2, 2, 1, 1, 1, 1, 2, 2, 4 ),
 ( 0.000000000000000000, 0.2500000000000449085, 0.3750000000000673905, 0.4375000000000786038, 0.4687500000000842104, 0.4843750000000877631, 0.4921875000000898170, 0.4960937500000907607, 0.4980468750000903166, 0.5000000000000898170, 1.000000000000000000 ),
 .UNSPECIFIED. ) ;
#21910=EDGE_CURVE ( 'NONE', #22153, #7941, #23813, .T. ) ;
#21911=CARTESIAN_POINT ( 'NONE',  ( -1.247133441849999969, -101.2306315440000049, -16.16540283980000225 ) ) ;
#21917=CARTESIAN_POINT ( 'NONE',  ( -15.42268928690000074, -101.6484615499999933, 4.259183627459999677 ) ) ;
#21918=CARTESIAN_POINT ( 'NONE',  ( -6.569756907160000381, -101.2530993010000060, 13.70087252790000143 ) ) ;
#21921=DIRECTION ( 'NONE',  ( 0.000000000000000000, -1.000000000000000000, 0.000000000000000000 ) ) ;
#21923=CARTESIAN_POINT ( 'NONE',  ( 24.29194483483871636, -94.04667188331129069, -9.262494893684873887 ) ) ;
#21926=ORIENTED_EDGE ( 'NONE', *, *, #20609, .F. ) ;
#21931=VERTEX_POINT ( 'NONE', #25802 ) ;
#21934=CARTESIAN_POINT ( 'NONE',  ( -26.75452624049999883, -92.97898997910000674, -0.3867577180200000297 ) ) ;
#21942=AXIS2_PLACEMENT_3D ( 'NONE', #22470, #2514, #16184 ) ;
#21944=B_SPLINE_CURVE_WITH_KNOTS ( 'NONE', 5,
 ( #6018, #28042, #3568, #12426, #21339, #10240, #19155, #15172, #23949 ),
 .UNSPECIFIED., .F., .F.,
 ( 6, 3, 6 ),
 ( 0.000000000000000000, 0.5000000000000000000, 1.000000000000000000 ),
 .UNSPECIFIED. ) ;
#21949=DIRECTION ( 'NONE',  ( 1.000000000000000000, 0.000000000000000000, 0.000000000000000000 ) ) ;
#21952=CARTESIAN_POINT ( 'NONE',  ( -17.54428855099999751, -94.59276292389999696, 16.07755916609999858 ) ) ;
#21953=B_SPLINE_SURFACE_WITH_KNOTS ( 'NONE', 5, 5, ( 
 ( #4335, #22116, #10993, #2301, #4477, #4034, #21817, #1867, #19906 ),
 ( #17743, #19625, #11149, #27662, #7258, #866, #7403, #22699, #9276 ),
 ( #9856, #11449, #4776, #576, #2741, #9572, #13948, #14243, #22848 ),
 ( #3178, #12035, #2891, #9708, #16124, #23131, #16421, #2601, #1011 ),
 ( #18766, #27216, #24739, #16268, #14096, #18175, #13653, #25181, #11751 ),
 ( #22560, #27513, #25024, #11598, #5056, #20954, #18621, #20357, #20506 ) ),
 .UNSPECIFIED., .F., .F., .F.,
 ( 6, 6 ),
 ( 6, 3, 6 ),
 ( 10.27983904170000073, 28.98451592950000233 ),
 ( 0.000000000000000000, 0.2500000000000000000, 0.5000000000000000000 ),
 .UNSPECIFIED. ) ;
#21956=CARTESIAN_POINT ( 'NONE',  ( -11.96873758509999952, -101.1030539030000028, -9.749858522220000268 ) ) ;
#21967=CARTESIAN_POINT ( 'NONE',  ( -14.77445022520000073, -101.2530993010000060, 3.545507728379999612 ) ) ;
#21968=CARTESIAN_POINT ( 'NONE',  ( -19.26870743061221347, -97.04550385075440033, 7.366219023504180008 ) ) ;
#21970=CARTESIAN_POINT ( 'NONE',  ( 23.84088130539999995, -93.01125933519999478, 11.79630522170000084 ) ) ;
#21973=VERTEX_POINT ( 'NONE', #24318 ) ;
#21976=AXIS2_PLACEMENT_3D ( 'NONE', #26383, #6411, #12429 ) ;
#21981=CARTESIAN_POINT ( 'NONE',  ( -13.46646228700000059, -101.3150700380000018, -9.098096927170001180 ) ) ;
#21984=CARTESIAN_POINT ( 'NONE',  ( 12.86597616020000068, -100.8023006570000035, -9.130347141119999677 ) ) ;
#21985=CARTESIAN_POINT ( 'NONE',  ( -18.26810397560000254, -94.98812477769999418, 16.32728546869999775 ) ) ;
#21987=CARTESIAN_POINT ( 'NONE',  ( 26.66586753799999698, -92.50000000000000000, 13.56661073689999952 ) ) ;
#21993=CARTESIAN_POINT ( 'NONE',  ( -23.89417554923151243, -92.74292563043789528, -18.95570639509220712 ) ) ;
#21995=CARTESIAN_POINT ( 'NONE',  ( 0.09048303299432611246, -92.89593097428102908, -30.49986667271737062 ) ) ;
#22005=CARTESIAN_POINT ( 'NONE',  ( 19.73038513050000020, -98.60488090890000024, -0.3427724926369999925 ) ) ;
#22007=CARTESIAN_POINT ( 'NONE',  ( -18.13877362739999910, -92.50000000000000000, -23.79298866759999598 ) ) ;
#22009=ADVANCED_FACE ( 'NONE', ( #11622 ), #10292, .F. ) ;
#22014=CARTESIAN_POINT ( 'NONE',  ( -14.10686381969999914, -92.91112761319999436, -23.69005823610000050 ) ) ;
#22015=CARTESIAN_POINT ( 'NONE',  ( -11.16205616639999931, -94.83055275160000974, -21.09956017769999903 ) ) ;
#22017=CARTESIAN_POINT ( 'NONE',  ( 1.312652382290000030, -94.71481430560001513, 24.32357623499999733 ) ) ;
#22018=CARTESIAN_POINT ( 'NONE',  ( -20.20035178370000040, -94.89195255890000169, 12.35537463580000050 ) ) ;
#22019=CARTESIAN_POINT ( 'NONE',  ( -29.68006920950033134, -92.66191076879675848, 7.024780034912508242 ) ) ;
#22020=CARTESIAN_POINT ( 'NONE',  ( 11.88502995134358819, -99.07183862004048081, -15.04908790469807300 ) ) ;
#22027=AXIS2_PLACEMENT_3D ( 'NONE', #3535, #25407, #5436 ) ;
#22029=CARTESIAN_POINT ( 'NONE',  ( -15.01536691379999944, -92.56128749459999483, 24.94218803040000054 ) ) ;
#22030=CARTESIAN_POINT ( 'NONE',  ( -20.53865360145708863, -92.95759695848158799, 17.41522175122109317 ) ) ;
#22032=CARTESIAN_POINT ( 'NONE',  ( 8.831064126840001194, -94.59276292389999696, -22.09756266850000017 ) ) ;
#22034=CARTESIAN_POINT ( 'NONE',  ( 0.6195791821380000064, -100.2522625769999962, -17.00587765690000097 ) ) ;
#22039=EDGE_LOOP ( 'NONE', ( #3877, #27356, #18090, #17158 ) ) ;
#22042=AXIS2_PLACEMENT_3D ( 'NONE', #21629, #23669, #10518 ) ;
#22045=CARTESIAN_POINT ( 'NONE',  ( 28.01404095332314625, -92.56492639277975343, 12.06120875835872042 ) ) ;
#22046=CARTESIAN_POINT ( 'NONE',  ( 15.55009014945955315, -101.2404586421511965, 2.819223758050509954 ) ) ;
#22050=CARTESIAN_POINT ( 'NONE',  ( 8.472249407519999664, -94.22763312370000222, -22.74885336210000020 ) ) ;
#22051=EDGE_CURVE ( 'NONE', #26855, #22409, #7514, .T. ) ;
#22052=CARTESIAN_POINT ( 'NONE',  ( -0.8955242351559999925, -101.2530993039999885, -15.16897421750000063 ) ) ;
#22053=DIRECTION ( 'NONE',  ( 0.000000000000000000, -1.000000000000000000, 0.000000000000000000 ) ) ;
#22054=ORIENTED_EDGE ( 'NONE', *, *, #22754, .F. ) ;
#22059=CARTESIAN_POINT ( 'NONE',  ( 26.58751350659999702, -92.65509162889999573, -7.785010380240000138 ) ) ;
#22060=CARTESIAN_POINT ( 'NONE',  ( -1.108943289259999965, -101.2141467319999890, -15.20603369630000046 ) ) ;
#22061=CIRCLE ( 'NONE', #9947, 18.64285714289999873 ) ;
#22064=AXIS2_PLACEMENT_3D ( 'NONE', #25867, #23816, #14771 ) ;
#22067=CARTESIAN_POINT ( 'NONE',  ( -7.476488366829999954, -100.9137139110000021, 13.72916197330000010 ) ) ;
#22073=CARTESIAN_POINT ( 'NONE',  ( 24.76402736475559152, -93.25521310992057522, -13.40803308253799919 ) ) ;
#22074=CARTESIAN_POINT ( 'NONE',  ( 20.81361611080448881, -94.60934249687453246, 13.89502885642193064 ) ) ;
#22086=EDGE_CURVE ( 'NONE', #11556, #7139, #17908, .T. ) ;
#22087=CARTESIAN_POINT ( 'NONE',  ( 16.16228525779999714, -100.3517545579999961, 4.402890113689999829 ) ) ;
#22088=VERTEX_POINT ( 'NONE', #14677 ) ;
#22099=CARTESIAN_POINT ( 'NONE',  ( -16.40265326879195129, -98.81923691017613010, 8.200441858953826824 ) ) ;
#22101=VERTEX_POINT ( 'NONE', #15084 ) ;
#22103=CARTESIAN_POINT ( 'NONE',  ( -15.38068916850000001, -101.6095197629999944, 4.516181925269999731 ) ) ;
#22105=CARTESIAN_POINT ( 'NONE',  ( -12.50278151429999873, -101.3256027139999986, -9.834025437379999346 ) ) ;
#22108=VERTEX_POINT ( 'NONE', #1859 ) ;
#22114=B_SPLINE_CURVE_WITH_KNOTS ( 'NONE', 3,
 ( #23852, #10988, #26332, #15221, #1717, #12756, #1863, #21667, #19471, #19620, #4176, #10702 ),
 .UNSPECIFIED., .F., .F.,
 ( 4, 2, 2, 2, 2, 4 ),
 ( 0.000000000000000000, 0.2500000000000487943, 0.3750000000000819900, 0.4375000000000869860, 0.5000000000000920375, 1.000000000000000000 ),
 .UNSPECIFIED. ) ;
#22116=CARTESIAN_POINT ( 'NONE',  ( -5.890278778139999893, -101.2306310700000012, 15.10563525420000097 ) ) ;
#22121=ORIENTED_EDGE ( 'NONE', *, *, #20134, .T. ) ;
#22122=CARTESIAN_POINT ( 'NONE',  ( 23.93718440349999810, -92.97899053829999616, 11.95681231160000024 ) ) ;
#22123=CARTESIAN_POINT ( 'NONE',  ( -14.94261203119999948, -100.8733967390000004, 4.897670397449999768 ) ) ;
#22127=ORIENTED_EDGE ( 'NONE', *, *, #16821, .F. ) ;
#22129=CARTESIAN_POINT ( 'NONE',  ( -21.81061053790000059, -92.49999926799999628, -19.59831469680000282 ) ) ;
#22133=CARTESIAN_POINT ( 'NONE',  ( 12.68316649459999823, -100.8772072149999985, -9.423397405859999409 ) ) ;
#22136=DIRECTION ( 'NONE',  ( 0.000000000000000000, 1.000000000000000000, 0.000000000000000000 ) ) ;
#22140=DIRECTION ( 'NONE',  ( 0.9999792992113792911, 0.000000000000000000, 0.006434372441722326086 ) ) ;
#22141=ORIENTED_EDGE ( 'NONE', *, *, #8750, .T. ) ;
#22144=CARTESIAN_POINT ( 'NONE',  ( -24.15301378228902252, -92.58608763742770975, -18.62476874987404329 ) ) ;
#22145=FACE_OUTER_BOUND ( 'NONE', #12625, .T. ) ;
#22152=CARTESIAN_POINT ( 'NONE',  ( 20.62756379660000050, -97.01506440939999720, -2.488770823180000313 ) ) ;
#22153=VERTEX_POINT ( 'NONE', #3610 ) ;
#22154=DIRECTION ( 'NONE',  ( 0.000000000000000000, 1.000000000000000000, 0.000000000000000000 ) ) ;
#22157=CARTESIAN_POINT ( 'NONE',  ( 15.91666809940000071, -101.0685849509999912, 2.371725914449999806 ) ) ;
#22161=FACE_OUTER_BOUND ( 'NONE', #15506, .T. ) ;
#22162=CARTESIAN_POINT ( 'NONE',  ( -29.69325694440044572, -92.68577957612751561, 6.968726778918060027 ) ) ;
#22165=CARTESIAN_POINT ( 'NONE',  ( 11.32290720589999822, -93.36531860510000058, -23.59732887200000206 ) ) ;
#22168=ADVANCED_FACE ( 'NONE', ( #10553 ), #19468, .F. ) ;
#22169=CARTESIAN_POINT ( 'NONE',  ( -13.26851675973651545, -92.83160374581382257, 27.46263779841126507 ) ) ;
#22172=CARTESIAN_POINT ( 'NONE',  ( -16.67583898440000212, -92.84059452359998943, 21.54669423090000180 ) ) ;
#22173=CARTESIAN_POINT ( 'NONE',  ( -6.569460039029999976, -101.6484611540000031, 14.03895276709999962 ) ) ;
#22175=EDGE_CURVE ( 'NONE', #6793, #19902, #22457, .T. ) ;
#22177=CARTESIAN_POINT ( 'NONE',  ( 0.9829826817099999170, -100.1512121650000040, -16.61044266980000117 ) ) ;
#22179=CARTESIAN_POINT ( 'NONE',  ( 15.80445266879999799, -101.5026188610000020, 2.634903237490000105 ) ) ;
#22180=EDGE_CURVE ( 'NONE', #11057, #11437, #9221, .T. ) ;
#22184=ORIENTED_EDGE ( 'NONE', *, *, #27969, .F. ) ;
#22187=CARTESIAN_POINT ( 'NONE',  ( -2.986711995579999890, -94.79581469870001342, 23.48470869699999852 ) ) ;
#22189=CARTESIAN_POINT ( 'NONE',  ( 20.48885040240000066, -93.05538536990000864, 16.53376986659999659 ) ) ;
#22191=CARTESIAN_POINT ( 'NONE',  ( -7.155293904009999650, -101.2927714249999980, 14.37234474879999979 ) ) ;
#22194=CARTESIAN_POINT ( 'NONE',  ( -12.91282149864488460, -100.3796496173521007, -11.05327605674254166 ) ) ;
#22197=CARTESIAN_POINT ( 'NONE',  ( 26.20717514349999888, -93.01085527740001169, -7.939310658160000145 ) ) ;
#22198=CARTESIAN_POINT ( 'NONE',  ( 9.119802927630001221, -98.28914429610000525, 16.69368728350000097 ) ) ;
#22200=CARTESIAN_POINT ( 'NONE',  ( -25.37284092810000047, -93.00000000000000000, 2.543411731580000001 ) ) ;
#22201=CARTESIAN_POINT ( 'NONE',  ( -20.33391829737038492, -92.64884742716812127, -22.73286488652288639 ) ) ;
#22203=CARTESIAN_POINT ( 'NONE',  ( 11.34527656030000031, -101.0555477039999914, -10.55639998680000069 ) ) ;
#22205=CARTESIAN_POINT ( 'NONE',  ( 16.32839208820038834, -94.64093351176255453, 17.22545126736804022 ) ) ;
#22207=AXIS2_PLACEMENT_3D ( 'NONE', #7786, #21052, #14047 ) ;
#22208=DIRECTION ( 'NONE',  ( 1.000000000000000000, 0.000000000000000000, 0.000000000000000000 ) ) ;
#22210=CARTESIAN_POINT ( 'NONE',  ( -30.34790777679999962, -111.0000000000000000, 3.042119914239999723 ) ) ;
#22211=CARTESIAN_POINT ( 'NONE',  ( 27.44308006103930708, -93.08694455168847526, 9.636015041101046563 ) ) ;
#22215=CARTESIAN_POINT ( 'NONE',  ( 7.799868133589999530, -101.0912156119999992, 13.74000810979999798 ) ) ;
#22216=AXIS2_PLACEMENT_3D ( 'NONE', #7127, #20228, #17904 ) ;
#22220=CARTESIAN_POINT ( 'NONE',  ( -24.70281971250000197, -94.64125147560000073, -3.583037810470000029 ) ) ;
#22228=VERTEX_POINT ( 'NONE', #25843 ) ;
#22233=CARTESIAN_POINT ( 'NONE',  ( 24.85760066650000155, -93.16461275549998788, -13.76036209870000171 ) ) ;
#22234=EDGE_CURVE ( 'NONE', #2616, #2738, #6118, .T. ) ;
#22237=CARTESIAN_POINT ( 'NONE',  ( 19.57843399940000140, -94.59276292389999696, 13.52682119470000011 ) ) ;
#22238=CARTESIAN_POINT ( 'NONE',  ( 14.11489916659999899, -97.73638926259998527, -14.10864689489999968 ) ) ;
#22241=CARTESIAN_POINT ( 'NONE',  ( 7.678730999230412912, -101.6404041080485001, 14.04396369532980771 ) ) ;
#22244=EDGE_LOOP ( 'NONE', ( #12638, #20311, #14653, #11245 ) ) ;
#22246=CARTESIAN_POINT ( 'NONE',  ( 26.65335633700317430, -92.66455718076046821, -14.82729397443163499 ) ) ;
#22247=VECTOR ( 'NONE', #18206, 1000.000000000000114 ) ;
#22249=ORIENTED_EDGE ( 'NONE', *, *, #4942, .T. ) ;
#22251=DIRECTION ( 'NONE',  ( 0.000000000000000000, 1.000000000000000000, 0.000000000000000000 ) ) ;
#22253=CARTESIAN_POINT ( 'NONE',  ( 11.95338359237086223, -101.3051320416555825, -10.44690246017028912 ) ) ;
#22257=EDGE_LOOP ( 'NONE', ( #3935, #6544, #21590, #2440 ) ) ;
#22259=CARTESIAN_POINT ( 'NONE',  ( 21.31694387499999976, -94.06807427549999545, 13.63926651669999934 ) ) ;
#22266=CARTESIAN_POINT ( 'NONE',  ( -14.06008659669999972, -93.67384740789999853, -21.43629181160000385 ) ) ;
#22268=VERTEX_POINT ( 'NONE', #715 ) ;
#22269=CARTESIAN_POINT ( 'NONE',  ( -1.283023294879999998, -101.3150694429999987, -16.20107482390000087 ) ) ;
#22274=CARTESIAN_POINT ( 'NONE',  ( -5.658845926663969017, -98.25430909850952332, -19.43178140796045028 ) ) ;
#22275=CARTESIAN_POINT ( 'NONE',  ( -13.83118819819999956, -111.0000000000000000, 21.42307711379999802 ) ) ;
#22279=CIRCLE ( 'NONE', #13905, 20.64285714289999873 ) ;
#22281=CIRCLE ( 'NONE', #25561, 0.5000000000000001110 ) ;
#22285=CARTESIAN_POINT ( 'NONE',  ( -4.794255386040000566, -108.5000000000000000, -8.775825618900000791 ) ) ;
#22290=ADVANCED_FACE ( 'NONE', ( #11891 ), #5484, .T. ) ;
#22292=CARTESIAN_POINT ( 'NONE',  ( 17.89054857160000367, -99.82967635330000178, 1.194493289920000034 ) ) ;
#22294=EDGE_LOOP ( 'NONE', ( #1220, #6096, #1513, #14696 ) ) ;
#22297=ORIENTED_EDGE ( 'NONE', *, *, #21568, .F. ) ;
#22298=CARTESIAN_POINT ( 'NONE',  ( 14.96040621690000094, -95.42941506580001487, 17.19850698980000203 ) ) ;
#22299=AXIS2_PLACEMENT_3D ( 'NONE', #21090, #13168, #1690 ) ;
#22303=CARTESIAN_POINT ( 'NONE',  ( 8.514116711873594312, -94.35876167791963098, -23.96130013197857878 ) ) ;
#22304=CARTESIAN_POINT ( 'NONE',  ( -23.50862727400000196, -94.59276292389999696, -3.692480628369999796 ) ) ;
#22305=CARTESIAN_POINT ( 'NONE',  ( 29.70835240799999966, -91.50000000000000000, 6.903897247299999762 ) ) ;
#22308=ORIENTED_EDGE ( 'NONE', *, *, #23375, .F. ) ;
#22319=CARTESIAN_POINT ( 'NONE',  ( 0.7684516987970000379, -100.0496341300000154, -16.89528639299999924 ) ) ;
#22324=VECTOR ( 'NONE', #24758, 1000.000000000000000 ) ;
#22326=CARTESIAN_POINT ( 'NONE',  ( -18.99756495820000168, -93.00000000000000000, -23.62136188200000220 ) ) ;
#22327=B_SPLINE_CURVE_WITH_KNOTS ( 'NONE', 5,
 ( #20032, #16092, #11719, #20635, #24410, #97 ),
 .UNSPECIFIED., .F., .F.,
 ( 6, 6 ),
 ( 0.000000000000000000, 1.000000000000000000 ),
 .UNSPECIFIED. ) ;
#22331=CARTESIAN_POINT ( 'NONE',  ( 28.49579638229387513, -92.86276748840948869, 10.87457464806996299 ) ) ;
#22335=CARTESIAN_POINT ( 'NONE',  ( 23.69288052678082934, -92.66191076872320309, -19.20680752137960567 ) ) ;
#22336=CARTESIAN_POINT ( 'NONE',  ( 24.54087331869999744, -92.99999854809999533, 14.48417091049999961 ) ) ;
#22338=CARTESIAN_POINT ( 'NONE',  ( -7.429654490199999017, -101.3090757639999993, 14.46660187589999857 ) ) ;
#22339=ORIENTED_EDGE ( 'NONE', *, *, #14258, .F. ) ;
#22341=CARTESIAN_POINT ( 'NONE',  ( -12.45048480342227037, -101.4304678898350005, -10.31532340321227359 ) ) ;
#22350=CARTESIAN_POINT ( 'NONE',  ( -21.30003612899999865, -91.50000000000000000, -21.83021898440000186 ) ) ;
#22351=CARTESIAN_POINT ( 'NONE',  ( -5.605778865269999578, -95.75647260680000272, -21.78235593370000345 ) ) ;
#22352=CARTESIAN_POINT ( 'NONE',  ( -20.85062936798085786, -92.82334897400905049, -22.25985776189306620 ) ) ;
#22353=CARTESIAN_POINT ( 'NONE',  ( 11.23915397940000105, -100.8869817940000075, -10.91500585829999892 ) ) ;
#22355=CARTESIAN_POINT ( 'NONE',  ( -15.46577867176106302, -100.1470170704337050, -8.781364183522299527 ) ) ;
#22364=CARTESIAN_POINT ( 'NONE',  ( 7.995260568349999986, -101.2398794199999941, 13.96161139179999999 ) ) ;
#22368=CARTESIAN_POINT ( 'NONE',  ( 21.24078103779999793, -96.65227117190001138, 0.9777240160550001447 ) ) ;
#22369=DIRECTION ( 'NONE',  ( 0.04503285875970659130, 0.000000000000000000, 0.9989855062171465461 ) ) ;
#22371=CARTESIAN_POINT ( 'NONE',  ( -25.24361395089999860, -94.34469964519999508, -3.017224276749999934 ) ) ;
#22373=DIRECTION ( 'NONE',  ( 0.000000000000000000, 1.000000000000000000, 0.000000000000000000 ) ) ;
#22377=DIRECTION ( 'NONE',  ( 0.000000000000000000, -1.000000000000000000, 0.000000000000000000 ) ) ;
#22381=CARTESIAN_POINT ( 'NONE',  ( 8.363467862889008231, -92.62800705134604584, 29.33100262325347884 ) ) ;
#22386=AXIS2_PLACEMENT_3D ( 'NONE', #2586, #21079, #23670 ) ;
#22387=CARTESIAN_POINT ( 'NONE',  ( 23.52739736179999852, -94.89419905519999077, -6.742685077560000018 ) ) ;
#22388=AXIS2_PLACEMENT_3D ( 'NONE', #2527, #18101, #22627 ) ;
#22391=CARTESIAN_POINT ( 'NONE',  ( 11.75050204837996048, -98.73470957942969051, 14.28466904018460504 ) ) ;
#22392=CARTESIAN_POINT ( 'NONE',  ( -17.18418019329581981, -97.30182645328051194, 10.80309787203176697 ) ) ;
#22394=B_SPLINE_CURVE_WITH_KNOTS ( 'NONE', 3,
 ( #23892, #10047, #8429, #1341, #17332, #5834, #3381, #3795, #1620, #5691, #12246, #10457, #1482, #21423, #21158, #14980, #23605 ),
 .UNSPECIFIED., .F., .F.,
 ( 4, 2, 2, 1, 1, 1, 1, 1, 2, 2, 4 ),
 ( 0.000000000000000000, 0.2500000000000329181, 0.3750000000000496270, 0.4375000000000587863, 0.4687500000000633937, 0.4843750000000668354, 0.4921875000000687783, 0.4960937500000701106, 0.4980468750000695555, 0.5000000000000690559, 1.000000000000000000 ),
 .UNSPECIFIED. ) ;
#22395=CARTESIAN_POINT ( 'NONE',  ( -23.49132717730000053, -93.00000000000000000, -19.26887671769999955 ) ) ;
#22396=CARTESIAN_POINT ( 'NONE',  ( -5.531648500956975134, -100.7167551761413620, 16.12067131280068821 ) ) ;
#22397=CARTESIAN_POINT ( 'NONE',  ( -12.70399662470000024, -100.4071172650000108, -10.97916378790000103 ) ) ;
#22404=DIRECTION ( 'NONE',  ( 0.000000000000000000, -1.000000000000000000, 0.000000000000000000 ) ) ;
#22407=CARTESIAN_POINT ( 'NONE',  ( -18.27190991239673679, -94.89419557768216862, 16.28310526143894776 ) ) ;
#22409=VERTEX_POINT ( 'NONE', #2962 ) ;
#22411=AXIS2_PLACEMENT_3D ( 'NONE', #24572, #24871, #19898 ) ;
#22414=CARTESIAN_POINT ( 'NONE',  ( 21.36417435310000101, -94.15497231989999705, 13.67389954769999960 ) ) ;
#22415=CARTESIAN_POINT ( 'NONE',  ( -15.50938051129999984, -101.3150705480000084, 4.855933523060000034 ) ) ;
#22416=VERTEX_POINT ( 'NONE', #22478 ) ;
#22417=CARTESIAN_POINT ( 'NONE',  ( 16.49890011910140331, -94.79581646409930329, 16.97758076399984617 ) ) ;
#22419=EDGE_CURVE ( 'NONE', #19835, #5829, #11225, .T. ) ;
#22421=CARTESIAN_POINT ( 'NONE',  ( 12.07615687260000037, -101.1292389600000092, -9.727384960349999332 ) ) ;
#22422=CARTESIAN_POINT ( 'NONE',  ( -13.23807356550000058, -93.85715850769999236, -21.09154035150000084 ) ) ;
#22423=DIRECTION ( 'NONE',  ( 1.000000000000000000, 0.000000000000000000, 0.000000000000000000 ) ) ;
#22425=DIRECTION ( 'NONE',  ( 1.000000000000000000, 0.000000000000000000, 0.000000000000000000 ) ) ;
#22426=B_SPLINE_CURVE_WITH_KNOTS ( 'NONE', 3,
 ( #13487, #22396, #11439, #27062, #20494, #275, #9117, #13785, #18018, #26916, #20345, #15818, #22687, #13640, #22548, #17581, #14504, #20800 ),
 .UNSPECIFIED., .F., .F.,
 ( 4, 2, 2, 2, 1, 1, 1, 1, 2, 2, 4 ),
 ( 0.000000000000000000, 0.2500000000000132672, 0.3750000000000190958, 0.4375000000000223710, 0.4687500000000239808, 0.4843750000000250910, 0.4921875000000259792, 0.4960937500000274225, 0.4980468750000278666, 0.5000000000000283107, 1.000000000000000000 ),
 .UNSPECIFIED. ) ;
#22431=CARTESIAN_POINT ( 'NONE',  ( -2.707548242715575260, -100.1989206112474733, -17.50807487101777227 ) ) ;
#22437=CARTESIAN_POINT ( 'NONE',  ( -7.384731607069999981, -94.63960343449998902, -22.55849074379999664 ) ) ;
#22439=CARTESIAN_POINT ( 'NONE',  ( -24.39543497051741738, -92.52048598158059178, -18.30609232284913190 ) ) ;
#22444=DIRECTION ( 'NONE',  ( 1.000000000000000000, 0.000000000000000000, 0.000000000000000000 ) ) ;
#22449=CARTESIAN_POINT ( 'NONE',  ( 17.98420307009999775, -100.0012764430000090, 1.149933891269999897 ) ) ;
#22453=VERTEX_POINT ( 'NONE', #24808 ) ;
#22454=AXIS2_PLACEMENT_3D ( 'NONE', #12651, #10592, #6253 ) ;
#22455=CARTESIAN_POINT ( 'NONE',  ( 14.93031796050000004, -95.36050459580000904, 17.28030220389999982 ) ) ;
#22457=B_SPLINE_CURVE_WITH_KNOTS ( 'NONE', 3,
 ( #4324, #28642, #17735, #4768, #28783, #2596 ),
 .UNSPECIFIED., .F., .F.,
 ( 4, 2, 4 ),
 ( 0.000000000000000000, 0.5000000000000000000, 1.000000000000000000 ),
 .UNSPECIFIED. ) ;
#22458=CARTESIAN_POINT ( 'NONE',  ( 8.915186176627273085, -94.60934249679789332, -23.38371009848104976 ) ) ;
#22464=CARTESIAN_POINT ( 'NONE',  ( 6.962673402130000078, -92.84292488370000740, -28.64060064759999946 ) ) ;
#22469=CARTESIAN_POINT ( 'NONE',  ( -16.58866213250000143, -92.84298581140001261, 21.51064311520000061 ) ) ;
#22470=CARTESIAN_POINT ( 'NONE',  ( 0.3059185938709999553, -101.1889999979999999, 14.72672055670000013 ) ) ;
#22472=FACE_OUTER_BOUND ( 'NONE', #17201, .T. ) ;
#22476=CARTESIAN_POINT ( 'NONE',  ( 0.1603605168660000024, -101.1030539030000028, -15.43647320760000063 ) ) ;
#22478=CARTESIAN_POINT ( 'NONE',  ( -22.27191869549999836, -94.59276292389999696, -8.381623179300000004 ) ) ;
#22483=ADVANCED_FACE ( 'NONE', ( #21284 ), #27434, .T. ) ;
#22488=ORIENTED_EDGE ( 'NONE', *, *, #16364, .F. ) ;
#22494=CARTESIAN_POINT ( 'NONE',  ( -7.109873676839999490, -101.0147083550000104, 13.82755951569999908 ) ) ;
#22499=AXIS2_PLACEMENT_3D ( 'NONE', #22860, #10941, #4272 ) ;
#22501=CARTESIAN_POINT ( 'NONE',  ( 7.994803016720000599, -99.33439196809999316, 16.09261115110000162 ) ) ;
#22513=CARTESIAN_POINT ( 'NONE',  ( -29.86363316589999783, -111.0000000000000000, 0.3450520984299999538 ) ) ;
#22515=CARTESIAN_POINT ( 'NONE',  ( 27.48096935534069019, -93.08384138313874701, 9.598179995941348963 ) ) ;
#22517=CARTESIAN_POINT ( 'NONE',  ( -29.74766882723250561, -92.84927079009166562, 6.732478952539187489 ) ) ;
#22530=CARTESIAN_POINT ( 'NONE',  ( 16.52251354239999870, -99.77922884479998800, 4.576493590060000116 ) ) ;
#22534=CARTESIAN_POINT ( 'NONE',  ( -15.43774787200000098, -99.62155223620000299, -8.682365224729998943 ) ) ;
#22535=VERTEX_POINT ( 'NONE', #28541 ) ;
#22537=CYLINDRICAL_SURFACE ( 'NONE', #13219, 0.8000000000000008216 ) ;
#22541=CARTESIAN_POINT ( 'NONE',  ( 0.000000000000000000, -92.50000000000000000, 29.91857981989999971 ) ) ;
#22542=CARTESIAN_POINT ( 'NONE',  ( 23.54313657470000010, -94.98812477599999227, -6.784142499889999733 ) ) ;
#22544=CARTESIAN_POINT ( 'NONE',  ( -19.43609242099999790, -92.50000000000000000, -23.50506990850000122 ) ) ;
#22545=CARTESIAN_POINT ( 'NONE',  ( -17.56540178540820918, -95.86369604245908249, 13.50288865853636366 ) ) ;
#22546=EDGE_LOOP ( 'NONE', ( #12338, #4533, #7399, #662 ) ) ;
#22548=CARTESIAN_POINT ( 'NONE',  ( -3.128864287929727706, -98.07255008584144207, 20.23552373180469388 ) ) ;
#22549=CARTESIAN_POINT ( 'NONE',  ( -13.32816354210000043, -99.92967571559999840, -11.12411009090000036 ) ) ;
#22550=CYLINDRICAL_SURFACE ( 'NONE', #10392, 15.99999999999999645 ) ;
#22555=CARTESIAN_POINT ( 'NONE',  ( 26.34145817392794342, -92.82334897396464157, -15.37457621828394672 ) ) ;
#22556=EDGE_LOOP ( 'NONE', ( #8658, #25532, #6044, #15523 ) ) ;
#22559=CARTESIAN_POINT ( 'NONE',  ( -1.283023294879999998, -101.1889999979999999, -16.20107482390000087 ) ) ;
#22560=CARTESIAN_POINT ( 'NONE',  ( 1.375203621220000061, -94.98812769030000425, 24.46248643120000210 ) ) ;
#22561=COLOUR_RGB ( '', 0.09019608, 0.27058824, 0.51372549) ;
#22562=CARTESIAN_POINT ( 'NONE',  ( 8.039511664659999113, -92.65193295299998510, 26.91643347890000015 ) ) ;
#22574=CARTESIAN_POINT ( 'NONE',  ( -23.69410943009695103, -94.52419745024906206, -3.934991533140109077 ) ) ;
#22575=ORIENTED_EDGE ( 'NONE', *, *, #17966, .T. ) ;
#22577=CARTESIAN_POINT ( 'NONE',  ( -16.74373768950000141, -99.87169021820000125, 2.814689237420000101 ) ) ;
#22580=CARTESIAN_POINT ( 'NONE',  ( -11.73626238637177899, -94.71481465629089769, -21.34524630996246586 ) ) ;
#22585=ADVANCED_FACE ( 'NONE', ( #22145 ), #6146, .F. ) ;
#22586=CARTESIAN_POINT ( 'NONE',  ( -13.18687770350000044, -93.32822605769999313, -23.58441588660000221 ) ) ;
#22587=AXIS2_PLACEMENT_3D ( 'NONE', #19480, #8831, #9392 ) ;
#22590=CARTESIAN_POINT ( 'NONE',  ( 15.69315028655411659, -101.4304678898235039, 3.891722348338785942 ) ) ;
#22591=CARTESIAN_POINT ( 'NONE',  ( -15.42268960139999834, -101.6484611540000031, 4.259183661159999801 ) ) ;
#22596=CARTESIAN_POINT ( 'NONE',  ( 9.525697108589946893, -93.08996184747134350, 27.45793313423234139 ) ) ;
#22597=ORIENTED_EDGE ( 'NONE', *, *, #8750, .F. ) ;
#22606=CARTESIAN_POINT ( 'NONE',  ( 4.127715330941034821, -93.15741110422700899, -28.33879718941593495 ) ) ;
#22608=CARTESIAN_POINT ( 'NONE',  ( -19.02290610980000096, -97.53593570510001598, 6.397707897409999234 ) ) ;
#22609=FACE_OUTER_BOUND ( 'NONE', #21654, .T. ) ;
#22612=CARTESIAN_POINT ( 'NONE',  ( 7.085361681160000202, -92.56168957700000988, -28.78018708169999940 ) ) ;
#22618=DIRECTION ( 'NONE',  ( 0.000000000000000000, -1.000000000000000000, 0.000000000000000000 ) ) ;
#22621=CARTESIAN_POINT ( 'NONE',  ( -2.903039748510000351, -94.98812477769999418, 23.52859306979999943 ) ) ;
#22623=CYLINDRICAL_SURFACE ( 'NONE', #9580, 20.64285714289999873 ) ;
#22625=CARTESIAN_POINT ( 'NONE',  ( 2.162714451969999821E-13, -111.0000000000000000, 6.000533403490000639E-12 ) ) ;
#22627=DIRECTION ( 'NONE',  ( 1.000000000000000000, 0.000000000000000000, 0.000000000000000000 ) ) ;
#22628=B_SPLINE_CURVE_WITH_KNOTS ( 'NONE', 3,
 ( #27267, #2794, #6719, #28 ),
 .UNSPECIFIED., .F., .F.,
 ( 4, 4 ),
 ( -0.1274251584810000004, -1.776356839400250465E-15 ),
 .UNSPECIFIED. ) ;
#22634=VERTEX_POINT ( 'NONE', #27674 ) ;
#22637=CARTESIAN_POINT ( 'NONE',  ( 20.48611068019999948, -93.36531860659999893, 16.28991794210000066 ) ) ;
#22639=CARTESIAN_POINT ( 'NONE',  ( -7.421872664780000406, -100.8815367389999977, 13.80620562409999863 ) ) ;
#22641=CARTESIAN_POINT ( 'NONE',  ( -12.52509995851851166, -101.6297509123138099, -9.979436452931571111 ) ) ;
#22645=CARTESIAN_POINT ( 'NONE',  ( 7.813212629879998872, -99.08067767480000043, 16.22119575690000204 ) ) ;
#22650=CARTESIAN_POINT ( 'NONE',  ( 11.33780648110000122, -100.8733988930000010, -10.89600415129999966 ) ) ;
#22652=CARTESIAN_POINT ( 'NONE',  ( 15.88351635808362516, -94.85336603632588037, 17.26556729870110729 ) ) ;
#22656=CARTESIAN_POINT ( 'NONE',  ( 16.41935458950000282, -111.0000000000000000, 3.555952033500000109 ) ) ;
#22657=FACE_OUTER_BOUND ( 'NONE', #27921, .T. ) ;
#22658=CARTESIAN_POINT ( 'NONE',  ( 0.000000000000000000, -111.0000000000000000, 0.000000000000000000 ) ) ;
#22662=CARTESIAN_POINT ( 'NONE',  ( 22.50364785879999729, -95.66919271840001215, -0.5489143750859999393 ) ) ;
#22664=CARTESIAN_POINT ( 'NONE',  ( -19.16019836899999618, -92.50000000000000000, 22.97842938279999814 ) ) ;
#22665=CARTESIAN_POINT ( 'NONE',  ( 19.57843399940000140, -94.59276292389999696, 13.52682119470000011 ) ) ;
#22666=DIRECTION ( 'NONE',  ( 1.000000000000000000, 0.000000000000000000, 0.000000000000000000 ) ) ;
#22670=CARTESIAN_POINT ( 'NONE',  ( 16.30068969910000121, -100.0496341300000154, 4.508739917940000730 ) ) ;
#22673=CARTESIAN_POINT ( 'NONE',  ( -17.92518616159999922, -98.60488091089999330, -8.251865930899999313 ) ) ;
#22675=CARTESIAN_POINT ( 'NONE',  ( 8.456806930322576576, -92.64884742711174681, 29.30416004283850739 ) ) ;
#22678=CARTESIAN_POINT ( 'NONE',  ( -11.77131553929999974, -101.2010924020000004, -9.714008462309999814 ) ) ;
#22680=CARTESIAN_POINT ( 'NONE',  ( 23.14927425619999823, -94.18458606750000683, -7.514520311420000098 ) ) ;
#22683=CARTESIAN_POINT ( 'NONE',  ( 14.04239374870000212, -98.93445099689999722, -12.32916220780000138 ) ) ;
#22684=B_SPLINE_SURFACE_WITH_KNOTS ( 'NONE', 5, 5, ( 
 ( #15641, #9534, #26746, #2563, #18435, #24542, #13909, #17991, #24696 ),
 ( #11412, #4585, #22364, #2411, #27324, #20172, #6925, #2703, #15790 ),
 ( #4733, #15492, #13311, #9386, #22215, #20313, #9230, #7078, #24842 ),
 ( #18289, #16085, #4881, #4440, #7218, #2262, #16229, #10087, #5738 ),
 ( #7523, #3558, #18872, #20774, #18729, #14343, #829, #7666, #14212 ),
 ( #25430, #27756, #12000, #3286, #12142, #21059, #16666, #25565, #23795 ) ),
 .UNSPECIFIED., .F., .F., .F.,
 ( 6, 6 ),
 ( 6, 3, 6 ),
 ( 4.057198812540000255, 5.368803751829999804 ),
 ( 0.000000000000000000, 0.2500000000000000000, 0.5000000000000000000 ),
 .UNSPECIFIED. ) ;
#22687=CARTESIAN_POINT ( 'NONE',  ( -3.141019993213900463, -98.08323606068540812, 20.21953806862122249 ) ) ;
#22688=CARTESIAN_POINT ( 'NONE',  ( -13.16264660049999868, -99.58396362730000817, -11.32285879039999799 ) ) ;
#22696=CARTESIAN_POINT ( 'NONE',  ( -23.24818410940000035, -93.00000000000000000, -18.83197690249999923 ) ) ;
#22699=CARTESIAN_POINT ( 'NONE',  ( -4.683949502529999975, -99.57131247770000471, 16.77925173899999933 ) ) ;
#22700=CARTESIAN_POINT ( 'NONE',  ( 8.002737880409998894, -92.75793418959999315, 27.16184970260000142 ) ) ;
#22713=CARTESIAN_POINT ( 'NONE',  ( 7.584268328590000330, -101.6484612600000048, 14.08825304710000026 ) ) ;
#22720=CARTESIAN_POINT ( 'NONE',  ( 13.91983387960000051, -99.74726900420000675, -10.02745453350000027 ) ) ;
#22723=ORIENTED_EDGE ( 'NONE', *, *, #6214, .F. ) ;
#22726=DIRECTION ( 'NONE',  ( -0.9037419867099893978, 0.000000000000000000, 0.4280775881279951789 ) ) ;
#22730=CARTESIAN_POINT ( 'NONE',  ( 23.58466923419999972, -94.98812477769999418, -2.405350023570000051 ) ) ;
#22732=CARTESIAN_POINT ( 'NONE',  ( 15.81801911784844172, -101.2145573445017703, 4.083609699486570932 ) ) ;
#22734=EDGE_LOOP ( 'NONE', ( #13403, #14812, #2308, #24539 ) ) ;
#22741=CARTESIAN_POINT ( 'NONE',  ( 9.610902359217210034, -93.08494104690983306, 27.46771387074625537 ) ) ;
#22746=DIRECTION ( 'NONE',  ( -0.8386955343508021299, 0.000000000000000000, -0.5446005881928723813 ) ) ;
#22747=VERTEX_POINT ( 'NONE', #24549 ) ;
#22751=CARTESIAN_POINT ( 'NONE',  ( -25.71126894084192216, -93.01584921936724015, -6.102654395426379885 ) ) ;
#22752=CARTESIAN_POINT ( 'NONE',  ( -20.27480073103475178, -94.70873045429671322, 12.26046566542698102 ) ) ;
#22753=CARTESIAN_POINT ( 'NONE',  ( -19.71577987869999760, -96.53868972700000484, 8.226325169349999911 ) ) ;
#22754=EDGE_CURVE ( 'NONE', #16297, #26053, #17167, .T. ) ;
#22763=VERTEX_POINT ( 'NONE', #22813 ) ;
#22767=VERTEX_POINT ( 'NONE', #15645 ) ;
#22768=CARTESIAN_POINT ( 'NONE',  ( -17.62778457210000127, -98.60479852289999769, 8.869694630919999767 ) ) ;
#22775=AXIS2_PLACEMENT_3D ( 'NONE', #19443, #8360, #17265 ) ;
#22778=CARTESIAN_POINT ( 'NONE',  ( 11.15108825559999950, -100.9197081840000010, -10.94438638200000113 ) ) ;
#22779=CIRCLE ( 'NONE', #16228, 20.64285714289999873 ) ;
#22780=EDGE_CURVE ( 'NONE', #7941, #21723, #10963, .T. ) ;
#22781=CARTESIAN_POINT ( 'NONE',  ( 10.14993553289999895, -99.56347846010000069, 14.32348655080000022 ) ) ;
#22786=CARTESIAN_POINT ( 'NONE',  ( -7.478713340969999734, -101.1191090859999946, 14.48799200630000072 ) ) ;
#22789=CARTESIAN_POINT ( 'NONE',  ( 7.579179873580000226, -101.3235621230000021, 13.98627925510000125 ) ) ;
#22790=ORIENTED_EDGE ( 'NONE', *, *, #11670, .F. ) ;
#22797=CARTESIAN_POINT ( 'NONE',  ( 11.83254868180000052, -101.2490009469999990, -10.89135062169999912 ) ) ;
#22799=CARTESIAN_POINT ( 'NONE',  ( -20.98832407942702005, -96.92941680200577537, -6.663699877346700440 ) ) ;
#22807=VERTEX_POINT ( 'NONE', #27888 ) ;
#22811=CARTESIAN_POINT ( 'NONE',  ( 22.48942068090000035, -95.85308664759999431, -0.6733658741689999561 ) ) ;
#22813=CARTESIAN_POINT ( 'NONE',  ( 14.40601943769999949, -92.50000000000000000, 26.88338899689999906 ) ) ;
#22816=CARTESIAN_POINT ( 'NONE',  ( -17.55776206427488972, -93.39299082544175690, -21.35661493576082037 ) ) ;
#22818=ADVANCED_FACE ( 'NONE', ( #5177 ), #14059, .T. ) ;
#22822=CARTESIAN_POINT ( 'NONE',  ( -17.97171875919999806, -98.69238697859999832, -8.234156820420000855 ) ) ;
#22825=CARTESIAN_POINT ( 'NONE',  ( -30.49344753122725038, -92.49999999999998579, 0.6399496674373281735 ) ) ;
#22839=CARTESIAN_POINT ( 'NONE',  ( -13.18661234450000030, -92.50000000000000000, 26.85581265420000108 ) ) ;
#22841=CARTESIAN_POINT ( 'NONE',  ( 15.98230758980000132, -101.4309749570000037, 2.416262475850000424 ) ) ;
#22848=CARTESIAN_POINT ( 'NONE',  ( -3.552756184370000181, -98.29702512609999587, 18.77134648699999886 ) ) ;
#22849=CARTESIAN_POINT ( 'NONE',  ( 5.602941559059999577, -93.28216931219999708, 26.66162101379999783 ) ) ;
#22850=ORIENTED_EDGE ( 'NONE', *, *, #4474, .T. ) ;
#22852=CARTESIAN_POINT ( 'NONE',  ( -11.25326567110000120, -94.84395216780001192, -20.59896464009999661 ) ) ;
#22858=CIRCLE ( 'NONE', #25190, 10.00000000000000000 ) ;
#22860=CARTESIAN_POINT ( 'NONE',  ( 0.000000000000000000, -92.50000000000000000, 29.91857981989999971 ) ) ;
#22867=DIRECTION ( 'NONE',  ( 0.000000000000000000, 1.000000000000000000, 0.000000000000000000 ) ) ;
#22871=VERTEX_POINT ( 'NONE', #5602 ) ;
#22872=CARTESIAN_POINT ( 'NONE',  ( -11.32307664130000013, -92.50000000000000000, 9.421136869679999748 ) ) ;
#22876=CARTESIAN_POINT ( 'NONE',  ( -13.10651597679999902, -92.87496451630001104, -23.83817055480000136 ) ) ;
#22880=CARTESIAN_POINT ( 'NONE',  ( 16.63653260355367891, -100.1406256088351796, 4.325926551192202929 ) ) ;
#22881=CARTESIAN_POINT ( 'NONE',  ( 13.82610735156381487, -99.76647888977575462, -10.42913651524955121 ) ) ;
#22883=CARTESIAN_POINT ( 'NONE',  ( -1.315109685649999971, -92.50000000000000000, -30.47163412939999816 ) ) ;
#22886=TOROIDAL_SURFACE ( 'NONE', #12602, 5.500000000000000000, 0.5000000000000000000 ) ;
#22891=CARTESIAN_POINT ( 'NONE',  ( 23.96368475870000125, -93.00000000000000000, 8.717328305520000598 ) ) ;
#22896=EDGE_LOOP ( 'NONE', ( #13714, #8767, #22308, #21371 ) ) ;
#22901=CIRCLE ( 'NONE', #17764, 30.50000000000000000 ) ;
#22918=CARTESIAN_POINT ( 'NONE',  ( -18.24886543000000216, -94.80026553199999739, 16.23660559380000024 ) ) ;
#22923=EDGE_CURVE ( 'NONE', #1616, #23041, #2966, .T. ) ;
#22924=TOROIDAL_SURFACE ( 'NONE', #26622, 15.50000000000000000, 0.5000000000000000000 ) ;
#22933=CARTESIAN_POINT ( 'NONE',  ( 17.49193124830000201, -96.07623110170000302, 14.96946685699999868 ) ) ;
#22936=CARTESIAN_POINT ( 'NONE',  ( 16.54057195469999897, -94.89197151650000706, 16.94454422099999746 ) ) ;
#22939=CARTESIAN_POINT ( 'NONE',  ( -10.46188072746246434, -93.89463536436431923, -23.23764647000281869 ) ) ;
#22941=CARTESIAN_POINT ( 'NONE',  ( 7.235323095100000046, -101.2527939679999918, 13.36104842480000165 ) ) ;
#22943=FACE_OUTER_BOUND ( 'NONE', #3107, .T. ) ;
#22946=CARTESIAN_POINT ( 'NONE',  ( 11.64683525529999919, -98.24904979019999018, -15.38395215939999972 ) ) ;
#22947=VERTEX_POINT ( 'NONE', #17091 ) ;
#22949=CARTESIAN_POINT ( 'NONE',  ( 0.000000000000000000, -101.1889999979999999, 0.000000000000000000 ) ) ;
#22950=AXIS2_PLACEMENT_3D ( 'NONE', #4045, #27967, #16749 ) ;
#22953=CARTESIAN_POINT ( 'NONE',  ( 14.16035994550885313, -95.68935540834247888, 17.33364939168795971 ) ) ;
#22955=CARTESIAN_POINT ( 'NONE',  ( 11.86655840719999944, -101.3150700380000018, -11.10431293650000129 ) ) ;
#22959=ORIENTED_EDGE ( 'NONE', *, *, #2317, .F. ) ;
#22963=EDGE_CURVE ( 'NONE', #11437, #9289, #3964, .T. ) ;
#22970=DIRECTION ( 'NONE',  ( 0.8531997950690719534, 0.000000000000000000, -0.5215842306800441142 ) ) ;
#22973=CARTESIAN_POINT ( 'NONE',  ( 6.114061450880000415, -92.50000000000000000, -13.40104985119999981 ) ) ;
#22975=CARTESIAN_POINT ( 'NONE',  ( 13.12517053680000068, -111.0000000000000000, 27.53143473160000099 ) ) ;
#22976=CARTESIAN_POINT ( 'NONE',  ( 0.2593320631483060357, -101.4728631013045970, -16.13356699571328789 ) ) ;
#22979=CARTESIAN_POINT ( 'NONE',  ( 23.76251265679999847, -94.45168166330000759, -7.425192885069999527 ) ) ;
#22980=CARTESIAN_POINT ( 'NONE',  ( -11.25326567110000120, -94.84395216780001192, -20.59896464009999661 ) ) ;
#22981=CARTESIAN_POINT ( 'NONE',  ( 23.76679749976556266, -92.71619979444686521, -19.11516032664452780 ) ) ;
#22986=CIRCLE ( 'NONE', #1573, 16.00000000000000000 ) ;
#22989=VERTEX_POINT ( 'NONE', #4261 ) ;
#22991=ORIENTED_EDGE ( 'NONE', *, *, #21568, .T. ) ;
#22994=VECTOR ( 'NONE', #20646, 1000.000000000000000 ) ;
#22995=CYLINDRICAL_SURFACE ( 'NONE', #14407, 0.7499999999999996669 ) ;
#22996=CARTESIAN_POINT ( 'NONE',  ( 1.316321141829999819, -94.80026165740000010, 24.39090473970000161 ) ) ;
#22998=CARTESIAN_POINT ( 'NONE',  ( -11.27245849040000003, -95.14589738820001230, -21.35309096379999971 ) ) ;
#23000=CARTESIAN_POINT ( 'NONE',  ( -18.94992598540000017, -92.68283714880000446, -20.51038952960000117 ) ) ;
#23001=CARTESIAN_POINT ( 'NONE',  ( 4.146788479588165544, -93.04141874247781629, 28.17739296888928280 ) ) ;
#23004=CARTESIAN_POINT ( 'NONE',  ( 3.166345171159999694, -93.00000000000000000, -25.30265318609999881 ) ) ;
#23005=CARTESIAN_POINT ( 'NONE',  ( 21.75659477429999811, -92.50000000000000000, -13.30039788230000042 ) ) ;
#23006=VERTEX_POINT ( 'NONE', #13579 ) ;
#23007=EDGE_CURVE ( 'NONE', #27814, #12485, #1969, .T. ) ;
#23008=CARTESIAN_POINT ( 'NONE',  ( 7.491164759823046637, -101.2404586314123520, 13.91530727530272493 ) ) ;
#23014=CARTESIAN_POINT ( 'NONE',  ( -16.03245889869999985, -100.9307694150000003, 3.138388912410000398 ) ) ;
#23017=EDGE_LOOP ( 'NONE', ( #24671, #12583, #19905, #4707 ) ) ;
#23026=CARTESIAN_POINT ( 'NONE',  ( 15.78742501808848608, -101.2637735887499986, 4.048283812879304833 ) ) ;
#23040=CARTESIAN_POINT ( 'NONE',  ( -6.000841078150000563, -101.4334236450000049, 14.90466326349999981 ) ) ;
#23041=VERTEX_POINT ( 'NONE', #13131 ) ;
#23043=DIRECTION ( 'NONE',  ( 0.000000000000000000, 1.000000000000000000, 0.000000000000000000 ) ) ;
#23044=EDGE_CURVE ( 'NONE', #10772, #21528, #19591, .T. ) ;
#23046=ORIENTED_EDGE ( 'NONE', *, *, #27912, .F. ) ;
#23049=CARTESIAN_POINT ( 'NONE',  ( -20.20035200647939888, -94.89195677473493618, 12.35537660001062754 ) ) ;
#23055=CARTESIAN_POINT ( 'NONE',  ( 18.35053352010000083, -98.58303758080000989, 3.544495826009999906 ) ) ;
#23061=CARTESIAN_POINT ( 'NONE',  ( -16.14562817639999892, -111.0000000000000000, 4.458832895280000486 ) ) ;
#23063=ORIENTED_EDGE ( 'NONE', *, *, #8435, .T. ) ;
#23064=CARTESIAN_POINT ( 'NONE',  ( -16.63714921780000111, -99.82961947799999791, 6.686300942209999931 ) ) ;
#23066=CARTESIAN_POINT ( 'NONE',  ( 0.3872054374930000153, -99.92967571559999840, -17.35614705709999939 ) ) ;
#23069=CARTESIAN_POINT ( 'NONE',  ( -0.1779554536940000098, -101.6484611540000031, -15.99901033990000165 ) ) ;
#23070=ORIENTED_EDGE ( 'NONE', *, *, #17966, .F. ) ;
#23076=CARTESIAN_POINT ( 'NONE',  ( 8.185346967789998374, -111.0000000000000000, 14.03998109830000018 ) ) ;
#23078=EDGE_CURVE ( 'NONE', #3331, #8764, #4283, .T. ) ;
#23080=CARTESIAN_POINT ( 'NONE',  ( 6.308882621530000456, -93.00000000000000000, -29.19167084780000110 ) ) ;
#23081=B_SPLINE_CURVE_WITH_KNOTS ( 'NONE', 3,
 ( #15279, #24201, #4234, #13108, #22020, #19814, #23629, #12530, #14730, #18231, #2653, #6572, #185, #24346, #26981, #2203, #26835, #6724 ),
 .UNSPECIFIED., .F., .F.,
 ( 4, 2, 2, 2, 1, 1, 1, 1, 2, 2, 4 ),
 ( 0.000000000000000000, 0.2499999999999109601, 0.3749999999998656630, 0.4374999999998440137, 0.4687499999998328004, 0.4843749999998279154, 0.4921874999998258615, 0.4960937499998256395, 0.4980468749998255285, 0.4999999999998253619, 1.000000000000000000 ),
 .UNSPECIFIED. ) ;
#23083=CARTESIAN_POINT ( 'NONE',  ( 7.577553826990000019, -101.4254869589999970, 14.05661196390000001 ) ) ;
#23086=CARTESIAN_POINT ( 'NONE',  ( -28.63163567490000005, -92.51556042380001088, -2.601810723099999834 ) ) ;
#23087=CARTESIAN_POINT ( 'NONE',  ( 11.63343543059999874, -100.9405345029999950, -10.90407306190000014 ) ) ;
#23088=VERTEX_POINT ( 'NONE', #14452 ) ;
#23091=CARTESIAN_POINT ( 'NONE',  ( 11.44042105569999990, -101.2530993000000024, -9.998588429439999814 ) ) ;
#23099=DIRECTION ( 'NONE',  ( -0.7858270635388553416, 0.000000000000000000, 0.6184463001828854889 ) ) ;
#23100=ORIENTED_EDGE ( 'NONE', *, *, #9769, .F. ) ;
#23101=CARTESIAN_POINT ( 'NONE',  ( 6.468171908630000466, -101.1402801299999936, 13.91008216630000049 ) ) ;
#23104=CARTESIAN_POINT ( 'NONE',  ( -11.30171162149999908, -94.71348074940000572, -20.91579854999999810 ) ) ;
#23107=CARTESIAN_POINT ( 'NONE',  ( -17.60846427396887393, -93.38554229068824952, -21.34790020497966267 ) ) ;
#23109=ORIENTED_EDGE ( 'NONE', *, *, #12030, .T. ) ;
#23111=CARTESIAN_POINT ( 'NONE',  ( -18.69985100839999959, -93.00000000000000000, 22.78328762010000119 ) ) ;
#23113=CARTESIAN_POINT ( 'NONE',  ( -30.40304712095338502, -92.82529299094046848, 2.429966744979142224 ) ) ;
#23114=EDGE_LOOP ( 'NONE', ( #11932, #5732, #2263, #16512 ) ) ;
#23116=CARTESIAN_POINT ( 'NONE',  ( 0.6129623820366252307, -100.5798851008108414, -16.82649590739602630 ) ) ;
#23117=CARTESIAN_POINT ( 'NONE',  ( -25.37284092810000047, -101.1889999979999999, 2.543411731580000001 ) ) ;
#23122=CARTESIAN_POINT ( 'NONE',  ( -17.64295153049999954, -98.69230457299998704, 8.917116780599998904 ) ) ;
#23123=CARTESIAN_POINT ( 'NONE',  ( 6.114061450890000415, -92.50000000000000000, -13.40104985119999981 ) ) ;
#23126=ORIENTED_EDGE ( 'NONE', *, *, #11306, .T. ) ;
#23128=B_SPLINE_CURVE_WITH_KNOTS ( 'NONE', 5,
 ( #8706, #26659, #6846, #24322, #10, #10737, #17774, #13235, #6392 ),
 .UNSPECIFIED., .F., .F.,
 ( 6, 3, 6 ),
 ( 0.000000000000000000, 0.3499052706296189585, 1.000000000000000000 ),
 .UNSPECIFIED. ) ;
#23131=CARTESIAN_POINT ( 'NONE',  ( -2.412598911559999948, -96.96081043750000106, 20.83962799120000042 ) ) ;
#23132=CARTESIAN_POINT ( 'NONE',  ( 1.631270863969999985, -94.59275870510001027, 23.74088086560000121 ) ) ;
#23138=CARTESIAN_POINT ( 'NONE',  ( 0.000000000000000000, -94.59276292389999696, 0.000000000000000000 ) ) ;
#23145=FACE_OUTER_BOUND ( 'NONE', #7112, .T. ) ;
#23152=CARTESIAN_POINT ( 'NONE',  ( -15.32770678129999986, -100.9616777990000003, 2.981256516259999767 ) ) ;
#23158=CARTESIAN_POINT ( 'NONE',  ( 23.32816514950000197, -93.91547326110000427, -8.285286069360001449 ) ) ;
#23159=ORIENTED_EDGE ( 'NONE', *, *, #5821, .T. ) ;
#23162=DIRECTION ( 'NONE',  ( 0.000000000000000000, -1.000000000000000000, 0.000000000000000000 ) ) ;
#23165=CARTESIAN_POINT ( 'NONE',  ( 16.40445051276553912, -100.4103893716901865, 4.355817310233436324 ) ) ;
#23178=CARTESIAN_POINT ( 'NONE',  ( -6.083378538189999851, -101.1716782080000030, 14.51061107299999975 ) ) ;
#23179=ORIENTED_EDGE ( 'NONE', *, *, #3223, .T. ) ;
#23185=ADVANCED_FACE ( 'NONE', ( #8520 ), #21785, .F. ) ;
#23189=PLANE ( 'NONE',  #7896 ) ;
#23190=CARTESIAN_POINT ( 'NONE',  ( 15.79772739633221157, -101.6174239712916432, 2.678369929592316456 ) ) ;
#23191=DIRECTION ( 'NONE',  ( 0.01112221585590945742, 0.000000000000000000, 0.9999381462442837876 ) ) ;
#23197=DIRECTION ( 'NONE',  ( 0.000000000000000000, 1.000000000000000000, 0.000000000000000000 ) ) ;
#23211=DIRECTION ( 'NONE',  ( 0.4794255386042041156, 0.000000000000000000, 0.8775825618903722036 ) ) ;
#23220=CARTESIAN_POINT ( 'NONE',  ( -23.91694143229999980, -93.67869433890000153, -7.293500637750000237 ) ) ;
#23222=CARTESIAN_POINT ( 'NONE',  ( 11.34550471930000093, -98.29702512450000995, -15.37091565870000132 ) ) ;
#23223=ORIENTED_EDGE ( 'NONE', *, *, #14883, .T. ) ;
#23227=CARTESIAN_POINT ( 'NONE',  ( -17.07087492460914291, -92.82044061136174662, 25.27519173372845174 ) ) ;
#23234=AXIS2_PLACEMENT_3D ( 'NONE', #16415, #12028, #25459 ) ;
#23237=CARTESIAN_POINT ( 'NONE',  ( 7.060623116049999481, -101.3256027139999986, 14.25378149400000005 ) ) ;
#23238=CARTESIAN_POINT ( 'NONE',  ( 13.30084296762267293, -95.75133629986981987, -18.44067507113092574 ) ) ;
#23251=DIRECTION ( 'NONE',  ( 1.000000000000000000, 0.000000000000000000, 0.000000000000000000 ) ) ;
#23255=CARTESIAN_POINT ( 'NONE',  ( 0.6119498907216414096, -100.5550990433582541, -16.84632490533061855 ) ) ;
#23258=CARTESIAN_POINT ( 'NONE',  ( 13.15187379876893559, -92.89593097429261093, 27.51868946396341542 ) ) ;
#23259=CARTESIAN_POINT ( 'NONE',  ( -12.60062440519999960, -94.64125147549999895, -21.54742969149999965 ) ) ;
#23262=CARTESIAN_POINT ( 'NONE',  ( 13.68846061079999998, -95.60035679230000483, -17.92298507690000164 ) ) ;
#23263=CARTESIAN_POINT ( 'NONE',  ( -15.16614058563374989, -101.1716787529999237, 4.188334258669885735 ) ) ;
#23270=EDGE_CURVE ( 'NONE', #22416, #6793, #22327, .T. ) ;
#23276=CARTESIAN_POINT ( 'NONE',  ( -28.36632169019999949, -93.16461275549998788, 1.612349139190000002 ) ) ;
#23278=EDGE_CURVE ( 'NONE', #13014, #4106, #10803, .T. ) ;
#23282=CARTESIAN_POINT ( 'NONE',  ( 0.000000000000000000, -94.59276292389999696, 0.000000000000000000 ) ) ;
#23284=ORIENTED_EDGE ( 'NONE', *, *, #22754, .T. ) ;
#23290=CARTESIAN_POINT ( 'NONE',  ( -16.70751862240000207, -99.92474288910000269, 2.933832141839999963 ) ) ;
#23295=CARTESIAN_POINT ( 'NONE',  ( -7.911012669536270359, -100.3266728694704000, 15.09234432844895046 ) ) ;
#23298=DIRECTION ( 'NONE',  ( 0.000000000000000000, -1.000000000000000000, 0.000000000000000000 ) ) ;
#23307=EDGE_CURVE ( 'NONE', #21547, #19815, #15944, .T. ) ;
#23308=ORIENTED_EDGE ( 'NONE', *, *, #8628, .F. ) ;
#23313=CARTESIAN_POINT ( 'NONE',  ( -5.890277023240000354, -101.2306315440000049, 15.10563561669999899 ) ) ;
#23314=VERTEX_POINT ( 'NONE', #9062 ) ;
#23315=CARTESIAN_POINT ( 'NONE',  ( -3.843858959260458619, -97.05288880177764099, -20.70537388607158391 ) ) ;
#23321=CARTESIAN_POINT ( 'NONE',  ( -14.45392997149999914, -92.99999875040001029, 26.19394095939999900 ) ) ;
#23324=CARTESIAN_POINT ( 'NONE',  ( 16.08037959500000014, -101.3150700380000018, 2.354223078750000031 ) ) ;
#23331=VECTOR ( 'NONE', #14381, 1000.000000000000000 ) ;
#23332=CARTESIAN_POINT ( 'NONE',  ( 23.53302756460000111, -93.00000000000000000, -18.47479450719999861 ) ) ;
#23333=VECTOR ( 'NONE', #13693, 1000.000000000000000 ) ;
#23335=CARTESIAN_POINT ( 'NONE',  ( 6.153546133999999945, -93.00000450890000536, 28.82528558229999760 ) ) ;
#23346=CARTESIAN_POINT ( 'NONE',  ( 6.962669195700001090, -93.00000450890000536, -28.64060852350000275 ) ) ;
#23349=CARTESIAN_POINT ( 'NONE',  ( -13.35118457799999980, -101.4309749570000037, -9.111440644229999108 ) ) ;
#23353=CARTESIAN_POINT ( 'NONE',  ( -7.893993299629999960, -100.5229262450000078, 14.92267151810000136 ) ) ;
#23355=CARTESIAN_POINT ( 'NONE',  ( 7.584268328590000330, -101.1889999979999999, 14.08825304710000026 ) ) ;
#23359=CARTESIAN_POINT ( 'NONE',  ( -23.90121231679999880, -94.07620464550001316, -7.056844240210001118 ) ) ;
#23361=CARTESIAN_POINT ( 'NONE',  ( 10.37409836790000028, -95.71128647580000859, -20.04562559420000412 ) ) ;
#23362=ORIENTED_EDGE ( 'NONE', *, *, #10335, .F. ) ;
#23364=DIRECTION ( 'NONE',  ( 0.000000000000000000, -1.000000000000000000, 0.000000000000000000 ) ) ;
#23366=CARTESIAN_POINT ( 'NONE',  ( -18.24886321460000005, -94.80026206440000180, 16.23660667690000281 ) ) ;
#23367=CARTESIAN_POINT ( 'NONE',  ( -17.13188320504061934, -92.80045754877718878, 25.23390446720919655 ) ) ;
#23368=CARTESIAN_POINT ( 'NONE',  ( 5.273680924649999824, -107.5000000000000000, 9.653408180790000515 ) ) ;
#23372=CARTESIAN_POINT ( 'NONE',  ( 18.08741318713345692, -95.90275958024609793, 14.78486932492663897 ) ) ;
#23375=EDGE_CURVE ( 'NONE', #16619, #22108, #2938, .T. ) ;
#23378=CARTESIAN_POINT ( 'NONE',  ( 13.08001772823451070, -95.36087494481114391, -19.20617372813112311 ) ) ;
#23387=CARTESIAN_POINT ( 'NONE',  ( 8.188637977920000921, -100.9197082849999987, 13.30686163390000054 ) ) ;
#23393=CARTESIAN_POINT ( 'NONE',  ( 0.5678894871162830649, -100.9510322836843272, -16.53366320519699073 ) ) ;
#23395=CARTESIAN_POINT ( 'NONE',  ( 6.185491179879999635, -101.0875971110000080, 14.11315596670000083 ) ) ;
#23396=B_SPLINE_CURVE_WITH_KNOTS ( 'NONE', 3,
 ( #20509, #27220, #18769, #5060, #9994, #27364 ),
 .UNSPECIFIED., .F., .F.,
 ( 4, 2, 4 ),
 ( 0.000000000000000000, 0.5000000000000000000, 1.000000000000000000 ),
 .UNSPECIFIED. ) ;
#23397=CARTESIAN_POINT ( 'NONE',  ( 13.66357347539002731, -92.59055325467724629, 27.26823877034133403 ) ) ;
#23399=CARTESIAN_POINT ( 'NONE',  ( 15.60984783840000034, -101.0640712160000021, 3.941010556740000670 ) ) ;
#23410=AXIS2_PLACEMENT_3D ( 'NONE', #12141, #20915, #25141 ) ;
#23413=AXIS2_PLACEMENT_3D ( 'NONE', #10828, #15500, #19875 ) ;
#23416=CARTESIAN_POINT ( 'NONE',  ( -28.36339762329999914, -93.07693985719998864, 1.604523527660000060 ) ) ;
#23421=CARTESIAN_POINT ( 'NONE',  ( -28.12914522643169590, -93.25521311031921812, 1.335511596251312660 ) ) ;
#23422=ORIENTED_EDGE ( 'NONE', *, *, #3564, .F. ) ;
#23426=CARTESIAN_POINT ( 'NONE',  ( 26.67791892279999999, -92.70565333729999224, -10.13078936369999994 ) ) ;
#23427=AXIS2_PLACEMENT_3D ( 'NONE', #23282, #21511, #19049 ) ;
#23433=CARTESIAN_POINT ( 'NONE',  ( -15.35368226649999990, -101.3957230199999913, 4.453032938229999793 ) ) ;
#23434=CARTESIAN_POINT ( 'NONE',  ( -15.39298286279999850, -100.9658258050000086, 3.068543784489999648 ) ) ;
#23443=EDGE_CURVE ( 'NONE', #1115, #22453, #9896, .T. ) ;
#23445=DIRECTION ( 'NONE',  ( 0.000000000000000000, -1.000000000000000000, 0.000000000000000000 ) ) ;
#23448=CARTESIAN_POINT ( 'NONE',  ( 13.98007502452994189, -99.57060688034719931, -10.30433862638093423 ) ) ;
#23449=ORIENTED_EDGE ( 'NONE', *, *, #12006, .F. ) ;
#23456=CARTESIAN_POINT ( 'NONE',  ( 28.21663026719999934, -92.49537389030000156, 8.246881169159999914 ) ) ;
#23457=CARTESIAN_POINT ( 'NONE',  ( -5.897337460870000214, -101.1411470150000014, 14.21533967550000099 ) ) ;
#23458=ORIENTED_EDGE ( 'NONE', *, *, #7780, .T. ) ;
#23459=CARTESIAN_POINT ( 'NONE',  ( 14.01704999690000086, -99.70407914540000149, -9.961568965490000593 ) ) ;
#23460=CARTESIAN_POINT ( 'NONE',  ( -29.47186832370000076, -93.00000450890000536, -0.4149655844399999793 ) ) ;
#23461=AXIS2_PLACEMENT_3D ( 'NONE', #26071, #17620, #4059 ) ;
#23464=CARTESIAN_POINT ( 'NONE',  ( -13.26381099438660982, -101.5019029710790477, -9.144658545510399250 ) ) ;
#23465=CARTESIAN_POINT ( 'NONE',  ( 7.405704750090000843, -101.1273033739999931, 13.62605079230000094 ) ) ;
#23469=CARTESIAN_POINT ( 'NONE',  ( -18.71084207290000023, -96.58372172930000943, -10.18677576210000169 ) ) ;
#23470=CARTESIAN_POINT ( 'NONE',  ( 15.85792770375962490, -101.5620304352200094, 2.570904433130984046 ) ) ;
#23472=VERTEX_POINT ( 'NONE', #24933 ) ;
#23478=DIRECTION ( 'NONE',  ( 0.8981584475625411512, 0.000000000000000000, 0.4396719266362661416 ) ) ;
#23480=DIRECTION ( 'NONE',  ( 0.000000000000000000, 1.000000000000000000, 0.000000000000000000 ) ) ;
#23484=AXIS2_PLACEMENT_3D ( 'NONE', #11085, #15770, #17830 ) ;
#23491=CARTESIAN_POINT ( 'NONE',  ( -12.92073601179999898, -101.4254868729999970, -9.384144184709999337 ) ) ;
#23492=CARTESIAN_POINT ( 'NONE',  ( -18.05095945240000077, -93.00000167610001256, -23.30076308599999635 ) ) ;
#23494=AXIS2_PLACEMENT_3D ( 'NONE', #22696, #11895, #25178 ) ;
#23498=CARTESIAN_POINT ( 'NONE',  ( 7.258489506040000094, -101.1848542409999823, 13.44827353360000188 ) ) ;
#23499=ORIENTED_EDGE ( 'NONE', *, *, #20883, .T. ) ;
#23501=CARTESIAN_POINT ( 'NONE',  ( 13.53766003414172303, -100.5798851008411958, -10.01191531143067515 ) ) ;
#23504=CARTESIAN_POINT ( 'NONE',  ( 11.77817161740000174, -101.0685845459999967, -10.96540424870000052 ) ) ;
#23508=CARTESIAN_POINT ( 'NONE',  ( 11.91396536729999944, -101.5026188610000020, -10.71358336220000140 ) ) ;
#23510=CARTESIAN_POINT ( 'NONE',  ( -17.84952165019999981, -94.52419090329999563, 16.07137172610000064 ) ) ;
#23511=CARTESIAN_POINT ( 'NONE',  ( -17.09135004194092744, -92.81370807125685474, 25.26135588419946743 ) ) ;
#23512=EDGE_LOOP ( 'NONE', ( #13470, #23519, #1328, #8560 ) ) ;
#23514=DIRECTION ( 'NONE',  ( 0.8270692982020247941, 0.000000000000000000, 0.5620999697310169463 ) ) ;
#23515=CARTESIAN_POINT ( 'NONE',  ( -0.06019592984270000224, -101.1411470200000053, -15.38951065810000074 ) ) ;
#23516=CARTESIAN_POINT ( 'NONE',  ( 26.73328043595045500, -92.86910576385056970, -12.41347163419055732 ) ) ;
#23517=CARTESIAN_POINT ( 'NONE',  ( 15.32699008580000033, -101.0555477039999914, 2.288286655999999919 ) ) ;
#23519=ORIENTED_EDGE ( 'NONE', *, *, #2317, .T. ) ;
#23520=CARTESIAN_POINT ( 'NONE',  ( 6.467641717930000311, -99.94549701829998867, 15.61536050989999858 ) ) ;
#23522=CIRCLE ( 'NONE', #22587, 16.00000000000000000 ) ;
#23523=CARTESIAN_POINT ( 'NONE',  ( -11.31666932600000131, -95.23931402160000914, -21.36057898460000004 ) ) ;
#23526=CARTESIAN_POINT ( 'NONE',  ( -7.895913362729999996, -99.83167544280000527, 15.41983155350000168 ) ) ;
#23527=CARTESIAN_POINT ( 'NONE',  ( 8.558808717420001599, -94.34469964509999329, -23.93930828130000066 ) ) ;
#23535=CARTESIAN_POINT ( 'NONE',  ( 0.3657531947015631446, -101.3586211803499850, -16.22016006312202663 ) ) ;
#23538=CARTESIAN_POINT ( 'NONE',  ( 13.33972531995206623, -92.72059904818746645, 27.42811962378058510 ) ) ;
#23545=AXIS2_PLACEMENT_3D ( 'NONE', #8612, #6588, #24217 ) ;
#23547=ORIENTED_EDGE ( 'NONE', *, *, #11336, .F. ) ;
#23549=VERTEX_POINT ( 'NONE', #25918 ) ;
#23553=CARTESIAN_POINT ( 'NONE',  ( 9.273496630181142564, -94.57749869816520061, -22.35125168207579804 ) ) ;
#23555=EDGE_LOOP ( 'NONE', ( #8317, #23284, #11198, #11778 ) ) ;
#23558=EDGE_LOOP ( 'NONE', ( #5860, #28357, #11584, #9068 ) ) ;
#23563=CARTESIAN_POINT ( 'NONE',  ( -14.69223322520000075, -101.0355888259999944, 4.860466037580000176 ) ) ;
#23564=CARTESIAN_POINT ( 'NONE',  ( -15.58109701669999936, -101.5369810459999940, 3.638540083340000120 ) ) ;
#23567=ORIENTED_EDGE ( 'NONE', *, *, #16219, .F. ) ;
#23568=CARTESIAN_POINT ( 'NONE',  ( 20.42441471257877694, -98.07255008151754794, -1.452410518408777884 ) ) ;
#23573=CARTESIAN_POINT ( 'NONE',  ( 0.000000000000000000, -92.50000000000000000, 0.000000000000000000 ) ) ;
#23577=CARTESIAN_POINT ( 'NONE',  ( 6.880390998654439372, -100.3041487039077992, 15.60897913166483519 ) ) ;
#23578=CARTESIAN_POINT ( 'NONE',  ( 8.852567479250000204, -98.72068567929999006, 16.20451607640000091 ) ) ;
#23581=B_SPLINE_CURVE_WITH_KNOTS ( 'NONE', 5,
 ( #229, #24091, #6171, #15045, #23958, #21766 ),
 .UNSPECIFIED., .F., .F.,
 ( 6, 6 ),
 ( 0.000000000000000000, 1.000000000000000000 ),
 .UNSPECIFIED. ) ;
#23582=CARTESIAN_POINT ( 'NONE',  ( -18.62868452085797344, -97.90567604392204260, 5.830860830108250070 ) ) ;
#23583=ORIENTED_EDGE ( 'NONE', *, *, #16712, .T. ) ;
#23584=CARTESIAN_POINT ( 'NONE',  ( 29.41463188180000188, -92.63555401869999173, 7.090046362370000743 ) ) ;
#23586=CARTESIAN_POINT ( 'NONE',  ( -5.811429032009999496, -101.0314399550000104, 14.75160927930000021 ) ) ;
#23589=CARTESIAN_POINT ( 'NONE',  ( -0.8008942093612425595, -98.99956643305974069, -18.58022514274053094 ) ) ;
#23592=CARTESIAN_POINT ( 'NONE',  ( 16.79922297439999923, -99.53431386179998697, 4.586272525910000120 ) ) ;
#23596=CARTESIAN_POINT ( 'NONE',  ( 16.76165095789999882, -99.73367660430000115, 4.320137484619999135 ) ) ;
#23598=CARTESIAN_POINT ( 'NONE',  ( 24.02750282179999886, -93.67384740789999853, -8.937547196530001514 ) ) ;
#23600=CARTESIAN_POINT ( 'NONE',  ( 0.000000000000000000, -107.5000000000000000, 0.000000000000000000 ) ) ;
#23602=ORIENTED_EDGE ( 'NONE', *, *, #3564, .T. ) ;
#23603=CARTESIAN_POINT ( 'NONE',  ( -15.43525743989999910, -101.1461852590000063, 4.782895807790000120 ) ) ;
#23605=CARTESIAN_POINT ( 'NONE',  ( 16.83483077069999823, -99.92967571559999840, 4.239603657359999112 ) ) ;
#23612=ADVANCED_FACE ( 'NONE', ( #12633 ), #17811, .F. ) ;
#23621=CARTESIAN_POINT ( 'NONE',  ( 10.69681779260000098, -97.83805864369999483, 16.80092975179999826 ) ) ;
#23624=CARTESIAN_POINT ( 'NONE',  ( -15.08595480590000015, -92.80303298520000510, -23.69775107969999794 ) ) ;
#23625=CARTESIAN_POINT ( 'NONE',  ( -8.119791933969999320, -99.97545561319999763, 14.82168165659999914 ) ) ;
#23626=ORIENTED_EDGE ( 'NONE', *, *, #16219, .T. ) ;
#23627=CARTESIAN_POINT ( 'NONE',  ( 0.05992568041179999888, -93.49005502529999490, 26.18698436240000049 ) ) ;
#23629=CARTESIAN_POINT ( 'NONE',  ( 11.76103934369071702, -98.56104011604492143, -15.97798918033824656 ) ) ;
#23630=ORIENTED_EDGE ( 'NONE', *, *, #21202, .T. ) ;
#23632=CARTESIAN_POINT ( 'NONE',  ( 13.64952044873572312, -100.3796496172744668, -10.12948479266517232 ) ) ;
#23633=CARTESIAN_POINT ( 'NONE',  ( -22.25450259269999975, -94.89197151650000706, -8.089821617090001027 ) ) ;
#23634=CARTESIAN_POINT ( 'NONE',  ( 10.27467259300000002, -95.70830610299999819, -20.00247075010000231 ) ) ;
#23636=DIRECTION ( 'NONE',  ( 1.000000000000000000, 0.000000000000000000, 0.000000000000000000 ) ) ;
#23638=CARTESIAN_POINT ( 'NONE',  ( -18.19849796460000135, -94.71480814230000078, 16.19177224499999923 ) ) ;
#23639=CARTESIAN_POINT ( 'NONE',  ( -16.77460173512971053, -92.92035260009522801, 25.47427353929137439 ) ) ;
#23642=TOROIDAL_SURFACE ( 'NONE', #4074, 15.50000000000000000, 0.5000000000000000000 ) ;
#23643=CARTESIAN_POINT ( 'NONE',  ( -0.08783699053769999932, -101.6484611540000031, -16.00001271889999899 ) ) ;
#23645=CARTESIAN_POINT ( 'NONE',  ( 15.58784579500000156, -100.8733988930000010, 2.070706579690000382 ) ) ;
#23648=ORIENTED_EDGE ( 'NONE', *, *, #3385, .F. ) ;
#23649=CARTESIAN_POINT ( 'NONE',  ( 6.321364180049999781, -100.1512121650000040, 15.39199192900000135 ) ) ;
#23650=CARTESIAN_POINT ( 'NONE',  ( 15.66067906339999816, -101.4829589650000088, 3.855162640470000124 ) ) ;
#23651=EDGE_CURVE ( 'NONE', #11243, #24004, #8419, .T. ) ;
#23656=CIRCLE ( 'NONE', #17137, 5.000000000000000888 ) ;
#23658=CARTESIAN_POINT ( 'NONE',  ( 8.985924787889999266, -94.36515553530000489, -23.15004553760000050 ) ) ;
#23660=CARTESIAN_POINT ( 'NONE',  ( -15.92623219940000112, -93.13202907839999511, -20.96831028749999959 ) ) ;
#23667=CARTESIAN_POINT ( 'NONE',  ( 11.64589452461991037, -93.86980009079697140, -22.69836348088650979 ) ) ;
#23669=DIRECTION ( 'NONE',  ( 0.8775825618903722036, 0.000000000000000000, -0.4794255386042041156 ) ) ;
#23670=DIRECTION ( 'NONE',  ( 1.000000000000000000, 0.000000000000000000, 0.000000000000000000 ) ) ;
#23674=CARTESIAN_POINT ( 'NONE',  ( 11.63343413870000020, -100.9405348700000076, -10.90407401050000047 ) ) ;
#23677=DIRECTION ( 'NONE',  ( 1.000000000000000000, 0.000000000000000000, 0.000000000000000000 ) ) ;
#23678=ORIENTED_EDGE ( 'NONE', *, *, #28239, .T. ) ;
#23686=CARTESIAN_POINT ( 'NONE',  ( -29.29520252239999678, -92.62399497440000573, 4.740789425840000071 ) ) ;
#23687=CARTESIAN_POINT ( 'NONE',  ( 9.370945656724327222, -94.71481465630654384, -22.48432281284479117 ) ) ;
#23688=AXIS2_PLACEMENT_3D ( 'NONE', #7214, #27176, #244 ) ;
#23690=AXIS2_PLACEMENT_3D ( 'NONE', #18028, #20065, #28793 ) ;
#23691=AXIS2_PLACEMENT_3D ( 'NONE', #2802, #24648, #11656 ) ;
#23696=ORIENTED_EDGE ( 'NONE', *, *, #8477, .T. ) ;
#23700=CARTESIAN_POINT ( 'NONE',  ( -13.15133833870000046, -100.9197081840000010, -8.436152112259998503 ) ) ;
#23705=CARTESIAN_POINT ( 'NONE',  ( -12.43113460380000035, -101.2902355740000075, -9.959137603120000293 ) ) ;
#23707=CARTESIAN_POINT ( 'NONE',  ( -7.459817445499475674, -101.2637735886632129, 14.49077341668773578 ) ) ;
#23708=ORIENTED_EDGE ( 'NONE', *, *, #19178, .T. ) ;
#23718=CARTESIAN_POINT ( 'NONE',  ( 6.947152782944919558, -100.1994045928328774, 15.67154092987886216 ) ) ;
#23721=DIRECTION ( 'NONE',  ( 0.000000000000000000, 1.000000000000000000, 0.000000000000000000 ) ) ;
#23728=CARTESIAN_POINT ( 'NONE',  ( 13.88148934900000064, -99.91102932019998661, -9.687780287520000755 ) ) ;
#23730=AXIS2_PLACEMENT_3D ( 'NONE', #24709, #22377, #4450 ) ;
#23736=CARTESIAN_POINT ( 'NONE',  ( 12.38736960600000003, -101.0403179300000005, -9.267121510750001789 ) ) ;
#23739=CARTESIAN_POINT ( 'NONE',  ( 24.53124433849999875, -92.68289710869998999, -13.70463660470000100 ) ) ;
#23742=CARTESIAN_POINT ( 'NONE',  ( 29.71005176673471482, -92.93978723898561611, 6.896596330736053382 ) ) ;
#23747=CARTESIAN_POINT ( 'NONE',  ( 29.11677867130000052, -93.00000000000000000, 6.880015861159999524 ) ) ;
#23758=ORIENTED_EDGE ( 'NONE', *, *, #9646, .F. ) ;
#23762=CARTESIAN_POINT ( 'NONE',  ( 13.61159746509999913, -96.44392658620000702, 17.13483077990000325 ) ) ;
#23764=CARTESIAN_POINT ( 'NONE',  ( -7.887657129469999973, -99.88067631459999518, 15.44459931949999998 ) ) ;
#23765=CARTESIAN_POINT ( 'NONE',  ( -3.215500290640000536, -94.59276479679999738, 23.57860595660000058 ) ) ;
#23767=CIRCLE ( 'NONE', #22386, 5.500000000000000000 ) ;
#23769=AXIS2_PLACEMENT_3D ( 'NONE', #8131, #22251, #11148 ) ;
#23777=EDGE_CURVE ( 'NONE', #3830, #10282, #25301, .T. ) ;
#23779=CARTESIAN_POINT ( 'NONE',  ( -17.45201720579999716, -93.65993419859999847, 18.14866333539999843 ) ) ;
#23792=ADVANCED_FACE ( 'NONE', ( #24894 ), #12190, .F. ) ;
#23793=CARTESIAN_POINT ( 'NONE',  ( 6.355965434729999863, -99.91102932029998840, 15.68918534660000041 ) ) ;
#23794=CARTESIAN_POINT ( 'NONE',  ( 15.61571272419999978, -101.4908759489999994, 3.625172433619999968 ) ) ;
#23795=CARTESIAN_POINT ( 'NONE',  ( 7.286238495500000134, -101.2500498790000023, 13.33737010350000141 ) ) ;
#23801=CARTESIAN_POINT ( 'NONE',  ( -7.371671982299999648, -98.73889367950000917, 17.11857524030000022 ) ) ;
#23802=ORIENTED_EDGE ( 'NONE', *, *, #8790, .T. ) ;
#23803=CARTESIAN_POINT ( 'NONE',  ( 8.558247864140000161, -94.18458606759999441, -22.78405818970000141 ) ) ;
#23804=CARTESIAN_POINT ( 'NONE',  ( 0.000000000000000000, -91.50000000000000000, 0.000000000000000000 ) ) ;
#23805=CARTESIAN_POINT ( 'NONE',  ( -6.871575534529999807, -101.3138676899999950, 14.35405997169999814 ) ) ;
#23807=CARTESIAN_POINT ( 'NONE',  ( -29.86363316589999783, -101.1889999979999999, 0.3450520983969999622 ) ) ;
#23809=CARTESIAN_POINT ( 'NONE',  ( -1.604079331969999966, -100.9197086960000007, -15.54198441969999855 ) ) ;
#23813=CIRCLE ( 'NONE', #14497, 16.00000000000000000 ) ;
#23814=CARTESIAN_POINT ( 'NONE',  ( 16.19996591404212793, -94.70212264478905695, 17.23798455394816287 ) ) ;
#23816=DIRECTION ( 'NONE',  ( 0.000000000000000000, 1.000000000000000000, 0.000000000000000000 ) ) ;
#23821=ADVANCED_FACE ( 'NONE', ( #2752 ), #7267, .F. ) ;
#23823=ORIENTED_EDGE ( 'NONE', *, *, #26072, .T. ) ;
#23825=EDGE_LOOP ( 'NONE', ( #8065, #28096, #3373, #25969 ) ) ;
#23831=CARTESIAN_POINT ( 'NONE',  ( 15.63315392260000003, -100.5027207520000019, 4.441352150160000178 ) ) ;
#23834=VERTEX_POINT ( 'NONE', #15174 ) ;
#23837=CARTESIAN_POINT ( 'NONE',  ( -7.550578184249999047, -94.89197151660000884, -22.44319203070000057 ) ) ;
#23839=CARTESIAN_POINT ( 'NONE',  ( -14.99618466630000135, -101.1411470330000100, 3.458522314510000140 ) ) ;
#23842=VERTEX_POINT ( 'NONE', #27933 ) ;
#23845=CARTESIAN_POINT ( 'NONE',  ( 16.94740002120616396, -100.7167551730822908, 1.805771684632079488 ) ) ;
#23846=CARTESIAN_POINT ( 'NONE',  ( -12.51867210719999868, -101.6311724339999927, -9.986052846930000726 ) ) ;
#23848=CARTESIAN_POINT ( 'NONE',  ( 26.37318901919999803, -93.00000450890000536, 13.16123549989999830 ) ) ;
#23849=CARTESIAN_POINT ( 'NONE',  ( -7.902774248908001731, -100.3796496173660131, 15.04865541543737351 ) ) ;
#23852=CARTESIAN_POINT ( 'NONE',  ( -0.7205257401540000606, -101.6484611540000031, -15.98376809950000066 ) ) ;
#23859=CARTESIAN_POINT ( 'NONE',  ( 7.003224168222498491, -100.1240332945425564, 15.71316356361139910 ) ) ;
#23865=VERTEX_POINT ( 'NONE', #19847 ) ;
#23867=CARTESIAN_POINT ( 'NONE',  ( 28.45101619980000152, -92.62399496609999971, 8.439409298800001125 ) ) ;
#23870=ORIENTED_EDGE ( 'NONE', *, *, #25528, .F. ) ;
#23877=CARTESIAN_POINT ( 'NONE',  ( -22.01409729879999944, -92.76004107139999633, -20.03404935359999683 ) ) ;
#23882=CARTESIAN_POINT ( 'NONE',  ( 12.73439086970000034, -101.3878691800000098, -9.855841448820001460 ) ) ;
#23884=CARTESIAN_POINT ( 'NONE',  ( 24.71445532999999983, -93.30149055180000062, -11.27282922470000237 ) ) ;
#23886=AXIS2_PLACEMENT_3D ( 'NONE', #3714, #28318, #7948 ) ;
#23888=DIRECTION ( 'NONE',  ( 0.000000000000000000, 1.000000000000000000, 0.000000000000000000 ) ) ;
#23892=CARTESIAN_POINT ( 'NONE',  ( 23.58466923419999972, -94.98812477769999418, -2.405350023570000051 ) ) ;
#23895=VECTOR ( 'NONE', #2726, 1000.000000000000114 ) ;
#23896=VERTEX_POINT ( 'NONE', #28007 ) ;
#23899=CARTESIAN_POINT ( 'NONE',  ( -11.85289063449999958, -94.98812477599999227, -21.44324726029999795 ) ) ;
#23900=ORIENTED_EDGE ( 'NONE', *, *, #1043, .T. ) ;
#23904=ORIENTED_EDGE ( 'NONE', *, *, #2488, .F. ) ;
#23905=CARTESIAN_POINT ( 'NONE',  ( 10.64217894839999978, -97.74063293919999751, 16.82202129059999862 ) ) ;
#23906=CARTESIAN_POINT ( 'NONE',  ( -16.08644287450000121, -92.54349754189999544, -23.90073121629999875 ) ) ;
#23907=CARTESIAN_POINT ( 'NONE',  ( -8.247318090510001198, -99.72202992580000114, 15.06295020069999957 ) ) ;
#23908=CARTESIAN_POINT ( 'NONE',  ( -1.709235988930000172, -93.75379239749999272, 24.88396779469999842 ) ) ;
#23910=TOROIDAL_SURFACE ( 'NONE', #9505, 5.500000000000000000, 0.5000000000000000000 ) ;
#23912=CARTESIAN_POINT ( 'NONE',  ( -18.88944331909999974, -111.0000000000000000, -23.13319212550000259 ) ) ;
#23914=CARTESIAN_POINT ( 'NONE',  ( 12.77542149835405638, -101.4728631013604456, -9.856360518087987188 ) ) ;
#23917=CARTESIAN_POINT ( 'NONE',  ( 9.108768065319999607, -94.52419709919999491, -22.22443129089999658 ) ) ;
#23920=APPLICATION_CONTEXT ( 'automotive_design' ) ;
#23923=CARTESIAN_POINT ( 'NONE',  ( -20.53694319417668268, -92.95475433444754287, 17.43128291165811916 ) ) ;
#23926=AXIS2_PLACEMENT_3D ( 'NONE', #2062, #13252, #26526 ) ;
#23927=DIRECTION ( 'NONE',  ( 1.000000000000000000, 0.000000000000000000, 0.000000000000000000 ) ) ;
#23933=CARTESIAN_POINT ( 'NONE',  ( 6.038481244350000665, -100.8023006570000035, 14.57509264930000015 ) ) ;
#23934=CARTESIAN_POINT ( 'NONE',  ( 15.61329055410000066, -101.5216621940000152, 3.544188506249999815 ) ) ;
#23935=AXIS2_PLACEMENT_3D ( 'NONE', #4876, #13165, #2403 ) ;
#23941=CARTESIAN_POINT ( 'NONE',  ( 4.528887711649999481, -92.66001714109999909, -27.65183955359999857 ) ) ;
#23945=CARTESIAN_POINT ( 'NONE',  ( -6.668573295719999905, -101.1716782170000073, 14.25075804799999979 ) ) ;
#23949=CARTESIAN_POINT ( 'NONE',  ( -5.873418876839999747, -101.3150700380000018, 15.15334698740000086 ) ) ;
#23951=EDGE_CURVE ( 'NONE', #23472, #23865, #170, .T. ) ;
#23952=CARTESIAN_POINT ( 'NONE',  ( 27.07580689300000287, -92.50000460620000808, -12.39707951610000158 ) ) ;
#23953=ADVANCED_FACE ( 'NONE', ( #7908 ), #811, .T. ) ;
#23954=ORIENTED_EDGE ( 'NONE', *, *, #6592, .T. ) ;
#23955=CARTESIAN_POINT ( 'NONE',  ( -0.7191277762650000183, -101.4254868729999970, -15.95275638909999749 ) ) ;
#23958=CARTESIAN_POINT ( 'NONE',  ( 12.83908560070000071, -94.89197151660000884, -19.89638108760000179 ) ) ;
#23959=CARTESIAN_POINT ( 'NONE',  ( 15.99636488046209060, -94.79936261290481525, 17.25621003525883168 ) ) ;
#23962=CARTESIAN_POINT ( 'NONE',  ( 13.81100091409999919, -99.92967571559999840, -10.51865105429999936 ) ) ;
#23971=CARTESIAN_POINT ( 'NONE',  ( -25.74949179000000044, -93.99830544879999650, -2.429629024850000096 ) ) ;
#23974=VECTOR ( 'NONE', #13521, 1000.000000000000000 ) ;
#23975=VERTEX_POINT ( 'NONE', #14461 ) ;
#23976=CARTESIAN_POINT ( 'NONE',  ( -18.06114732863891348, -97.34036579259480959, -10.09119009767709407 ) ) ;
#23980=DIRECTION ( 'NONE',  ( 1.000000000000000000, 0.000000000000000000, 0.000000000000000000 ) ) ;
#23987=CARTESIAN_POINT ( 'NONE',  ( 11.14159932559999966, -101.1364147039999892, -10.55279472049999967 ) ) ;
#23990=CARTESIAN_POINT ( 'NONE',  ( -11.82347332360000003, -101.2358105800000061, -9.579693020240000578 ) ) ;
#23992=CARTESIAN_POINT ( 'NONE',  ( -7.312065474886813909, -101.4085864806282160, 14.43964435962598358 ) ) ;
#23994=B_SPLINE_CURVE_WITH_KNOTS ( 'NONE', 5,
 ( #2185, #13381, #24324, #13088, #26814, #6550 ),
 .UNSPECIFIED., .F., .F.,
 ( 6, 6 ),
 ( 0.000000000000000000, 1.000000000000000000 ),
 .UNSPECIFIED. ) ;
#23997=ORIENTED_EDGE ( 'NONE', *, *, #17203, .F. ) ;
#23999=FACE_OUTER_BOUND ( 'NONE', #4449, .T. ) ;
#24001=FACE_OUTER_BOUND ( 'NONE', #7802, .T. ) ;
#24004=VERTEX_POINT ( 'NONE', #27452 ) ;
#24006=CARTESIAN_POINT ( 'NONE',  ( -15.36947826900000003, -101.0685828069999985, 4.769131590209999771 ) ) ;
#24007=CARTESIAN_POINT ( 'NONE',  ( 10.52519477159999894, -92.53453854219999641, 27.02797911619999738 ) ) ;
#24015=CARTESIAN_POINT ( 'NONE',  ( -16.50842902520000166, -93.39359504729999628, -21.60523500349999892 ) ) ;
#24019=CARTESIAN_POINT ( 'NONE',  ( 13.66933441149999950, -100.1459902240000019, -10.03108682719999933 ) ) ;
#24022=B_SPLINE_CURVE_WITH_KNOTS ( 'NONE', 5,
 ( #22665, #9390, #13766, #9676, #25145, #20179, #2709, #26892, #9539, #20319, #543, #389 ),
 .UNSPECIFIED., .F., .F.,
 ( 6, 3, 3, 6 ),
 ( -25.08217526889999860, -18.82033206645258616, -10.56888224947905819, -7.186327137053730496 ),
 .UNSPECIFIED. ) ;
#24027=DIRECTION ( 'NONE',  ( 0.000000000000000000, 1.000000000000000000, 0.000000000000000000 ) ) ;
#24029=CARTESIAN_POINT ( 'NONE',  ( -0.6731250195771717459, -92.54938211485213628, -30.49269871153447298 ) ) ;
#24031=CARTESIAN_POINT ( 'NONE',  ( -11.69653606700000026, -94.52419709919999491, -20.97822790150000216 ) ) ;
#24034=CARTESIAN_POINT ( 'NONE',  ( 20.76627821419999975, -96.95622423369999865, -2.346863933399999880 ) ) ;
#24035=ORIENTED_EDGE ( 'NONE', *, *, #16821, .T. ) ;
#24040=CARTESIAN_POINT ( 'NONE',  ( -12.96744186819999989, -101.1042759770000004, -9.004950000140000910 ) ) ;
#24043=CARTESIAN_POINT ( 'NONE',  ( -8.190587505059999884, -99.74726900420000675, 15.07401393059999961 ) ) ;
#24049=CARTESIAN_POINT ( 'NONE',  ( 13.65853266997999071, -100.3617719036068081, -10.14140713304427877 ) ) ;
#24056=CARTESIAN_POINT ( 'NONE',  ( -15.93508487770000137, -92.93255488879999859, 23.98294276400000058 ) ) ;
#24057=CARTESIAN_POINT ( 'NONE',  ( -20.55830956777789709, -92.99223971643057496, 17.22324199352144092 ) ) ;
#24062=CARTESIAN_POINT ( 'NONE',  ( 0.6375376905170000441, -100.5229262450000078, -16.86993779310000008 ) ) ;
#24064=CARTESIAN_POINT ( 'NONE',  ( 15.53498458480000011, -101.1499348409999897, 2.599897626340000212 ) ) ;
#24067=ORIENTED_EDGE ( 'NONE', *, *, #6681, .F. ) ;
#24068=CARTESIAN_POINT ( 'NONE',  ( 6.656205481639999810, -101.1976625110000043, 14.93341658319999965 ) ) ;
#24069=CARTESIAN_POINT ( 'NONE',  ( 15.00803725019999924, -101.1284992150000051, 3.477295974860000083 ) ) ;
#24071=ORIENTED_EDGE ( 'NONE', *, *, #8694, .F. ) ;
#24076=ORIENTED_EDGE ( 'NONE', *, *, #196, .F. ) ;
#24077=CARTESIAN_POINT ( 'NONE',  ( 4.580264318640000276, -92.68289710869998999, -27.72400028910000458 ) ) ;
#24079=CARTESIAN_POINT ( 'NONE',  ( 6.738397544221694346, -101.4241070619504796, 14.70285685720373792 ) ) ;
#24081=ORIENTED_EDGE ( 'NONE', *, *, #17203, .T. ) ;
#24084=DIRECTION ( 'NONE',  ( 1.000000000000000000, 0.000000000000000000, 0.000000000000000000 ) ) ;
#24087=CARTESIAN_POINT ( 'NONE',  ( 26.91890708249999875, -92.56168957700000988, -12.40459431399999879 ) ) ;
#24088=CARTESIAN_POINT ( 'NONE',  ( -1.229530056899999835, -101.0685849509999912, -16.04536266459999894 ) ) ;
#24091=CARTESIAN_POINT ( 'NONE',  ( 13.03263341399999931, -94.63960343439998724, -19.83860458410000049 ) ) ;
#24093=ORIENTED_EDGE ( 'NONE', *, *, #1428, .T. ) ;
#24094=CARTESIAN_POINT ( 'NONE',  ( -14.83395525729999775, -101.1411475039999885, 4.096596759159999657 ) ) ;
#24098=ADVANCED_FACE ( 'NONE', ( #17498 ), #13584, .T. ) ;
#24103=CARTESIAN_POINT ( 'NONE',  ( 24.19803400451018760, -94.16483583547625358, -8.868831527973414453 ) ) ;
#24107=VECTOR ( 'NONE', #20633, 1000.000000000000000 ) ;
#24114=CARTESIAN_POINT ( 'NONE',  ( -25.20910175530000075, -93.61368346379998684, -2.138151043640000193 ) ) ;
#24116=FACE_OUTER_BOUND ( 'NONE', #22896, .T. ) ;
#24117=ORIENTED_EDGE ( 'NONE', *, *, #21910, .T. ) ;
#24127=DIRECTION ( 'NONE',  ( 0.000000000000000000, 1.000000000000000000, 0.000000000000000000 ) ) ;
#24129=CARTESIAN_POINT ( 'NONE',  ( -13.41619584950000110, -101.2306315440000049, -9.103915625870000028 ) ) ;
#24132=CARTESIAN_POINT ( 'NONE',  ( -12.12074076350000063, -101.1180794200000008, -9.692271323269999073 ) ) ;
#24135=CARTESIAN_POINT ( 'NONE',  ( -7.422674037662165603, -101.3038909012893924, 14.47466155340364757 ) ) ;
#24137=ADVANCED_FACE ( 'NONE', ( #22161 ), #6865, .F. ) ;
#24148=AXIS2_PLACEMENT_3D ( 'NONE', #1396, #16830, #25719 ) ;
#24150=CARTESIAN_POINT ( 'NONE',  ( -18.26810397560000254, -94.98812477769999418, 16.32728546869999775 ) ) ;
#24151=ORIENTED_EDGE ( 'NONE', *, *, #26367, .T. ) ;
#24152=CARTESIAN_POINT ( 'NONE',  ( -20.25756709850169557, -95.19002702548807804, 10.95028088663572774 ) ) ;
#24154=CARTESIAN_POINT ( 'NONE',  ( 22.14531096509999841, -93.99830645880000191, 13.36130718660000127 ) ) ;
#24161=CARTESIAN_POINT ( 'NONE',  ( -20.49992799259999998, -92.87863185410000710, -20.70054720279999927 ) ) ;
#24167=CARTESIAN_POINT ( 'NONE',  ( 13.52017591309999922, -100.2511768809999921, -9.777168233029998490 ) ) ;
#24169=CARTESIAN_POINT ( 'NONE',  ( -11.69298166125931004, -94.57749869814954025, -21.18608910009514901 ) ) ;
#24170=DIRECTION ( 'NONE',  ( 0.000000000000000000, 1.000000000000000000, 0.000000000000000000 ) ) ;
#24171=CARTESIAN_POINT ( 'NONE',  ( 29.95046995577899196, -92.50630337894793342, 5.765085911501825144 ) ) ;
#24174=EDGE_CURVE ( 'NONE', #3921, #19835, #12249, .T. ) ;
#24175=DIRECTION ( 'NONE',  ( 0.9601004944592521628, 0.000000000000000000, -0.2796552172570708761 ) ) ;
#24179=CARTESIAN_POINT ( 'NONE',  ( -0.1055951870944554088, -92.72722989461847476, -30.49981915221950146 ) ) ;
#24180=EDGE_CURVE ( 'NONE', #4878, #11981, #24642, .T. ) ;
#24187=CARTESIAN_POINT ( 'NONE',  ( 22.49719386810000188, -95.90105812930001150, -4.302050608990000136 ) ) ;
#24188=EDGE_LOOP ( 'NONE', ( #6789, #8096, #1540, #5051 ) ) ;
#24191=EDGE_LOOP ( 'NONE', ( #23179, #10463, #5967, #14412, #25760, #7158, #1807 ) ) ;
#24192=CARTESIAN_POINT ( 'NONE',  ( 16.49889766720000139, -94.79581468469999095, 16.97757898100000062 ) ) ;
#24193=B_SPLINE_CURVE_WITH_KNOTS ( 'NONE', 5,
 ( #1205, #27421, #10039, #5685, #784, #7881, #20570, #7312, #18954, #926, #18824, #27837 ),
 .UNSPECIFIED., .F., .F.,
 ( 6, 3, 3, 6 ),
 ( 0.000000000000000000, 0.4964111757593314134, 0.7833083924331026848, 1.000000000000000000 ),
 .UNSPECIFIED. ) ;
#24194=CARTESIAN_POINT ( 'NONE',  ( -16.09760936190000180, -92.53016485179999506, -24.04852265159999902 ) ) ;
#24195=DIRECTION ( 'NONE',  ( 0.000000000000000000, 1.000000000000000000, 0.000000000000000000 ) ) ;
#24197=CARTESIAN_POINT ( 'NONE',  ( -6.571450035919999877, -97.39505561490000218, -20.10197936720000200 ) ) ;
#24198=CARTESIAN_POINT ( 'NONE',  ( -29.03051485019999944, -92.50425969839999141, 5.507518881380000231 ) ) ;
#24200=CARTESIAN_POINT ( 'NONE',  ( -29.53621923517769332, -92.52640451558471568, 7.606711608869601626 ) ) ;
#24201=CARTESIAN_POINT ( 'NONE',  ( 11.97834023485886235, -100.7167551706393738, -12.12413065688971692 ) ) ;
#24209=CARTESIAN_POINT ( 'NONE',  ( -13.35883408399999972, -92.54627707209999699, 27.01063094439999901 ) ) ;
#24210=CARTESIAN_POINT ( 'NONE',  ( 27.07127034026193968, -92.49999918154685474, -10.05443361004321723 ) ) ;
#24216=CARTESIAN_POINT ( 'NONE',  ( 0.5403162009290000123, -100.8772072149999985, -15.79149104430000250 ) ) ;
#24217=DIRECTION ( 'NONE',  ( 1.000000000000000000, 0.000000000000000000, 0.000000000000000000 ) ) ;
#24218=CARTESIAN_POINT ( 'NONE',  ( 15.48147096319999960, -101.1716782170000073, 2.806783133030000155 ) ) ;
#24221=ORIENTED_EDGE ( 'NONE', *, *, #27357, .T. ) ;
#24224=CARTESIAN_POINT ( 'NONE',  ( -17.53169073309999959, -94.47975186520000079, 16.30735973009999995 ) ) ;
#24226=DIRECTION ( 'NONE',  ( 1.000000000000000000, 0.000000000000000000, 0.000000000000000000 ) ) ;
#24229=CARTESIAN_POINT ( 'NONE',  ( -17.00715350810000004, -99.92967601899998442, 3.484608414699999823 ) ) ;
#24234=CARTESIAN_POINT ( 'NONE',  ( -6.572142520109999886, -101.1292389600000092, 14.04468523589999940 ) ) ;
#24236=CARTESIAN_POINT ( 'NONE',  ( -13.11204875850966012, -100.1406256088236830, -11.11584611941340839 ) ) ;
#24239=CARTESIAN_POINT ( 'NONE',  ( 25.53753465840000203, -93.24058218609999926, -5.819240763660000759 ) ) ;
#24240=CARTESIAN_POINT ( 'NONE',  ( -1.044714352840000027, -101.1042759770000004, -15.75284879089999812 ) ) ;
#24241=CARTESIAN_POINT ( 'NONE',  ( -23.77081188420000046, -93.00000000000000000, -19.11016751280000037 ) ) ;
#24243=CARTESIAN_POINT ( 'NONE',  ( -21.10288026827540264, -92.92035259892315935, -22.02258658995163287 ) ) ;
#24245=CARTESIAN_POINT ( 'NONE',  ( -15.30640947800000085, -101.3256025499999993, 4.329700326000000210 ) ) ;
#24253=CARTESIAN_POINT ( 'NONE',  ( 27.00388527187511656, -93.12686943497722325, 10.05985568221045767 ) ) ;
#24255=VERTEX_POINT ( 'NONE', #9902 ) ;
#24261=CARTESIAN_POINT ( 'NONE',  ( -24.12299397890000208, -94.89419905519999077, -4.133205798090000549 ) ) ;
#24265=CARTESIAN_POINT ( 'NONE',  ( -17.97303742817231509, -97.38870237790561646, -10.12129934261613151 ) ) ;
#24267=EDGE_LOOP ( 'NONE', ( #10408, #28643, #28403, #5065 ) ) ;
#24271=CARTESIAN_POINT ( 'NONE',  ( 0.7331063123750001242, -99.53431386179998697, -17.39857302659999760 ) ) ;
#24281=CARTESIAN_POINT ( 'NONE',  ( -12.32330071950000061, -101.1617736559999940, -9.795274802109998902 ) ) ;
#24288=ORIENTED_EDGE ( 'NONE', *, *, #6843, .T. ) ;
#24290=CYLINDRICAL_SURFACE ( 'NONE', #18602, 18.64285714289999163 ) ;
#24291=CARTESIAN_POINT ( 'NONE',  ( -18.19849796459701707, -94.71480814228209510, 16.19177224503937751 ) ) ;
#24293=EDGE_CURVE ( 'NONE', #26855, #18774, #5254, .T. ) ;
#24294=CARTESIAN_POINT ( 'NONE',  ( -20.39102396179032084, -94.78512952904711142, 11.78310433714105976 ) ) ;
#24303=VECTOR ( 'NONE', #4307, 1000.000000000000000 ) ;
#24304=CIRCLE ( 'NONE', #2001, 16.00000000000000000 ) ;
#24307=CARTESIAN_POINT ( 'NONE',  ( -23.28637498790000038, -92.50000947299999154, -18.90060859649999969 ) ) ;
#24309=DIRECTION ( 'NONE',  ( 0.000000000000000000, -1.000000000000000000, 0.000000000000000000 ) ) ;
#24311=EDGE_CURVE ( 'NONE', #21723, #7597, #16393, .T. ) ;
#24313=CARTESIAN_POINT ( 'NONE',  ( 12.81378706179999938, -101.0640712160000021, -9.747090585469999624 ) ) ;
#24318=CARTESIAN_POINT ( 'NONE',  ( 12.39757656149999931, -101.6484611540000031, -10.11435096289999969 ) ) ;
#24322=CARTESIAN_POINT ( 'NONE',  ( 7.615531154710000195, -93.65023553240000354, -24.05380218500000211 ) ) ;
#24324=CARTESIAN_POINT ( 'NONE',  ( 21.33284145582814517, -96.53847999911016586, 1.142362698555328793 ) ) ;
#24325=CARTESIAN_POINT ( 'NONE',  ( -25.37284092810000047, -93.00000000000000000, 2.543411731580000001 ) ) ;
#24328=AXIS2_PLACEMENT_3D ( 'NONE', #26, #26674, #4824 ) ;
#24332=CARTESIAN_POINT ( 'NONE',  ( 15.77847595849999784, -100.9405345029999950, 2.296807716130000010 ) ) ;
#24333=ORIENTED_EDGE ( 'NONE', *, *, #18924, .T. ) ;
#24336=VERTEX_POINT ( 'NONE', #5406 ) ;
#24341=CARTESIAN_POINT ( 'NONE',  ( -4.663136541669999247, -98.35430138709999426, -18.48787719950000152 ) ) ;
#24344=DIRECTION ( 'NONE',  ( 0.000000000000000000, 1.000000000000000000, 0.000000000000000000 ) ) ;
#24346=CARTESIAN_POINT ( 'NONE',  ( 11.60004717582089739, -98.07566646012705291, -16.86827489351441045 ) ) ;
#24347=ORIENTED_EDGE ( 'NONE', *, *, #23007, .F. ) ;
#24350=CARTESIAN_POINT ( 'NONE',  ( -13.34153245340000105, -111.0000000000000000, 27.42724032409999779 ) ) ;
#24356=CARTESIAN_POINT ( 'NONE',  ( -17.75840719219999997, -93.65013249519999761, 19.45109209530000172 ) ) ;
#24360=CARTESIAN_POINT ( 'NONE',  ( 0.2077369398249999943, -101.1402801299999936, -15.33898559480000046 ) ) ;
#24362=CARTESIAN_POINT ( 'NONE',  ( 15.74335372269999844, -101.6484611540000031, 2.854262349889999939 ) ) ;
#24365=CARTESIAN_POINT ( 'NONE',  ( -18.34989813179999985, -101.1889999979999999, 23.56346505449999995 ) ) ;
#24367=ORIENTED_EDGE ( 'NONE', *, *, #25496, .F. ) ;
#24369=DIRECTION ( 'NONE',  ( 1.000000000000000000, 0.000000000000000000, 0.000000000000000000 ) ) ;
#24372=CARTESIAN_POINT ( 'NONE',  ( 22.61295488650000252, -92.68419354099999907, 15.80596811629999721 ) ) ;
#24377=CARTESIAN_POINT ( 'NONE',  ( -12.57246511061115157, -100.9510322836001137, -10.75256427542645099 ) ) ;
#24382=CARTESIAN_POINT ( 'NONE',  ( 9.220169834260000030, -98.40144667389999711, 16.53004056780000042 ) ) ;
#24385=CARTESIAN_POINT ( 'NONE',  ( -5.660850080320000366, -95.85308664740000495, -21.77572594749999979 ) ) ;
#24387=CARTESIAN_POINT ( 'NONE',  ( -20.12052720778319426, -92.59033770634258076, -22.92234717996245408 ) ) ;
#24389=CARTESIAN_POINT ( 'NONE',  ( 11.80818982729999966, -101.2459394079999981, -10.72877140129999951 ) ) ;
#24394=B_SPLINE_CURVE_WITH_KNOTS ( 'NONE', 5,
 ( #28076, #19332, #8242, #28492, #23837, #21240 ),
 .UNSPECIFIED., .F., .F.,
 ( 6, 6 ),
 ( 0.000000000000000000, 1.000000000000000000 ),
 .UNSPECIFIED. ) ;
#24398=CARTESIAN_POINT ( 'NONE',  ( 24.68647381493572723, -93.48480241409957614, -11.77680583462976216 ) ) ;
#24399=CARTESIAN_POINT ( 'NONE',  ( 22.55799654273938160, -93.99439547208534407, 13.13363697907470851 ) ) ;
#24402=AXIS2_PLACEMENT_3D ( 'NONE', #15644, #13463, #22369 ) ;
#24404=EDGE_LOOP ( 'NONE', ( #11278, #15342, #17021, #18885, #27999, #17959, #16756 ) ) ;
#24408=DIRECTION ( 'NONE',  ( 1.000000000000000000, 0.000000000000000000, 0.000000000000000000 ) ) ;
#24410=CARTESIAN_POINT ( 'NONE',  ( -14.99091303862281777, -98.53908159007769996, -11.25711904965173460 ) ) ;
#24414=CARTESIAN_POINT ( 'NONE',  ( -13.16239939709999796, -100.8816831189999874, -8.729909459909999114 ) ) ;
#24417=CARTESIAN_POINT ( 'NONE',  ( 8.036636119666090039, -92.56492639278413037, 29.42229982729625704 ) ) ;
#24422=CARTESIAN_POINT ( 'NONE',  ( 24.54513662149999931, -93.07154530310000951, -11.24897352390000016 ) ) ;
#24423=CARTESIAN_POINT ( 'NONE',  ( 8.852567479250000204, -98.72068567929999006, 16.20451607640000091 ) ) ;
#24425=CARTESIAN_POINT ( 'NONE',  ( 13.88364982429999905, -99.64579499010000063, -10.35699147140000065 ) ) ;
#24426=VERTEX_POINT ( 'NONE', #17031 ) ;
#24430=CARTESIAN_POINT ( 'NONE',  ( -12.90060417029999940, -99.77922884479998800, -11.29212820419999908 ) ) ;
#24432=DIRECTION ( 'NONE',  ( 1.000000000000000000, 0.000000000000000000, 0.000000000000000000 ) ) ;
#24433=EDGE_LOOP ( 'NONE', ( #7734, #13424, #3778, #20947 ) ) ;
#24435=CARTESIAN_POINT ( 'NONE',  ( 0.000000000000000000, -108.5000000000000000, 6.000000000000000000 ) ) ;
#24436=VERTEX_POINT ( 'NONE', #12914 ) ;
#24437=DIRECTION ( 'NONE',  ( 0.000000000000000000, -1.000000000000000000, 0.000000000000000000 ) ) ;
#24439=CARTESIAN_POINT ( 'NONE',  ( 12.04737265749960784, -101.5555610555548469, -10.52904611307853777 ) ) ;
#24440=ORIENTED_EDGE ( 'NONE', *, *, #5792, .F. ) ;
#24444=CARTESIAN_POINT ( 'NONE',  ( -19.13290590728680129, -97.24060876560415068, 7.010995730810996029 ) ) ;
#24446=CARTESIAN_POINT ( 'NONE',  ( -24.46593625966632501, -94.79128788238732284, -3.807804778192843020 ) ) ;
#24447=CARTESIAN_POINT ( 'NONE',  ( 22.17077749659999952, -94.09272483339999837, 13.34913124499999881 ) ) ;
#24455=VERTEX_POINT ( 'NONE', #12634 ) ;
#24456=CARTESIAN_POINT ( 'NONE',  ( -1.381305061119999955, -100.8816835080000089, -15.73378738089999729 ) ) ;
#24457=CARTESIAN_POINT ( 'NONE',  ( -17.12548609519999943, -99.53431381699999747, 3.156820590889999778 ) ) ;
#24461=DIRECTION ( 'NONE',  ( 0.000000000000000000, -1.000000000000000000, 0.000000000000000000 ) ) ;
#24466=EDGE_CURVE ( 'NONE', #17507, #11243, #8028, .T. ) ;
#24479=CARTESIAN_POINT ( 'NONE',  ( 17.94519931069999785, -99.91547912500000450, 1.181841864839999756 ) ) ;
#24492=CARTESIAN_POINT ( 'NONE',  ( 12.21423488090000120, -93.96464232169999775, -21.69898374830000165 ) ) ;
#24498=CARTESIAN_POINT ( 'NONE',  ( -15.81949116929999910, -92.71181266049998726, 23.89725124530000144 ) ) ;
#24500=VERTEX_POINT ( 'NONE', #18042 ) ;
#24502=CARTESIAN_POINT ( 'NONE',  ( 0.4062216120019999654, -101.0147083550000104, -15.54305921829999981 ) ) ;
#24507=ADVANCED_FACE ( 'NONE', ( #15693 ), #12702, .F. ) ;
#24509=EDGE_CURVE ( 'NONE', #20007, #21750, #22986, .T. ) ;
#24511=CARTESIAN_POINT ( 'NONE',  ( 28.44836026452301070, -92.82668962668340384, 10.99730886889462056 ) ) ;
#24512=CARTESIAN_POINT ( 'NONE',  ( 7.894724219650000485, -99.51557806589998734, 16.06685178089999866 ) ) ;
#24514=CARTESIAN_POINT ( 'NONE',  ( 17.44131645659999919, -95.98460699740000734, 14.95162584959999919 ) ) ;
#24519=CARTESIAN_POINT ( 'NONE',  ( -7.009104771800000577, -101.4908759489999994, 14.41751744779999989 ) ) ;
#24520=ORIENTED_EDGE ( 'NONE', *, *, #24509, .F. ) ;
#24524=ORIENTED_EDGE ( 'NONE', *, *, #15198, .T. ) ;
#24525=CARTESIAN_POINT ( 'NONE',  ( 9.279094190520000396, -98.48918237500001283, 16.48187022329999962 ) ) ;
#24527=CARTESIAN_POINT ( 'NONE',  ( -0.8449272815640000989, -98.83667233820000320, -18.63222145299999966 ) ) ;
#24528=CARTESIAN_POINT ( 'NONE',  ( -19.92928515724098659, -92.55017404142323301, -23.08838732444159092 ) ) ;
#24529=CARTESIAN_POINT ( 'NONE',  ( -15.50938067939999954, -101.3150705480000084, 4.855933298290000089 ) ) ;
#24531=CARTESIAN_POINT ( 'NONE',  ( 12.90275855517485049, -96.31541554714243603, 17.28766916121755770 ) ) ;
#24537=CARTESIAN_POINT ( 'NONE',  ( 24.70175895849127912, -93.12686943433988063, -14.84027023513776200 ) ) ;
#24538=CARTESIAN_POINT ( 'NONE',  ( 24.27624741938561570, -93.55106866556637613, 12.16912909751702720 ) ) ;
#24539=ORIENTED_EDGE ( 'NONE', *, *, #1831, .T. ) ;
#24542=CARTESIAN_POINT ( 'NONE',  ( 8.071148094770000725, -100.8816835939999947, 13.57632622700000091 ) ) ;
#24543=CONICAL_SURFACE ( 'NONE', #22216, 5.999999999999999112, 0.7853981633970000820 ) ;
#24544=ADVANCED_FACE ( 'NONE', ( #8993 ), #8039, .T. ) ;
#24549=CARTESIAN_POINT ( 'NONE',  ( 7.102042752109999135, -111.0000000000000000, 14.33739825589999839 ) ) ;
#24550=CARTESIAN_POINT ( 'NONE',  ( -24.07227057460000097, -94.80026553589999594, -4.144178597490000726 ) ) ;
#24559=CARTESIAN_POINT ( 'NONE',  ( 7.312846564840000063, -92.50000000000000000, 29.61034067890000188 ) ) ;
#24561=DIRECTION ( 'NONE',  ( 0.000000000000000000, 1.000000000000000000, 0.000000000000000000 ) ) ;
#24564=CARTESIAN_POINT ( 'NONE',  ( 24.44279401320000034, -92.66001714109999909, -13.69981297090000005 ) ) ;
#24568=CARTESIAN_POINT ( 'NONE',  ( -17.43464046073879814, -96.56053630746443162, 12.16311153714526050 ) ) ;
#24572=CARTESIAN_POINT ( 'NONE',  ( 27.25648091989999955, -93.00000000000000000, -13.26500883389999963 ) ) ;
#24573=CARTESIAN_POINT ( 'NONE',  ( -11.94559458280000008, -100.4792519539999915, -10.93369168340000108 ) ) ;
#24574=DIRECTION ( 'NONE',  ( 0.4794255386042041156, 0.000000000000000000, 0.8775825618903722036 ) ) ;
#24576=EDGE_LOOP ( 'NONE', ( #23626, #12157, #21305, #8394, #24093, #8266, #4339 ) ) ;
#24579=CARTESIAN_POINT ( 'NONE',  ( 26.34682155151427096, -92.82044061126494228, -15.36538583964133053 ) ) ;
#24580=PRODUCT_DEFINITION_FORMATION_WITH_SPECIFIED_SOURCE ( 'ANY', '', #26194, .NOT_KNOWN. ) ;
#24583=B_SPLINE_SURFACE_WITH_KNOTS ( 'NONE', 5, 5, ( 
 ( #24457, #443, #11171, #4933, #303, #9440, #26944, #6986, #149 ),
 ( #27090, #9001, #596, #11617, #20527, #24903, #7131, #15850, #24759 ),
 ( #13672, #22577, #14670, #23290, #18639, #16442, #5649, #19057, #14115 ),
 ( #1167, #3470, #14259, #27535, #14527, #7978, #7423, #27800, #16724 ),
 ( #2909, #18920, #16868, #5511, #27942, #3333, #12197, #12335, #25757 ),
 ( #25201, #5230, #21112, #7716, #25477, #11919, #23014, #9872, #11771 ),
 ( #5785, #14398, #20971, #10006, #20822, #12055, #18786, #7842, #25620 ),
 ( #3064, #9726, #23152, #23434, #21243, #884, #7578, #25346, #3197 ),
 ( #1034, #1294, #10137, #20683, #5376, #16290, #744, #27678, #9589 ),
 ( #16583, #18489, #27380, #12462, #19187, #8667, #14935, #17139, #17575 ),
 ( #8244, #17435, #23839, #3882, #12747, #10279, #26029, #23564, #21375 ),
 ( #6055, #21659, #6500, #19748, #1707, #28636, #8113, #3602, #6208 ) ),
 .UNSPECIFIED., .F., .F., .F.,
 ( 6, 3, 3, 6 ),
 ( 6, 3, 6 ),
 ( 3.365447998909999683, 5.319894352600000431, 6.690827956829999756, 7.896981424030000696 ),
 ( 0.000000000000000000, 0.2500000000000000000, 0.5000000000000000000 ),
 .UNSPECIFIED. ) ;
#24586=CARTESIAN_POINT ( 'NONE',  ( 12.79650330539999992, -92.63554657719998886, 27.41785451570000021 ) ) ;
#24595=ORIENTED_EDGE ( 'NONE', *, *, #25740, .T. ) ;
#24596=DIRECTION ( 'NONE',  ( 0.000000000000000000, 1.000000000000000000, 0.000000000000000000 ) ) ;
#24600=CARTESIAN_POINT ( 'NONE',  ( -13.34720188679999886, -94.24983875549999368, -21.61594323940000351 ) ) ;
#24608=CARTESIAN_POINT ( 'NONE',  ( -12.35307240344411994, -101.1962283502562059, -8.971858293833401277 ) ) ;
#24610=CARTESIAN_POINT ( 'NONE',  ( 28.66244647610000129, -91.50000000000000000, 10.42660836539999991 ) ) ;
#24615=ADVANCED_FACE ( 'NONE', ( #20374 ), #24583, .T. ) ;
#24616=CARTESIAN_POINT ( 'NONE',  ( -10.69999465949999973, -93.40479992090000394, -23.45152081580000214 ) ) ;
#24617=ADVANCED_FACE ( 'NONE', ( #10694 ), #10373, .F. ) ;
#24619=DIRECTION ( 'NONE',  ( 1.000000000000000000, 0.000000000000000000, 0.000000000000000000 ) ) ;
#24620=CARTESIAN_POINT ( 'NONE',  ( -24.48306397703444048, -92.50630337894787658, -18.18918482052484720 ) ) ;
#24632=ORIENTED_EDGE ( 'NONE', *, *, #3531, .F. ) ;
#24639=EDGE_CURVE ( 'NONE', #20422, #1013, #17728, .T. ) ;
#24640=CARTESIAN_POINT ( 'NONE',  ( 8.040406065020551551, -94.10917102489311503, -24.59531423993398036 ) ) ;
#24642=LINE ( 'NONE', #22305, #3426 ) ;
#24645=ORIENTED_EDGE ( 'NONE', *, *, #21392, .F. ) ;
#24648=DIRECTION ( 'NONE',  ( 0.000000000000000000, 1.000000000000000000, 0.000000000000000000 ) ) ;
#24651=ADVANCED_FACE ( 'NONE', ( #24866 ), #28775, .F. ) ;
#24653=CARTESIAN_POINT ( 'NONE',  ( -17.77445941079999869, -93.74388477669999986, 19.47957637960000099 ) ) ;
#24655=CARTESIAN_POINT ( 'NONE',  ( -16.03899174369999869, -99.57125562240000249, 6.799714415290000424 ) ) ;
#24656=CARTESIAN_POINT ( 'NONE',  ( 0.5505338958400000093, -101.0875971110000080, -15.39929819530000010 ) ) ;
#24657=CARTESIAN_POINT ( 'NONE',  ( -3.215510237749999778, -94.59276292389999696, 23.57860181210000405 ) ) ;
#24662=CARTESIAN_POINT ( 'NONE',  ( 7.100891874899999401, -99.78393592979999482, 15.80033508019999822 ) ) ;
#24665=CARTESIAN_POINT ( 'NONE',  ( -13.52989530590000022, -92.50182112220001329, 26.44972089899999901 ) ) ;
#24666=CARTESIAN_POINT ( 'NONE',  ( 12.61928293329999917, -98.69239344479998977, 15.21635193949999909 ) ) ;
#24667=ORIENTED_EDGE ( 'NONE', *, *, #24174, .F. ) ;
#24669=CARTESIAN_POINT ( 'NONE',  ( 22.54964778510000301, -92.87437365150000801, 15.59122118179999994 ) ) ;
#24671=ORIENTED_EDGE ( 'NONE', *, *, #14848, .F. ) ;
#24681=CARTESIAN_POINT ( 'NONE',  ( -0.6842253571740000151, -101.2530993000000024, -15.17849927279999989 ) ) ;
#24682=CARTESIAN_POINT ( 'NONE',  ( -29.63524900250000016, -92.56168957700000988, -0.5035227619879999450 ) ) ;
#24683=CARTESIAN_POINT ( 'NONE',  ( -3.898844501749999747, -96.83679385029999764, -20.89542445309999863 ) ) ;
#24686=CARTESIAN_POINT ( 'NONE',  ( 11.86655925200000183, -101.3150705500000157, -11.10431217030000006 ) ) ;
#24687=CARTESIAN_POINT ( 'NONE',  ( 14.95895049385062059, -95.29940929529944071, 17.31812158372859045 ) ) ;
#24694=ORIENTED_EDGE ( 'NONE', *, *, #2561, .T. ) ;
#24695=CARTESIAN_POINT ( 'NONE',  ( -29.76177017585215268, -92.96960399592616398, 6.669860268962034766 ) ) ;
#24696=CARTESIAN_POINT ( 'NONE',  ( 8.188640737180000073, -100.9197086730000024, 13.30685945699999984 ) ) ;
#24707=CARTESIAN_POINT ( 'NONE',  ( 16.60616815699999904, -99.99711545080000974, 4.374379691520000613 ) ) ;
#24709=CARTESIAN_POINT ( 'NONE',  ( 16.48132342839999964, -101.1889999979999999, 2.988055897779999803 ) ) ;
#24711=CARTESIAN_POINT ( 'NONE',  ( -22.13586109129999713, -95.90105813160000992, -5.885152931789999542 ) ) ;
#24713=CARTESIAN_POINT ( 'NONE',  ( 8.955369301398645732, -92.77481473455837602, 29.15572894638344792 ) ) ;
#24727=CARTESIAN_POINT ( 'NONE',  ( -16.10740345911051108, -99.26499635306740288, 7.485719296024102576 ) ) ;
#24731=CARTESIAN_POINT ( 'NONE',  ( -13.06366830770000043, -99.99711545080000974, -11.14632625079999961 ) ) ;
#24736=ORIENTED_EDGE ( 'NONE', *, *, #28680, .T. ) ;
#24738=DIRECTION ( 'NONE',  ( 0.6285074900730004410, 0.000000000000000000, -0.7778035323410003032 ) ) ;
#24739=CARTESIAN_POINT ( 'NONE',  ( -0.8151677527090001041, -95.98460638129999722, 22.95835728570000001 ) ) ;
#24740=AXIS2_PLACEMENT_3D ( 'NONE', #17546, #4133, #13301 ) ;
#24741=CARTESIAN_POINT ( 'NONE',  ( 5.626505627759999406, -93.46569726110000431, 26.69085374259999810 ) ) ;
#24743=ORIENTED_EDGE ( 'NONE', *, *, #13150, .F. ) ;
#24747=CARTESIAN_POINT ( 'NONE',  ( 21.02256860540000005, -93.91547409650000588, 13.07290323880000038 ) ) ;
#24750=DIRECTION ( 'NONE',  ( 0.000000000000000000, 1.000000000000000000, 0.000000000000000000 ) ) ;
#24753=CARTESIAN_POINT ( 'NONE',  ( 11.84128442000000092, -101.1848541609999899, -9.660509526330001151 ) ) ;
#24754=CARTESIAN_POINT ( 'NONE',  ( -13.18688177930000016, -93.32822605769999313, -23.58441486170000090 ) ) ;
#24758=DIRECTION ( 'NONE',  ( 0.000000000000000000, 1.000000000000000000, 0.000000000000000000 ) ) ;
#24759=CARTESIAN_POINT ( 'NONE',  ( -16.91430575710000284, -100.0771588430000065, 3.341621066080000091 ) ) ;
#24771=CARTESIAN_POINT ( 'NONE',  ( 15.69647852281674538, -101.4241070620424381, 3.898789967113180932 ) ) ;
#24777=CARTESIAN_POINT ( 'NONE',  ( 1.375225265779999928, -94.98812079580000045, 24.46248543800000164 ) ) ;
#24778=ORIENTED_EDGE ( 'NONE', *, *, #5821, .F. ) ;
#24786=CARTESIAN_POINT ( 'NONE',  ( 15.50925563669999896, -100.9197081840000010, 1.894558565230000102 ) ) ;
#24791=CARTESIAN_POINT ( 'NONE',  ( 0.000000000000000000, -108.5000000000000000, 0.000000000000000000 ) ) ;
#24808=CARTESIAN_POINT ( 'NONE',  ( -0.6842253573819999657, -101.2530993000000024, -15.17849927279999989 ) ) ;
#24812=FACE_BOUND ( 'NONE', #747, .T. ) ;
#24814=CARTESIAN_POINT ( 'NONE',  ( -15.06840628259999981, -92.56711348129999806, 24.34572243330000063 ) ) ;
#24816=CARTESIAN_POINT ( 'NONE',  ( 14.80687252510000107, -97.01506571140001256, 14.57555587629999927 ) ) ;
#24819=CARTESIAN_POINT ( 'NONE',  ( 24.55398044940000446, -92.70565333729999224, 14.54119304790000022 ) ) ;
#24822=CIRCLE ( 'NONE', #23427, 23.79684788999999867 ) ;
#24826=CARTESIAN_POINT ( 'NONE',  ( 7.073120017670000870, -99.73367811500000357, 15.79835279589999963 ) ) ;
#24828=CARTESIAN_POINT ( 'NONE',  ( -5.542684685070000228, -95.66919271819999437, -21.81728948419999981 ) ) ;
#24829=CARTESIAN_POINT ( 'NONE',  ( 13.81100091409999919, -99.92967571559999840, -10.51865105429999936 ) ) ;
#24830=CARTESIAN_POINT ( 'NONE',  ( 11.77817022719999862, -101.0685849509999912, -10.96540529560000010 ) ) ;
#24831=DIRECTION ( 'NONE',  ( 0.000000000000000000, -1.000000000000000000, 0.000000000000000000 ) ) ;
#24838=CARTESIAN_POINT ( 'NONE',  ( -14.77445022520000073, -101.2530993010000060, 3.545507728379999612 ) ) ;
#24839=EDGE_LOOP ( 'NONE', ( #7153, #13581, #8547, #9059 ) ) ;
#24842=CARTESIAN_POINT ( 'NONE',  ( 7.844113379649998663, -101.1184174639999895, 13.21637662110000022 ) ) ;
#24852=CIRCLE ( 'NONE', #26726, 4.999999999999999112 ) ;
#24854=ORIENTED_EDGE ( 'NONE', *, *, #6683, .F. ) ;
#24857=CARTESIAN_POINT ( 'NONE',  ( -23.50863772330000145, -94.59276583650000703, -3.692488328609999648 ) ) ;
#24859=CARTESIAN_POINT ( 'NONE',  ( -30.47693414353797792, -92.55017404142812154, 1.185968520876313326 ) ) ;
#24861=DIRECTION ( 'NONE',  ( 0.000000000000000000, 1.000000000000000000, 0.000000000000000000 ) ) ;
#24863=CARTESIAN_POINT ( 'NONE',  ( 15.74335372269999844, -101.1889999979999999, 2.854262350110000401 ) ) ;
#24866=FACE_OUTER_BOUND ( 'NONE', #10577, .T. ) ;
#24868=CARTESIAN_POINT ( 'NONE',  ( -17.53389815281536812, -96.07279461669297405, 13.09664283538910468 ) ) ;
#24869=ORIENTED_EDGE ( 'NONE', *, *, #130, .F. ) ;
#24871=DIRECTION ( 'NONE',  ( -0.006434372441722441445, 0.000000000000000000, 0.9999792992113792911 ) ) ;
#24873=FACE_OUTER_BOUND ( 'NONE', #19352, .T. ) ;
#24877=CARTESIAN_POINT ( 'NONE',  ( 26.33787588810572444, -92.82529299094895237, -15.38071215267214420 ) ) ;
#24878=ORIENTED_EDGE ( 'NONE', *, *, #25773, .T. ) ;
#24882=CARTESIAN_POINT ( 'NONE',  ( 12.61209325099999923, -101.1889999979999999, -11.02259514940000074 ) ) ;
#24884=CARTESIAN_POINT ( 'NONE',  ( 5.611330023069999839, -93.37393516990000819, 26.68650669730000047 ) ) ;
#24894=FACE_OUTER_BOUND ( 'NONE', #2736, .T. ) ;
#24895=CARTESIAN_POINT ( 'NONE',  ( 7.236990221556244940, -101.1962284174823594, 13.44316210220003249 ) ) ;
#24898=CARTESIAN_POINT ( 'NONE',  ( 12.37352278080000012, -101.4254868729999970, -10.09472709699999982 ) ) ;
#24899=CARTESIAN_POINT ( 'NONE',  ( -18.05096283909999855, -93.00000167610001256, -23.30076369320000040 ) ) ;
#24900=CARTESIAN_POINT ( 'NONE',  ( 5.273680924649999824, -107.3487944130000074, 9.653408180790000515 ) ) ;
#24903=CARTESIAN_POINT ( 'NONE',  ( -16.86763901309999980, -99.92604429489999518, 3.250425998059999877 ) ) ;
#24907=DIRECTION ( 'NONE',  ( 1.000000000000000000, 0.000000000000000000, 0.000000000000000000 ) ) ;
#24911=CARTESIAN_POINT ( 'NONE',  ( -13.12430011460000046, -92.94829811809999853, -23.71756069369999764 ) ) ;
#24915=CARTESIAN_POINT ( 'NONE',  ( 16.04726154520435699, -100.8738282915798123, 4.264385135213858646 ) ) ;
#24920=CARTESIAN_POINT ( 'NONE',  ( 6.114061450890000415, -101.1889999979999999, -13.40104985119999981 ) ) ;
#24926=VERTEX_POINT ( 'NONE', #2660 ) ;
#24933=CARTESIAN_POINT ( 'NONE',  ( 13.81100091409999919, -111.0000000000000000, -10.51865105429999936 ) ) ;
#24934=CARTESIAN_POINT ( 'NONE',  ( -28.75282704045790538, -92.49999918155121748, -2.687052330903884290 ) ) ;
#24936=CARTESIAN_POINT ( 'NONE',  ( -19.51771074589999699, -96.73994798520000415, 8.394649969090000496 ) ) ;
#24940=CARTESIAN_POINT ( 'NONE',  ( 12.83908560070000071, -94.89197151660000884, -19.89638108760000179 ) ) ;
#24942=CARTESIAN_POINT ( 'NONE',  ( -13.11938740068049825, -92.71619979444491833, 27.53419132531503166 ) ) ;
#24943=ORIENTED_EDGE ( 'NONE', *, *, #26296, .T. ) ;
#24944=CARTESIAN_POINT ( 'NONE',  ( -11.98370860700000051, -101.2530993010000060, -9.340542411159999503 ) ) ;
#24948=CARTESIAN_POINT ( 'NONE',  ( -17.58843202809999795, -98.51728656799998873, 8.830207771419999574 ) ) ;
#24949=CARTESIAN_POINT ( 'NONE',  ( 0.6893497139830000453, -99.55609327400000552, -17.37226014440000199 ) ) ;
#24960=CIRCLE ( 'NONE', #2637, 16.00000000000000000 ) ;
#24961=CARTESIAN_POINT ( 'NONE',  ( 23.54413596224770799, -92.59055325462402664, -19.38875311991260730 ) ) ;
#24964=CARTESIAN_POINT ( 'NONE',  ( 6.153538926910000484, -92.84292488370000740, 28.82528031139999669 ) ) ;
#24968=ORIENTED_EDGE ( 'NONE', *, *, #24180, .F. ) ;
#24969=CARTESIAN_POINT ( 'NONE',  ( 8.932460458690000493, -98.93374375299998746, 16.36585915649999734 ) ) ;
#24970=ADVANCED_FACE ( 'NONE', ( #17947 ), #7026, .T. ) ;
#24974=CARTESIAN_POINT ( 'NONE',  ( -15.43525461730000004, -101.1461875130000010, 4.782897338129999731 ) ) ;
#24976=CARTESIAN_POINT ( 'NONE',  ( 14.57207603078257030, -95.48799328830101274, 17.32764375622651798 ) ) ;
#24980=FACE_OUTER_BOUND ( 'NONE', #9129, .T. ) ;
#24981=CARTESIAN_POINT ( 'NONE',  ( 0.000000000000000000, -108.5000000000000000, 0.000000000000000000 ) ) ;
#24983=CARTESIAN_POINT ( 'NONE',  ( -29.76015270875833707, -92.93978723898862881, 6.677089761457638772 ) ) ;
#24985=CARTESIAN_POINT ( 'NONE',  ( 7.021283738330000190, -101.6484611540000031, 14.37740230390000029 ) ) ;
#24987=CARTESIAN_POINT ( 'NONE',  ( 23.58655624800000083, -94.70873613630000420, -2.249367945439999961 ) ) ;
#24989=CARTESIAN_POINT ( 'NONE',  ( -18.69985100839999959, -93.00000000000000000, 22.78328762010000119 ) ) ;
#24993=CARTESIAN_POINT ( 'NONE',  ( -19.98978262542267359, -95.81137667811660208, 9.708844812268232261 ) ) ;
#24994=CARTESIAN_POINT ( 'NONE',  ( 16.23185304080000080, -99.92384627689999377, 4.745118442920000845 ) ) ;
#24997=CARTESIAN_POINT ( 'NONE',  ( -17.68956059909999823, -98.30614355279999472, -8.105910472710000647 ) ) ;
#25005=CARTESIAN_POINT ( 'NONE',  ( 23.06813085299999955, -94.22763312370000222, -7.559806761219999949 ) ) ;
#25008=CARTESIAN_POINT ( 'NONE',  ( -16.27155717411393354, -99.02168173220448466, 7.873387082247683466 ) ) ;
#25009=B_SPLINE_SURFACE_WITH_KNOTS ( 'NONE', 5, 5, ( 
 ( #19636, #28526, #17171, #19922, #19362, #8562, #13416, #24307, #28235 ),
 ( #26060, #6088, #12779, #23877, #12915, #3914, #4195, #6378, #22129 ),
 ( #21828, #4348, #24161, #6238, #19494, #2028, #15103, #17464, #10868 ),
 ( #19778, #28381, #17757, #26350, #8411, #17317, #13363, #1885, #26212 ),
 ( #15394, #24015, #2170, #10722, #28659, #8691, #8844, #26641, #6685 ),
 ( #15549, #1605, #9839, #439, #22266, #16684, #13513, #2614, #26939 ),
 ( #9976, #24600, #13668, #11167, #20081, #18191, #22422, #18891, #27773 ),
 ( #23259, #5476, #298, #7810, #145, #16551, #8995, #11464, #2468 ),
 ( #20370, #9287, #18749, #3302, #9139, #25589, #13810, #27084, #17903 ) ),
 .UNSPECIFIED., .F., .F., .F.,
 ( 6, 3, 6 ),
 ( 6, 3, 6 ),
 ( 7.186332008850000008, 18.82032538960000068, 25.08217527079999698 ),
 ( 0.000000000000000000, 0.2500000000000000000, 0.5000000000000000000 ),
 .UNSPECIFIED. ) ;
#25010=ORIENTED_EDGE ( 'NONE', *, *, #20939, .T. ) ;
#25016=DIRECTION ( 'NONE',  ( 1.000000000000000000, 0.000000000000000000, 0.000000000000000000 ) ) ;
#25019=CARTESIAN_POINT ( 'NONE',  ( 26.35926584486895408, -92.81370807106951304, -15.34403634914452397 ) ) ;
#25021=AXIS2_PLACEMENT_3D ( 'NONE', #23747, #21564, #25665 ) ;
#25023=VECTOR ( 'NONE', #18831, 1000.000000000000000 ) ;
#25024=CARTESIAN_POINT ( 'NONE',  ( 1.316303147800000017, -94.80026829419999501, 24.39090705379999946 ) ) ;
#25025=CARTESIAN_POINT ( 'NONE',  ( 5.717411334609999507, -92.96448467939998750, 26.13902206350000057 ) ) ;
#25047=ORIENTED_EDGE ( 'NONE', *, *, #12350, .F. ) ;
#25049=CARTESIAN_POINT ( 'NONE',  ( 0.000000000000000000, -94.59276292389999696, 0.000000000000000000 ) ) ;
#25050=EDGE_CURVE ( 'NONE', #21458, #16504, #12286, .T. ) ;
#25051=CARTESIAN_POINT ( 'NONE',  ( -0.02543935853460000188, -101.2530993010000060, -15.19457030269999898 ) ) ;
#25053=B_SPLINE_CURVE_WITH_KNOTS ( 'NONE', 3,
 ( #13398, #2649, #22458, #22303, #13848, #4827, #24640, #2349, #11500, #11202, #18379, #20113, #2501, #181, #9029, #26678, #7013, #17936, #26830, #19957, #6863, #15727, #4669, #13549, #328, #15880, #22606, #20259, #11355, #13704, #20408, #9322, #18226, #27123, #13997, #7163, #16171 ),
 .UNSPECIFIED., .F., .F.,
 ( 4, 2, 2, 1, 1, 1, 2, 2, 2, 2, 1, 1, 1, 2, 2, 2, 2, 1, 1, 1, 2, 2, 4 ),
 ( 0.000000000000000000, 0.1249999999999811817, 0.1874999999999717726, 0.2187499999999666933, 0.2343749999999644451, 0.2421874999999634459, 0.2460937499999632794, 0.2499999999999630851, 0.3749999999999583111, 0.4374999999999563127, 0.4687499999999551470, 0.4843749999999545364, 0.4921874999999544809, 0.4960937499999547029, 0.4999999999999548139, 0.6249999999999622524, 0.6874999999999660272, 0.7187499999999676925, 0.7343749999999685807, 0.7421874999999692468, 0.7460937499999694689, 0.7499999999999698019, 1.000000000000000000 ),
 .UNSPECIFIED. ) ;
#25054=ORIENTED_EDGE ( 'NONE', *, *, #502, .F. ) ;
#25056=CARTESIAN_POINT ( 'NONE',  ( -11.86917066319999847, -93.06764199929999393, -23.73933353450000183 ) ) ;
#25059=CARTESIAN_POINT ( 'NONE',  ( 15.63748056140000209, -101.6484611540000031, 3.386620984279999913 ) ) ;
#25061=VERTEX_POINT ( 'NONE', #24944 ) ;
#25063=CARTESIAN_POINT ( 'NONE',  ( 16.42966103859999905, -94.59276292389999696, 17.21499949629999904 ) ) ;
#25069=CARTESIAN_POINT ( 'NONE',  ( 6.602264112093322090, -93.38552847742499807, 26.87384619217190007 ) ) ;
#25072=ORIENTED_EDGE ( 'NONE', *, *, #10462, .F. ) ;
#25082=CARTESIAN_POINT ( 'NONE',  ( 22.78264860270000014, -94.59276292389999696, -6.873201011689999085 ) ) ;
#25087=VECTOR ( 'NONE', #4611, 1000.000000000000000 ) ;
#25096=EDGE_CURVE ( 'NONE', #25651, #22535, #8716, .T. ) ;
#25112=CARTESIAN_POINT ( 'NONE',  ( 8.097645732220000170, -101.1461871030000168, 13.98396704560000003 ) ) ;
#25113=ORIENTED_EDGE ( 'NONE', *, *, #28215, .F. ) ;
#25115=CARTESIAN_POINT ( 'NONE',  ( 15.63748056140000209, -101.6484611540000031, 3.386620984279999913 ) ) ;
#25118=CARTESIAN_POINT ( 'NONE',  ( -10.83727467601077699, -93.79427251235401286, -23.30769844343626218 ) ) ;
#25120=CARTESIAN_POINT ( 'NONE',  ( 7.625237055219999505, -101.6466297510000061, 14.06768965610000066 ) ) ;
#25125=CARTESIAN_POINT ( 'NONE',  ( 11.40864485750000057, -99.60591459030000294, -13.10462926860000010 ) ) ;
#25126=ORIENTED_EDGE ( 'NONE', *, *, #20155, .T. ) ;
#25129=DIRECTION ( 'NONE',  ( 1.000000000000000000, 0.000000000000000000, 0.000000000000000000 ) ) ;
#25131=CARTESIAN_POINT ( 'NONE',  ( 14.73729790613776203, -95.40730986357353061, 17.32447803859898983 ) ) ;
#25132=EDGE_CURVE ( 'NONE', #16242, #17051, #12723, .T. ) ;
#25140=CARTESIAN_POINT ( 'NONE',  ( 6.878957409089999864, -101.2902355740000075, 14.36654009489999950 ) ) ;
#25141=DIRECTION ( 'NONE',  ( 0.7529607911047510038, 0.000000000000000000, -0.6580653820547830435 ) ) ;
#25145=CARTESIAN_POINT ( 'NONE',  ( 23.44684503250000063, -93.13202985540000611, 11.98166338640000106 ) ) ;
#25152=ORIENTED_EDGE ( 'NONE', *, *, #6891, .F. ) ;
#25153=CARTESIAN_POINT ( 'NONE',  ( 8.071148094770000725, -100.8816835939999947, 13.57632622700000091 ) ) ;
#25158=CARTESIAN_POINT ( 'NONE',  ( 0.5062329661385056578, -101.1248211537367894, -16.39898467942452953 ) ) ;
#25166=ORIENTED_EDGE ( 'NONE', *, *, #7322, .F. ) ;
#25177=EDGE_CURVE ( 'NONE', #11981, #22767, #1103, .T. ) ;
#25178=DIRECTION ( 'NONE',  ( 0.4862861358100820097, 0.000000000000000000, 0.8737996304181516738 ) ) ;
#25180=DIRECTION ( 'NONE',  ( 1.000000000000000000, 0.000000000000000000, 0.000000000000000000 ) ) ;
#25181=CARTESIAN_POINT ( 'NONE',  ( -0.5009807240759999170, -95.72998414420000302, 22.40906914880000045 ) ) ;
#25182=CARTESIAN_POINT ( 'NONE',  ( 11.26569178309999941, -92.63504499639999779, 27.45908696089999879 ) ) ;
#25183=ORIENTED_EDGE ( 'NONE', *, *, #6926, .F. ) ;
#25184=CARTESIAN_POINT ( 'NONE',  ( -11.21686577274311603, -94.79904837829768383, -20.68495353529920777 ) ) ;
#25186=CARTESIAN_POINT ( 'NONE',  ( -27.90659341333026688, -93.31462968106396261, 0.8904257685511188791 ) ) ;
#25190=AXIS2_PLACEMENT_3D ( 'NONE', #16618, #18529, #11812 ) ;
#25196=CARTESIAN_POINT ( 'NONE',  ( -11.20154639050000078, -94.96739875689999621, -21.25936308859999713 ) ) ;
#25200=FACE_OUTER_BOUND ( 'NONE', #16742, .T. ) ;
#25201=CARTESIAN_POINT ( 'NONE',  ( -15.71880468089999816, -100.6825640990000039, 2.591412482229999981 ) ) ;
#25204=ORIENTED_EDGE ( 'NONE', *, *, #13137, .F. ) ;
#25206=CARTESIAN_POINT ( 'NONE',  ( -7.915630935209213348, -100.0863963177362166, 15.30813341843738229 ) ) ;
#25208=CARTESIAN_POINT ( 'NONE',  ( -8.556134930689999862, -94.37361474979999798, -22.79835356780000311 ) ) ;
#25211=CARTESIAN_POINT ( 'NONE',  ( 16.65148481214054854, -100.1240332945786662, 4.321656103344765576 ) ) ;
#25212=CARTESIAN_POINT ( 'NONE',  ( 19.83536231727052268, -94.71481465627687157, 14.13922899595298333 ) ) ;
#25214=CIRCLE ( 'NONE', #10729, 0.4999999999999997780 ) ;
#25216=AXIS2_PLACEMENT_3D ( 'NONE', #6179, #1409, #14909 ) ;
#25222=CARTESIAN_POINT ( 'NONE',  ( 6.393980055115425998, -93.41742240778975770, 26.81347393697559411 ) ) ;
#25231=ADVANCED_FACE ( 'NONE', ( #7278 ), #23910, .F. ) ;
#25237=AXIS2_PLACEMENT_3D ( 'NONE', #18053, #26952, #22140 ) ;
#25239=ORIENTED_EDGE ( 'NONE', *, *, #20576, .T. ) ;
#25241=CARTESIAN_POINT ( 'NONE',  ( 16.83481230680000351, -99.92967428129999519, 4.239616764530000026 ) ) ;
#25242=CARTESIAN_POINT ( 'NONE',  ( -19.88566801240000004, -92.51556124920000457, 20.76300894400000274 ) ) ;
#25244=EDGE_LOOP ( 'NONE', ( #3571, #11572, #12121, #18193 ) ) ;
#25245=DIRECTION ( 'NONE',  ( 0.000000000000000000, -1.000000000000000000, 0.000000000000000000 ) ) ;
#25246=CARTESIAN_POINT ( 'NONE',  ( 7.292753731799999528, -92.50000000000000000, -29.01615345709999971 ) ) ;
#25249=CARTESIAN_POINT ( 'NONE',  ( -18.15843401709999938, -97.14937512070000025, 11.14356573500000103 ) ) ;
#25255=DIRECTION ( 'NONE',  ( 1.000000000000000000, 0.000000000000000000, 0.000000000000000000 ) ) ;
#25263=ORIENTED_EDGE ( 'NONE', *, *, #19654, .T. ) ;
#25265=CARTESIAN_POINT ( 'NONE',  ( 27.70978180510000044, -92.50000000000000000, 12.74433177200000067 ) ) ;
#25266=EDGE_CURVE ( 'NONE', #7118, #1115, #7319, .T. ) ;
#25269=CARTESIAN_POINT ( 'NONE',  ( -8.022941090739999837, -100.0496341300000154, 14.88870835790000058 ) ) ;
#25272=CARTESIAN_POINT ( 'NONE',  ( 7.394414626720000605, -101.1280782930000015, 13.63119500039999998 ) ) ;
#25277=CARTESIAN_POINT ( 'NONE',  ( 12.11202172750000017, -100.0012764439999984, -13.34364409169999988 ) ) ;
#25281=CARTESIAN_POINT ( 'NONE',  ( 11.58748549300000086, -101.1411470200000053, -10.12711838239999906 ) ) ;
#25284=CARTESIAN_POINT ( 'NONE',  ( -16.94283757680843294, -92.86276749033184785, 25.36152676960142927 ) ) ;
#25288=CYLINDRICAL_SURFACE ( 'NONE', #6722, 18.64285714290000229 ) ;
#25289=CYLINDRICAL_SURFACE ( 'NONE', #225, 30.50000000000002132 ) ;
#25290=EDGE_LOOP ( 'NONE', ( #28102, #3979, #17456, #15738 ) ) ;
#25291=CARTESIAN_POINT ( 'NONE',  ( 6.496108347790000792, -101.2358105800000061, 13.76101799030000095 ) ) ;
#25295=EDGE_CURVE ( 'NONE', #139, #20804, #9299, .T. ) ;
#25296=CARTESIAN_POINT ( 'NONE',  ( -11.38188984059999775, -94.78088171070000101, -20.62154665490000127 ) ) ;
#25300=CARTESIAN_POINT ( 'NONE',  ( 16.79922297439999923, -99.53431386179998697, 4.586272525910000120 ) ) ;
#25301=CIRCLE ( 'NONE', #14579, 5.500000000000001776 ) ;
#25303=ADVANCED_FACE ( 'NONE', ( #5083 ), #9008, .T. ) ;
#25304=DIRECTION ( 'NONE',  ( 0.000000000000000000, 1.000000000000000000, 0.000000000000000000 ) ) ;
#25307=CARTESIAN_POINT ( 'NONE',  ( -20.43643619460000238, -93.49011727610000833, 16.37406953600000037 ) ) ;
#25310=CARTESIAN_POINT ( 'NONE',  ( -0.007034495156453384086, -101.6297509123136393, -16.01459432531875748 ) ) ;
#25315=B_SPLINE_CURVE_WITH_KNOTS ( 'NONE', 5,
 ( #25451, #27202, #14079, #997, #15963, #22980 ),
 .UNSPECIFIED., .F., .F.,
 ( 6, 6 ),
 ( 0.000000000000000000, 1.000000000000000000 ),
 .UNSPECIFIED. ) ;
#25316=CARTESIAN_POINT ( 'NONE',  ( 23.92048446921776161, -92.96960399593338309, -18.92248458225377661 ) ) ;
#25322=ORIENTED_EDGE ( 'NONE', *, *, #9898, .F. ) ;
#25331=CARTESIAN_POINT ( 'NONE',  ( 4.060851860889999720, -93.80272730500000478, 26.06633832969999887 ) ) ;
#25332=ORIENTED_EDGE ( 'NONE', *, *, #4581, .T. ) ;
#25335=CARTESIAN_POINT ( 'NONE',  ( -0.6441375867304897085, -93.86980009075321618, 25.50348311024104575 ) ) ;
#25346=CARTESIAN_POINT ( 'NONE',  ( -15.80605669150000203, -101.3276421320000082, 3.296406198950000199 ) ) ;
#25349=EDGE_LOOP ( 'NONE', ( #26922, #20514, #20465, #14731, #14067 ) ) ;
#25358=CARTESIAN_POINT ( 'NONE',  ( 16.68572014148854166, -100.0863963178369431, 4.310789395909731425 ) ) ;
#25366=CARTESIAN_POINT ( 'NONE',  ( 8.971603365988027434, -93.12686175135999633, 27.38471516527505756 ) ) ;
#25374=ORIENTED_EDGE ( 'NONE', *, *, #14703, .F. ) ;
#25379=CARTESIAN_POINT ( 'NONE',  ( 7.635702898730000854, -101.6454117330000031, 14.06304778130000166 ) ) ;
#25380=VERTEX_POINT ( 'NONE', #19755 ) ;
#25382=CARTESIAN_POINT ( 'NONE',  ( 21.27250945180000130, -96.93384555780001222, 0.8126110531310000162 ) ) ;
#25383=EDGE_CURVE ( 'NONE', #17197, #11057, #12486, .T. ) ;
#25387=CARTESIAN_POINT ( 'NONE',  ( 29.72283664746381149, -92.84927079009172246, 6.841275840752675030 ) ) ;
#25405=CARTESIAN_POINT ( 'NONE',  ( -18.13877171349999884, -92.50000171950000549, -23.79299170569999688 ) ) ;
#25406=DIRECTION ( 'NONE',  ( 0.000000000000000000, 1.000000000000000000, 0.000000000000000000 ) ) ;
#25407=DIRECTION ( 'NONE',  ( 0.000000000000000000, -1.000000000000000000, 0.000000000000000000 ) ) ;
#25408=CARTESIAN_POINT ( 'NONE',  ( 7.345882526619999631, -101.1398235650000146, 13.52469188849999959 ) ) ;
#25411=CARTESIAN_POINT ( 'NONE',  ( -23.87973397989999924, -93.75379239759999450, -7.203585628490000836 ) ) ;
#25412=CARTESIAN_POINT ( 'NONE',  ( 12.03370358959999820, -98.60488091059998794, -15.63955140670000077 ) ) ;
#25418=DIRECTION ( 'NONE',  ( 0.5853721519882836288, 0.000000000000000000, 0.8107647276963926286 ) ) ;
#25427=ADVANCED_FACE ( 'NONE', ( #24873 ), #22550, .F. ) ;
#25428=CARTESIAN_POINT ( 'NONE',  ( 7.023258447689999961, -101.4254868729999970, 14.34178107630000021 ) ) ;
#25430=CARTESIAN_POINT ( 'NONE',  ( 7.635702898730000854, -101.6454117330000031, 14.06304778130000166 ) ) ;
#25436=CARTESIAN_POINT ( 'NONE',  ( -19.58257540287776166, -93.15741110474085929, -20.89612884129461179 ) ) ;
#25437=CARTESIAN_POINT ( 'NONE',  ( 0.3059185938709999553, -111.0000000000000000, 14.72672055670000013 ) ) ;
#25440=CARTESIAN_POINT ( 'NONE',  ( -17.09009608839999927, -99.55609322370000314, 3.193624944930000265 ) ) ;
#25444=CARTESIAN_POINT ( 'NONE',  ( 8.489585298007764180, -93.04141874247987687, -27.18617793450870579 ) ) ;
#25446=CARTESIAN_POINT ( 'NONE',  ( 13.12524984231539804, -92.96960399592983038, 27.53139692395792792 ) ) ;
#25451=CARTESIAN_POINT ( 'NONE',  ( -1.604070449259999753, -100.9197075889999979, -15.54198650660000069 ) ) ;
#25452=CARTESIAN_POINT ( 'NONE',  ( 23.79740151902118228, -92.74292563041596793, -19.07705719069169348 ) ) ;
#25456=PRESENTATION_STYLE_ASSIGNMENT (( #16559 ) ) ;
#25457=VERTEX_POINT ( 'NONE', #26619 ) ;
#25458=EDGE_CURVE ( 'NONE', #927, #1616, #4385, .T. ) ;
#25459=DIRECTION ( 'NONE',  ( 1.000000000000000000, 0.000000000000000000, 0.000000000000000000 ) ) ;
#25460=VERTEX_POINT ( 'NONE', #27209 ) ;
#25465=CARTESIAN_POINT ( 'NONE',  ( -11.20154639050000078, -94.96739875689999621, -21.25936308859999713 ) ) ;
#25475=ADVANCED_FACE ( 'NONE', ( #16113 ), #6808, .F. ) ;
#25477=CARTESIAN_POINT ( 'NONE',  ( -15.86429039329999924, -100.7450341080000129, 3.014304981200000455 ) ) ;
#25479=CARTESIAN_POINT ( 'NONE',  ( -6.236885381186699995, -101.3051320416518024, 14.59871265079590863 ) ) ;
#25481=DIRECTION ( 'NONE',  ( 0.000000000000000000, 1.000000000000000000, 0.000000000000000000 ) ) ;
#25484=VERTEX_POINT ( 'NONE', #22839 ) ;
#25486=CYLINDRICAL_SURFACE ( 'NONE', #27035, 18.64285714289999873 ) ;
#25489=CARTESIAN_POINT ( 'NONE',  ( 19.98296175649999995, -94.98812477599999227, 14.17692170039999944 ) ) ;
#25490=ORIENTED_EDGE ( 'NONE', *, *, #20788, .T. ) ;
#25492=B_SPLINE_SURFACE_WITH_KNOTS ( 'NONE', 5, 5, ( 
 ( #11960, #343, #20276, #3108, #15897, #16188, #22918, #20423, #18536 ),
 ( #27429, #20577, #5132, #11665, #27137, #641, #7479, #493, #9490 ),
 ( #13865, #4841, #13720, #9630, #16340, #25249, #7318, #5277, #7179 ),
 ( #2809, #9187, #932, #11819, #14165, #16044, #24948, #22768, #2516 ),
 ( #26845, #24655, #2957, #11372, #791, #18394, #23064, #20873, #9775 ),
 ( #6879, #15744, #4686, #8159, #1480, #12511, #23603, #8021, #7760 ) ),
 .UNSPECIFIED., .F., .F., .F.,
 ( 6, 6 ),
 ( 6, 3, 6 ),
 ( 22.76138574470000009, 41.46675637300000261 ),
 ( 0.000000000000000000, 0.2500000000000000000, 0.5000000000000000000 ),
 .UNSPECIFIED. ) ;
#25496=EDGE_CURVE ( 'NONE', #3132, #15723, #15646, .T. ) ;
#25499=ORIENTED_EDGE ( 'NONE', *, *, #16156, .F. ) ;
#25501=CARTESIAN_POINT ( 'NONE',  ( -5.733321685880000018, -101.0535396030000044, 14.50026364080000008 ) ) ;
#25506=CARTESIAN_POINT ( 'NONE',  ( 18.49452695338690233, -98.73470581664456347, -0.2805694970595983273 ) ) ;
#25512=CARTESIAN_POINT ( 'NONE',  ( -20.20541296980000112, -94.98812148390000232, 12.40015329510000086 ) ) ;
#25520=CARTESIAN_POINT ( 'NONE',  ( -13.09441083470000144, -92.84549618469999643, -23.96915825600000005 ) ) ;
#25521=FACE_OUTER_BOUND ( 'NONE', #8122, .T. ) ;
#25522=CARTESIAN_POINT ( 'NONE',  ( -7.931859541086235588, -99.76647888979522349, 15.39525047448377926 ) ) ;
#25528=EDGE_CURVE ( 'NONE', #2579, #2729, #2066, .T. ) ;
#25532=ORIENTED_EDGE ( 'NONE', *, *, #19026, .T. ) ;
#25533=CARTESIAN_POINT ( 'NONE',  ( -13.21936873900000009, -100.9405348700000076, -8.915374923630000836 ) ) ;
#25534=TOROIDAL_SURFACE ( 'NONE', #3211, 29.91857981989999971, 10.00000000000000000 ) ;
#25535=DIRECTION ( 'NONE',  ( 1.000000000000000000, 0.000000000000000000, 0.000000000000000000 ) ) ;
#25540=CARTESIAN_POINT ( 'NONE',  ( 7.269124901809999706, -101.2512678979999947, 13.34492656639999986 ) ) ;
#25541=EDGE_LOOP ( 'NONE', ( #13922, #22575, #5579, #24968, #26405, #349 ) ) ;
#25543=CARTESIAN_POINT ( 'NONE',  ( -28.51730836919999845, -92.58502644590001296, -2.516715198190000002 ) ) ;
#25544=CARTESIAN_POINT ( 'NONE',  ( 10.66329234459999853, -95.90105813160000992, -20.27129911129999940 ) ) ;
#25561=AXIS2_PLACEMENT_3D ( 'NONE', #10906, #8305, #26250 ) ;
#25562=CARTESIAN_POINT ( 'NONE',  ( 6.852899841210000176, -101.1617736559999940, 14.17211744369999948 ) ) ;
#25563=CARTESIAN_POINT ( 'NONE',  ( 13.64609657498295370, -96.57210918286925505, -16.84344588869538839 ) ) ;
#25565=CARTESIAN_POINT ( 'NONE',  ( 7.318052426040000391, -101.1822553929999913, 13.41977313900000013 ) ) ;
#25566=CARTESIAN_POINT ( 'NONE',  ( -11.25330392600000096, -94.84395216780001192, -20.59896425910000062 ) ) ;
#25569=B_SPLINE_CURVE_WITH_KNOTS ( 'NONE', 3,
 ( #3488, #14545, #27818, #19073, #14952, #23859, #25633, #28365, #5803, #23718, #3899, #23577, #8132, #16740, #5931, #3622, #5665, #19204, #19349, #17156, #12348, #10022, #21258, #1310, #21394, #10154, #12623, #8395, #16886, #15090, #28092, #26045, #17018, #7995, #27955, #25906, #1450, #21535, #6071, #26197, #12762, #21672, #1723, #6224, #3352, #17243, #15169, #28304, #24079, #4117, #8622, #17387, #19707, #17529, #17676, #28452, #1671, #3839, #10647 ),
 .UNSPECIFIED., .F., .F.,
 ( 4, 2, 1, 1, 2, 2, 2, 1, 1, 1, 2, 2, 2, 2, 2, 2, 2, 1, 1, 2, 2, 2, 2, 1, 2, 2, 2, 1, 2, 2, 2, 2, 2, 4 ),
 ( 0.000000000000000000, 0.06250000000013401780, 0.09375000000019519109, 0.1093750000002202127, 0.1171875000002372408, 0.1250000000002542688, 0.1875000000004052869, 0.2187500000004812262, 0.2343750000005198064, 0.2421875000005390965, 0.2460937500005491718, 0.2500000000005592748, 0.3125000000005516698, 0.3437500000005482281, 0.3750000000005447864, 0.4375000000005389578, 0.4687500000005295764, 0.4843750000005255796, 0.4921875000005235812, 0.4960937500005233591, 0.5000000000005231371, 0.5625000000004112266, 0.5937500000003553824, 0.6093750000003334000, 0.6171875000003288481, 0.6250000000003242961, 0.6875000000002615685, 0.7187500000002239320, 0.7343750000002052802, 0.7500000000001865175, 0.8125000000001336709, 0.8437500000001117995, 0.8750000000000900391, 1.000000000000000000 ),
 .UNSPECIFIED. ) ;
#25570=CARTESIAN_POINT ( 'NONE',  ( 26.68170793902356763, -93.00000166546708158, -11.33666327679907049 ) ) ;
#25583=AXIS2_PLACEMENT_3D ( 'NONE', #11273, #28337, #10679 ) ;
#25585=CARTESIAN_POINT ( 'NONE',  ( 0.5752469741175000317, -100.9229461903683926, -16.55552124226701594 ) ) ;
#25587=DIRECTION ( 'NONE',  ( -0.9950133697301837277, 0.000000000000000000, 0.09974163653251839901 ) ) ;
#25588=CARTESIAN_POINT ( 'NONE',  ( 13.40137751648780373, -92.68577957619636720, 27.39809740741056743 ) ) ;
#25589=CARTESIAN_POINT ( 'NONE',  ( -11.69653564380000077, -94.52419443349998573, -20.97821456950000041 ) ) ;
#25592=CARTESIAN_POINT ( 'NONE',  ( -18.26050467580000003, -97.41004717059999507, 11.26842931770000078 ) ) ;
#25593=CARTESIAN_POINT ( 'NONE',  ( 22.66360738736820579, -92.65509297698689295, 15.93307463348966202 ) ) ;
#25597=ORIENTED_EDGE ( 'NONE', *, *, #3582, .F. ) ;
#25599=VERTEX_POINT ( 'NONE', #14648 ) ;
#25601=AXIS2_PLACEMENT_3D ( 'NONE', #26801, #19926, #22425 ) ;
#25603=B_SPLINE_CURVE_WITH_KNOTS ( 'NONE', 3,
 ( #10493, #28023, #19408, #14744, #23516, #21738 ),
 .UNSPECIFIED., .F., .F.,
 ( 4, 2, 4 ),
 ( 0.000000000000000000, 0.5000000000000000000, 1.000000000000000000 ),
 .UNSPECIFIED. ) ;
#25611=CARTESIAN_POINT ( 'NONE',  ( -1.315109685649999971, -92.50000000000000000, -30.47163412939999816 ) ) ;
#25617=ORIENTED_EDGE ( 'NONE', *, *, #13509, .F. ) ;
#25619=CARTESIAN_POINT ( 'NONE',  ( -15.42268928930000094, -101.5369814700000148, 4.259183639510000674 ) ) ;
#25620=CARTESIAN_POINT ( 'NONE',  ( -16.03654356910000089, -101.2023582690000012, 3.165913905190000044 ) ) ;
#25631=ORIENTED_EDGE ( 'NONE', *, *, #23078, .T. ) ;
#25633=CARTESIAN_POINT ( 'NONE',  ( 6.990562848071419033, -100.1406256088127122, 15.70413603688146331 ) ) ;
#25640=CARTESIAN_POINT ( 'NONE',  ( -18.29385458159615396, -98.30143183942811902, 5.155709219538591626 ) ) ;
#25642=CARTESIAN_POINT ( 'NONE',  ( 28.55300759750000239, -92.83702889490000132, 8.518421555419999791 ) ) ;
#25643=CARTESIAN_POINT ( 'NONE',  ( -6.181362597580000617, -101.1716782170000073, 14.46875015949999899 ) ) ;
#25648=CARTESIAN_POINT ( 'NONE',  ( 23.54313657600000198, -94.98812477599999227, -6.784142512209999865 ) ) ;
#25651=VERTEX_POINT ( 'NONE', #18615 ) ;
#25653=CARTESIAN_POINT ( 'NONE',  ( 19.84870995880000066, -97.83383802310000021, 2.182632968150000075 ) ) ;
#25654=CARTESIAN_POINT ( 'NONE',  ( -20.80195327079999856, -93.01591283300000157, 16.29683310170000254 ) ) ;
#25661=AXIS2_PLACEMENT_3D ( 'NONE', #3217, #23721, #28226 ) ;
#25665=DIRECTION ( 'NONE',  ( 0.8172561201429201505, 0.000000000000000000, 0.5762746169049446365 ) ) ;
#25670=MANIFOLD_SOLID_BREP ( 'Rotational Bodies', #17472 ) ;
#25673=EDGE_CURVE ( 'NONE', #18774, #24426, #11461, .T. ) ;
#25676=CARTESIAN_POINT ( 'NONE',  ( 7.120468124967428203, -92.55389105865127419, -28.82010846582078045 ) ) ;
#25680=CARTESIAN_POINT ( 'NONE',  ( -13.25127150620000016, -101.2490009469999990, -9.112328469719999546 ) ) ;
#25682=CARTESIAN_POINT ( 'NONE',  ( -7.876988035330001026, -100.4071172650000108, 14.82857468579999960 ) ) ;
#25684=CARTESIAN_POINT ( 'NONE',  ( -1.283017171710000071, -101.3150694429999987, -16.20107591070000197 ) ) ;
#25686=CARTESIAN_POINT ( 'NONE',  ( 7.602022623930000833, -101.5367116919999972, 14.07888202740000239 ) ) ;
#25689=CARTESIAN_POINT ( 'NONE',  ( -29.91145159459999903, -92.50000467790000869, -0.6532164815390000268 ) ) ;
#25691=CARTESIAN_POINT ( 'NONE',  ( 11.33780749240000141, -100.8733984769999950, -10.89600342719999837 ) ) ;
#25694=CARTESIAN_POINT ( 'NONE',  ( 11.58372824880000174, -101.1292389529999980, -10.30936447240000042 ) ) ;
#25696=CARTESIAN_POINT ( 'NONE',  ( -17.78957887869999865, -94.03833868319999567, 17.10921786280000134 ) ) ;
#25697=CARTESIAN_POINT ( 'NONE',  ( -18.23251993885847710, -92.52498922770502077, 24.45057987636252150 ) ) ;
#25708=CARTESIAN_POINT ( 'NONE',  ( 6.745190077079999291, -100.5229262450000078, 15.47590599200000128 ) ) ;
#25709=CARTESIAN_POINT ( 'NONE',  ( 13.81100091409999919, -99.92967571559999840, -10.51865105429999936 ) ) ;
#25710=CARTESIAN_POINT ( 'NONE',  ( -11.46795327739999948, -94.84072973010000851, -21.30482454299999873 ) ) ;
#25713=FACE_OUTER_BOUND ( 'NONE', #2479, .T. ) ;
#25714=CARTESIAN_POINT ( 'NONE',  ( -6.439729480049999566, -101.2530993010000060, 13.76171823350000167 ) ) ;
#25715=B_SPLINE_CURVE_WITH_KNOTS ( 'NONE', 3,
 ( #6617, #26432, #15476, #12851, #8500, #10809, #6768, #15629, #24528, #13444, #24387, #15326, #22201, #6318, #4565, #26730, #26147, #19854, #2245, #2113, #28463, #8635, #10946, #20006, #22352, #19719, #28605, #17542, #24243, #4279 ),
 .UNSPECIFIED., .F., .F.,
 ( 4, 1, 1, 1, 1, 2, 2, 1, 1, 1, 1, 2, 2, 2, 1, 1, 1, 1, 2, 2, 4 ),
 ( 0.000000000000000000, 0.1249999999999575895, 0.1874999999999370504, 0.2187499999999273637, 0.2343749999999251155, 0.2421874999999223954, 0.2499999999999197309, 0.3749999999998104294, 0.4374999999997585820, 0.4687499999997326583, 0.4843749999997227218, 0.4921874999997177258, 0.4999999999997127298, 0.6249999999996563860, 0.6874999999996247446, 0.7187499999996056488, 0.7343749999995959898, 0.7421874999995905497, 0.7460937499995909938, 0.7499999999995914379, 1.000000000000000000 ),
 .UNSPECIFIED. ) ;
#25716=ORIENTED_EDGE ( 'NONE', *, *, #8198, .F. ) ;
#25718=CARTESIAN_POINT ( 'NONE',  ( -5.360408304419999936, -101.0356131030000029, 14.51726283890000069 ) ) ;
#25719=DIRECTION ( 'NONE',  ( 1.000000000000000000, 0.000000000000000000, 0.000000000000000000 ) ) ;
#25720=ORIENTED_EDGE ( 'NONE', *, *, #15323, .F. ) ;
#25722=CARTESIAN_POINT ( 'NONE',  ( 0.5820789627235478658, -100.8945630385067176, -16.57764313316371130 ) ) ;
#25724=CARTESIAN_POINT ( 'NONE',  ( 13.30333552573421940, -92.74292563041898063, 27.44579556150942423 ) ) ;
#25726=CARTESIAN_POINT ( 'NONE',  ( -8.303419408699999948, -99.91102932029998840, 14.75134094139999874 ) ) ;
#25728=EDGE_CURVE ( 'NONE', #18453, #7330, #26273, .T. ) ;
#25729=CARTESIAN_POINT ( 'NONE',  ( 11.86104588439999930, -101.2306315440000049, -11.05401200120000027 ) ) ;
#25740=EDGE_CURVE ( 'NONE', #22807, #14760, #12741, .T. ) ;
#25747=ORIENTED_EDGE ( 'NONE', *, *, #12503, .F. ) ;
#25756=CARTESIAN_POINT ( 'NONE',  ( -15.29387583709999809, -101.2458775890000027, 4.542988961549999871 ) ) ;
#25757=CARTESIAN_POINT ( 'NONE',  ( -16.40085562500000194, -100.7638431670000045, 3.096686113970000154 ) ) ;
#25759=CARTESIAN_POINT ( 'NONE',  ( -6.208760515565253435, -101.2404586421421158, 14.53288061996913783 ) ) ;
#25760=ORIENTED_EDGE ( 'NONE', *, *, #11854, .T. ) ;
#25761=CARTESIAN_POINT ( 'NONE',  ( 16.08037959500000014, -101.3150700380000018, 2.354223078750000031 ) ) ;
#25762=LINE ( 'NONE', #5791, #10630 ) ;
#25763=EDGE_CURVE ( 'NONE', #23842, #25778, #3485, .T. ) ;
#25765=CARTESIAN_POINT ( 'NONE',  ( -7.511256938544575767, -101.2021794472616989, 14.51835494349533207 ) ) ;
#25773=EDGE_CURVE ( 'NONE', #10772, #4529, #3147, .T. ) ;
#25775=CARTESIAN_POINT ( 'NONE',  ( -7.879410208250000380, -111.0000000000000000, 15.46934584979999983 ) ) ;
#25778=VERTEX_POINT ( 'NONE', #22210 ) ;
#25783=FACE_OUTER_BOUND ( 'NONE', #8649, .T. ) ;
#25785=CARTESIAN_POINT ( 'NONE',  ( 11.86373224459999776, -101.2530993010000060, -9.493548918760000177 ) ) ;
#25790=CARTESIAN_POINT ( 'NONE',  ( 22.78264860270000014, -94.59276292389999696, -6.873201011689999085 ) ) ;
#25792=ORIENTED_EDGE ( 'NONE', *, *, #9296, .T. ) ;
#25793=CARTESIAN_POINT ( 'NONE',  ( -20.54204567169999862, -95.55433883429999753, -9.451949542510000413 ) ) ;
#25794=CARTESIAN_POINT ( 'NONE',  ( 15.80921915986327875, -101.6077248516952665, 2.654137683538275727 ) ) ;
#25795=CARTESIAN_POINT ( 'NONE',  ( -20.72181756220000182, -93.63285492290000889, 14.13430432360000211 ) ) ;
#25797=CARTESIAN_POINT ( 'NONE',  ( 23.96026145669999607, -92.49999926799999628, -16.90273770479999982 ) ) ;
#25801=CARTESIAN_POINT ( 'NONE',  ( 29.76135012335695151, -92.72059904821338705, 6.671735646977375644 ) ) ;
#25802=CARTESIAN_POINT ( 'NONE',  ( 9.119802927630001221, -98.28914429610000525, 16.69368728350000097 ) ) ;
#25819=CARTESIAN_POINT ( 'NONE',  ( -13.12062273610000140, -101.6095085860000040, -9.209289609949999900 ) ) ;
#25821=CARTESIAN_POINT ( 'NONE',  ( -7.879410026489999552, -99.92967571559999840, 15.46934602219999988 ) ) ;
#25825=DIRECTION ( 'NONE',  ( -0.8775825618903722036, 0.000000000000000000, 0.4794255386042041156 ) ) ;
#25826=CARTESIAN_POINT ( 'NONE',  ( -20.20543299319999875, -94.98810756820000734, 12.40017484579999874 ) ) ;
#25827=CARTESIAN_POINT ( 'NONE',  ( 7.332920525790000532, -101.1404853350000081, 13.53079052370000035 ) ) ;
#25829=CARTESIAN_POINT ( 'NONE',  ( 13.33933447234251801, -100.8738282928510017, -9.887453640032017432 ) ) ;
#25830=CARTESIAN_POINT ( 'NONE',  ( -25.54375670880000015, -93.49005502550001268, -5.768728999770000421 ) ) ;
#25833=AXIS2_PLACEMENT_3D ( 'NONE', #14610, #3550, #12405 ) ;
#25837=CARTESIAN_POINT ( 'NONE',  ( -17.87039757315234567, -92.59033770622343695, 24.71676568516515715 ) ) ;
#25839=EDGE_CURVE ( 'NONE', #7941, #6448, #8107, .T. ) ;
#25841=CARTESIAN_POINT ( 'NONE',  ( -0.02519810411110000314, -101.1617736559999940, -15.74199841589999771 ) ) ;
#25843=CARTESIAN_POINT ( 'NONE',  ( 16.08037959500000014, -101.3150700380000018, 2.354223078750000031 ) ) ;
#25846=EDGE_LOOP ( 'NONE', ( #14764, #1415, #23159, #106, #16162, #9562, #2799 ) ) ;
#25848=CARTESIAN_POINT ( 'NONE',  ( 6.647943390380000039, -101.0678230150000019, 14.35910459099999947 ) ) ;
#25849=CARTESIAN_POINT ( 'NONE',  ( 15.53144063390000085, -101.3256027139999986, 3.435397172430000090 ) ) ;
#25852=CARTESIAN_POINT ( 'NONE',  ( -6.761572831579999665, -97.58045781590000445, 18.83461070039999896 ) ) ;
#25853=CARTESIAN_POINT ( 'NONE',  ( 3.387657239720000213, -92.79907188619999658, -28.90154850299999723 ) ) ;
#25854=ADVANCED_FACE ( 'NONE', ( #24980 ), #25288, .F. ) ;
#25856=CARTESIAN_POINT ( 'NONE',  ( -6.902767321779999854, -101.4121386959999995, 14.40917022280000026 ) ) ;
#25859=CARTESIAN_POINT ( 'NONE',  ( -16.98520236649999759, -99.83167676440000093, 3.436659022809999797 ) ) ;
#25861=CARTESIAN_POINT ( 'NONE',  ( -0.8544872754590000508, -101.1411470150000014, -15.36633732259999974 ) ) ;
#25862=CARTESIAN_POINT ( 'NONE',  ( 6.888451955769999913, -99.53431386179998697, 15.99365555089999802 ) ) ;
#25864=CARTESIAN_POINT ( 'NONE',  ( 13.98842255709134896, -92.52640451557674339, 27.10303198118710455 ) ) ;
#25867=CARTESIAN_POINT ( 'NONE',  ( 0.3059185938709999553, -92.50000000000000000, 14.72672055670000013 ) ) ;
#25869=CARTESIAN_POINT ( 'NONE',  ( 11.23915397940000105, -100.8869817940000075, -10.91500585829999892 ) ) ;
#25872=( NAMED_UNIT ( * ) PLANE_ANGLE_UNIT ( ) SI_UNIT ( $, .RADIAN. ) );
#25874=FACE_OUTER_BOUND ( 'NONE', #17567, .T. ) ;
#25880=CARTESIAN_POINT ( 'NONE',  ( -29.29590816570000200, -92.50000947299999154, 6.421684369280000304 ) ) ;
#25884=CARTESIAN_POINT ( 'NONE',  ( -17.88989799939055203, -97.43430234701037307, -10.14936231854670190 ) ) ;
#25886=ORIENTED_EDGE ( 'NONE', *, *, #24639, .F. ) ;
#25889=EDGE_CURVE ( 'NONE', #13918, #20274, #21905, .T. ) ;
#25893=B_SPLINE_SURFACE_WITH_KNOTS ( 'NONE', 5, 5, ( 
 ( #12555, #15020, #25979, #6005, #21326, #6293, #16958, #26407, #15160 ),
 ( #15302, #8329, #28585, #25849, #12694, #21608, #10501, #19552, #4109 ),
 ( #3557, #23934, #21467, #3973, #28168, #5870, #24069, #3832, #12980 ),
 ( #1794, #23794, #19415, #1942, #28295, #10783, #12412, #26122, #6150 ),
 ( #23650, #1385, #1522, #28031, #10366, #19280, #8200, #12833, #21745 ),
 ( #10640, #28441, #14498, #23399, #12435, #26150, #6172, #28048, #21770 ),
 ( #16977, #17562, #1841, #21650, #19325, #1565, #26021, #28200, #19598 ),
 ( #28762, #26456, #8234, #8802, #15201, #23831, #10535, #19453, #6489 ),
 ( #15348, #4304, #13177, #22087, #19877, #17714, #4592, #6934, #257 ),
 ( #15800, #9097, #692, #9545, #22670, #20322, #18447, #24994, #2862 ),
 ( #393, #27190, #24707, #9242, #26897, #22530, #15651, #4889, #5029 ),
 ( #27331, #7229, #16094, #16237, #27041, #13621, #20034, #18000, #18299 ) ),
 .UNSPECIFIED., .F., .F., .F.,
 ( 6, 3, 3, 6 ),
 ( 6, 3, 6 ),
 ( 3.852920539479999906, 4.834764074430000669, 6.134713715070000184, 8.383984506260000913 ),
 ( 0.000000000000000000, 0.2500000000000000000, 0.5000000000000000000 ),
 .UNSPECIFIED. ) ;
#25896=CARTESIAN_POINT ( 'NONE',  ( -12.03351515999999855, -100.7833805400000102, -10.41203369199999962 ) ) ;
#25898=CARTESIAN_POINT ( 'NONE',  ( -7.853002983444719476, -100.5798851023766929, 14.89419455703112938 ) ) ;
#25899=ORIENTED_EDGE ( 'NONE', *, *, #4911, .T. ) ;
#25906=CARTESIAN_POINT ( 'NONE',  ( 6.656280120269700618, -101.0610180774001208, 15.05062505483333979 ) ) ;
#25908=ORIENTED_EDGE ( 'NONE', *, *, #3588, .T. ) ;
#25909=CARTESIAN_POINT ( 'NONE',  ( -18.28476853637538113, -98.31192523452679666, 5.137975449739348832 ) ) ;
#25912=CARTESIAN_POINT ( 'NONE',  ( 26.25674219109999896, -93.16461300810000523, 10.85501170439999896 ) ) ;
#25918=CARTESIAN_POINT ( 'NONE',  ( 0.2284267155709999997, -92.50000000000000000, -29.91770779450000362 ) ) ;
#25927=CARTESIAN_POINT ( 'NONE',  ( 13.55377673239999936, -100.4650220110000021, -9.985834839249999817 ) ) ;
#25929=CARTESIAN_POINT ( 'NONE',  ( 23.88294446200000110, -92.63555401869999173, -18.57671364879999842 ) ) ;
#25936=CARTESIAN_POINT ( 'NONE',  ( -6.665307709260000379, -93.00000000000000000, -13.13558364449999871 ) ) ;
#25943=ORIENTED_EDGE ( 'NONE', *, *, #22086, .F. ) ;
#25946=AXIS2_PLACEMENT_3D ( 'NONE', #6547, #2328, #24619 ) ;
#25950=CARTESIAN_POINT ( 'NONE',  ( 10.58737011899999914, -97.65299964609999961, 16.87371021290000073 ) ) ;
#25952=B_SPLINE_CURVE_WITH_KNOTS ( 'NONE', 3,
 ( #13449, #27168, #22355, #20613, #375, #20763, #9219, #7065, #2399, #20161, #16074, #9079, #27314, #18424, #17982, #22799, #6914, #15929 ),
 .UNSPECIFIED., .F., .F.,
 ( 4, 2, 2, 2, 1, 1, 1, 1, 2, 2, 4 ),
 ( 0.000000000000000000, 0.2500000000000573430, 0.3750000000000868194, 0.4375000000001025846, 0.4687500000001104672, 0.4843750000001151856, 0.4921875000001167955, 0.4960937500001167955, 0.4980468750001167955, 0.5000000000001167955, 1.000000000000000000 ),
 .UNSPECIFIED. ) ;
#25955=CARTESIAN_POINT ( 'NONE',  ( 0.03691039440750000511, -93.36531860680000250, 26.17328399250000004 ) ) ;
#25962=CARTESIAN_POINT ( 'NONE',  ( -25.53339762659999934, -93.24058218849999946, -5.837366266040000085 ) ) ;
#25967=CARTESIAN_POINT ( 'NONE',  ( -18.18547914559999867, -94.42120323109999447, 17.31458345580000113 ) ) ;
#25968=CARTESIAN_POINT ( 'NONE',  ( -19.92371129995309076, -92.49999999999992895, 21.06559270865390587 ) ) ;
#25969=ORIENTED_EDGE ( 'NONE', *, *, #14414, .T. ) ;
#25972=CARTESIAN_POINT ( 'NONE',  ( 0.03568166535660000083, -101.2902355740000075, -15.92847312690000372 ) ) ;
#25977=VERTEX_POINT ( 'NONE', #17081 ) ;
#25978=CARTESIAN_POINT ( 'NONE',  ( 6.186462384450000407, -100.1275643909999928, 15.45527146859999945 ) ) ;
#25979=CARTESIAN_POINT ( 'NONE',  ( 15.60714071820000015, -101.4254868729999970, 3.380050261510000098 ) ) ;
#25984=CARTESIAN_POINT ( 'NONE',  ( -0.7205257401540000606, -101.1889999979999999, -15.98376809950000066 ) ) ;
#25985=ORIENTED_EDGE ( 'NONE', *, *, #4474, .F. ) ;
#25986=CARTESIAN_POINT ( 'NONE',  ( 8.236226396380001091, -93.85715850789999593, -23.50030299510000020 ) ) ;
#25991=CARTESIAN_POINT ( 'NONE',  ( 15.74335372269999844, -111.0000000000000000, 2.854262350119999958 ) ) ;
#25998=CARTESIAN_POINT ( 'NONE',  ( 16.20707181140645758, -94.69873403835963188, 17.23731209724227753 ) ) ;
#26005=CARTESIAN_POINT ( 'NONE',  ( 0.000000000000000000, -92.50000000000000000, 0.000000000000000000 ) ) ;
#26010=ORIENTED_EDGE ( 'NONE', *, *, #13273, .F. ) ;
#26013=CIRCLE ( 'NONE', #28336, 18.64285714289999518 ) ;
#26014=CARTESIAN_POINT ( 'NONE',  ( -29.00049327840000046, -92.49537389370000540, 4.812555014239999096 ) ) ;
#26015=CARTESIAN_POINT ( 'NONE',  ( -0.7149044700954795273, -101.3051320416606700, -15.85906875946512251 ) ) ;
#26017=VECTOR ( 'NONE', #11948, 1000.000000000000000 ) ;
#26021=CARTESIAN_POINT ( 'NONE',  ( 15.28250192019999965, -100.7707614970000094, 4.221087105419999652 ) ) ;
#26024=CARTESIAN_POINT ( 'NONE',  ( -16.55071332594993549, -98.16872836274220049, -10.59832500731132754 ) ) ;
#26029=CARTESIAN_POINT ( 'NONE',  ( -15.54889200169999874, -101.4254868860000016, 3.639708781509999991 ) ) ;
#26033=CARTESIAN_POINT ( 'NONE',  ( -12.00940321250000054, -100.8772072149999985, -10.26826983859999842 ) ) ;
#26034=CARTESIAN_POINT ( 'NONE',  ( 24.61545324444739435, -93.04141874247781629, 14.32622737458234496 ) ) ;
#26035=CARTESIAN_POINT ( 'NONE',  ( -7.533632261058696322, -101.1742791176865097, 14.53131762976900276 ) ) ;
#26039=EDGE_CURVE ( 'NONE', #22634, #8673, #18307, .T. ) ;
#26045=CARTESIAN_POINT ( 'NONE',  ( 6.661515206416465773, -100.9570234915945122, 15.13779097725072376 ) ) ;
#26051=CARTESIAN_POINT ( 'NONE',  ( 29.30603805220000169, -92.54628605920001405, 7.013473232189999962 ) ) ;
#26052=FACE_OUTER_BOUND ( 'NONE', #1733, .T. ) ;
#26053=VERTEX_POINT ( 'NONE', #9451 ) ;
#26054=CARTESIAN_POINT ( 'NONE',  ( 12.38290840660000036, -101.0875971110000080, -9.170880648609999852 ) ) ;
#26060=CARTESIAN_POINT ( 'NONE',  ( -22.03947464310000015, -92.99999932709999939, -20.07685987300000008 ) ) ;
#26063=CARTESIAN_POINT ( 'NONE',  ( -14.99089894709999982, -98.53908914310000000, -11.25712186019999983 ) ) ;
#26064=CARTESIAN_POINT ( 'NONE',  ( 12.92698146070000043, -100.9678331089999972, -9.732993700310000662 ) ) ;
#26066=CARTESIAN_POINT ( 'NONE',  ( 24.04045223339999993, -92.49537389370000540, -16.91880470280000281 ) ) ;
#26070=ORIENTED_EDGE ( 'NONE', *, *, #25528, .T. ) ;
#26071=CARTESIAN_POINT ( 'NONE',  ( 0.000000000000000000, -92.50000000000000000, 29.91857981989999971 ) ) ;
#26072=EDGE_CURVE ( 'NONE', #22767, #3830, #539, .T. ) ;
#26074=DIRECTION ( 'NONE',  ( 0.4794255386042040601, 0.000000000000000000, 0.8775825618903720926 ) ) ;
#26079=ADVANCED_FACE ( 'NONE', ( #14809 ), #25486, .F. ) ;
#26090=CARTESIAN_POINT ( 'NONE',  ( 12.15866047070000100, -97.18712516009998126, 17.03251418340000001 ) ) ;
#26091=CARTESIAN_POINT ( 'NONE',  ( -16.07598155610000035, -92.73227869829999293, -23.64671446510000052 ) ) ;
#26092=CARTESIAN_POINT ( 'NONE',  ( -8.110006665580000274, -99.58396362730000817, 15.35220468210000178 ) ) ;
#26095=CARTESIAN_POINT ( 'NONE',  ( -29.71794281087073841, -92.74292563043081827, 6.862529067643276193 ) ) ;
#26100=CARTESIAN_POINT ( 'NONE',  ( 13.50420993948647741, -100.6338045025844821, -9.984825884511051797 ) ) ;
#26109=CARTESIAN_POINT ( 'NONE',  ( 11.70455088819999823, -111.0000000000000000, 8.942783294160001617 ) ) ;
#26110=CARTESIAN_POINT ( 'NONE',  ( -20.65988748905770578, -93.37625791770756223, 15.48159536565925798 ) ) ;
#26113=CARTESIAN_POINT ( 'NONE',  ( -0.09837475146920000857, -101.5369810359999860, -15.99989550839999985 ) ) ;
#26121=CARTESIAN_POINT ( 'NONE',  ( 6.782523189059999957, -100.1981337080000003, 15.56999851120000145 ) ) ;
#26122=CARTESIAN_POINT ( 'NONE',  ( 14.90817938300000023, -101.1402801299999936, 3.615773941519999646 ) ) ;
#26123=CARTESIAN_POINT ( 'NONE',  ( -5.868160160552678306, -97.38870237642460381, 19.77461684056510194 ) ) ;
#26126=EDGE_CURVE ( 'NONE', #8703, #20241, #17241, .T. ) ;
#26132=CARTESIAN_POINT ( 'NONE',  ( 7.776016120819999600, -93.59856727299998624, -24.15955163539999617 ) ) ;
#26139=CARTESIAN_POINT ( 'NONE',  ( -12.46749392793309319, -101.2637735887273038, -10.49728468171560714 ) ) ;
#26142=CARTESIAN_POINT ( 'NONE',  ( -1.017451505570000192, -101.1130130960000031, -15.39193785830000039 ) ) ;
#26146=TOROIDAL_SURFACE ( 'NONE', #27567, 16.50000000000000000, 5.500000000000000000 ) ;
#26147=CARTESIAN_POINT ( 'NONE',  ( -20.40343802174961496, -92.66972459458344247, -22.67045984017129001 ) ) ;
#26148=CARTESIAN_POINT ( 'NONE',  ( -14.42556421679999978, -93.00000000000000000, -2.978755036369999942 ) ) ;
#26150=CARTESIAN_POINT ( 'NONE',  ( 15.27533372839999792, -100.8772072149999985, 4.040706681419999668 ) ) ;
#26158=CARTESIAN_POINT ( 'NONE',  ( 26.73328265790000202, -93.00000450890000536, -12.41349335419999989 ) ) ;
#26173=ORIENTED_EDGE ( 'NONE', *, *, #5667, .F. ) ;
#26174=CARTESIAN_POINT ( 'NONE',  ( -14.62247892739999955, -92.50000000000000000, -26.76626813769999913 ) ) ;
#26181=CARTESIAN_POINT ( 'NONE',  ( 20.17093527805420194, -98.28141828962287718, -1.154278920403048803 ) ) ;
#26182=CARTESIAN_POINT ( 'NONE',  ( -12.43709190490000083, -101.4829589650000088, -10.26829550889999965 ) ) ;
#26185=CARTESIAN_POINT ( 'NONE',  ( -7.616929725699291609, -101.0610180770348450, 14.58800058767319463 ) ) ;
#26187=EDGE_CURVE ( 'NONE', #19071, #2738, #16453, .T. ) ;
#26192=ORIENTED_EDGE ( 'NONE', *, *, #6214, .T. ) ;
#26194=PRODUCT ( 'Coolant Impeller Vanes', 'Coolant Impeller Vanes', '', ( #2334 ) ) ;
#26197=CARTESIAN_POINT ( 'NONE',  ( 6.665674591485936773, -101.1884902310438861, 14.93720712614567248 ) ) ;
#26199=ORIENTED_EDGE ( 'NONE', *, *, #25050, .F. ) ;
#26200=CARTESIAN_POINT ( 'NONE',  ( -14.21627981196383139, -94.10917102368060227, -21.62117019558515452 ) ) ;
#26203=DIRECTION ( 'NONE',  ( 0.1241703988689521337, 0.000000000000000000, -0.9922609092596188507 ) ) ;
#26204=CARTESIAN_POINT ( 'NONE',  ( 12.77500156440000012, -92.50000000000000000, 27.05403395929999988 ) ) ;
#26205=ORIENTED_EDGE ( 'NONE', *, *, #16076, .F. ) ;
#26207=DIRECTION ( 'NONE',  ( 0.4794255386042041156, 0.000000000000000000, 0.8775825618903722036 ) ) ;
#26212=CARTESIAN_POINT ( 'NONE',  ( -18.75204558950000333, -92.67327634539999792, -20.60858423150000363 ) ) ;
#26214=EDGE_LOOP ( 'NONE', ( #15225, #22141, #14802, #10344 ) ) ;
#26216=CARTESIAN_POINT ( 'NONE',  ( 13.68203184070000233, -100.2522625769999962, -10.11858478029999908 ) ) ;
#26223=ADVANCED_FACE ( 'NONE', ( #15086, #21809 ), #6065, .F. ) ;
#26227=CARTESIAN_POINT ( 'NONE',  ( -0.1866349815764706266, -92.68577957618185792, -30.49947259001435995 ) ) ;
#26233=CONICAL_SURFACE ( 'NONE', #8541, 13.13304743849999667, 0.9119902906770002149 ) ;
#26240=CARTESIAN_POINT ( 'NONE',  ( -12.66827223139999958, -101.1130130960000031, -8.801240666549999148 ) ) ;
#26242=CARTESIAN_POINT ( 'NONE',  ( -13.34153245340000105, -93.00000000000000000, 27.42724032409999779 ) ) ;
#26243=CARTESIAN_POINT ( 'NONE',  ( 0.000000000000000000, -101.2530993010000060, 0.000000000000000000 ) ) ;
#26244=CARTESIAN_POINT ( 'NONE',  ( -1.788617204129999916, -93.67869433870001217, 24.94025035040000304 ) ) ;
#26248=AXIS2_PLACEMENT_3D ( 'NONE', #856, #27505, #14238 ) ;
#26250=DIRECTION ( 'NONE',  ( 0.4438776720071309079, 0.000000000000000000, 0.8960873909912636659 ) ) ;
#26255=CARTESIAN_POINT ( 'NONE',  ( -16.40085562500000194, -100.7638431670000045, 3.096686113970000154 ) ) ;
#26258=EDGE_CURVE ( 'NONE', #842, #14037, #22114, .T. ) ;
#26260=CARTESIAN_POINT ( 'NONE',  ( -13.30343089850000027, -92.51541830560000790, 26.96082632650000122 ) ) ;
#26263=CARTESIAN_POINT ( 'NONE',  ( 26.37318901919999803, -93.00000450890000536, 13.16123549989999830 ) ) ;
#26264=AXIS2_PLACEMENT_3D ( 'NONE', #18556, #25406, #5435 ) ;
#26265=CARTESIAN_POINT ( 'NONE',  ( 0.9481071690910000127, -99.94549701829998867, -16.87515825230000033 ) ) ;
#26266=CARTESIAN_POINT ( 'NONE',  ( 15.73111530680000314, -101.4254868690000109, 2.747748852119999974 ) ) ;
#26270=CARTESIAN_POINT ( 'NONE',  ( 6.377887625069999622, -101.0147083550000104, 14.18006541960000000 ) ) ;
#26271=CARTESIAN_POINT ( 'NONE',  ( -16.09259912896104439, -92.55138318345946402, -24.01119014493966120 ) ) ;
#26272=CARTESIAN_POINT ( 'NONE',  ( -3.982536363037985971, -95.75133628813770770, 22.38549364098651395 ) ) ;
#26273=CIRCLE ( 'NONE', #23935, 5.000000000000000888 ) ;
#26280=CARTESIAN_POINT ( 'NONE',  ( 4.740176215359999112, -93.16461275549998788, -28.01390021799999985 ) ) ;
#26282=CARTESIAN_POINT ( 'NONE',  ( -13.14566783280000095, -99.53431386179998697, -11.42099844400000030 ) ) ;
#26285=CARTESIAN_POINT ( 'NONE',  ( -12.72085913849602257, -100.6644468681186027, -10.92796509865996235 ) ) ;
#26288=CARTESIAN_POINT ( 'NONE',  ( 23.56065605869999757, -94.89197151660000884, -2.367189373290000010 ) ) ;
#26290=CARTESIAN_POINT ( 'NONE',  ( -0.9479808564000000715, -101.5026188610000020, -15.99452317279999924 ) ) ;
#26296=EDGE_CURVE ( 'NONE', #22947, #16053, #21899, .T. ) ;
#26297=FACE_OUTER_BOUND ( 'NONE', #26982, .T. ) ;
#26298=CARTESIAN_POINT ( 'NONE',  ( 16.32098426875123209, -94.64445995926946864, 17.22619538277506379 ) ) ;
#26301=VECTOR ( 'NONE', #21201, 1000.000000000000000 ) ;
#26311=DIRECTION ( 'NONE',  ( 0.000000000000000000, 1.000000000000000000, 0.000000000000000000 ) ) ;
#26314=ORIENTED_EDGE ( 'NONE', *, *, #3341, .F. ) ;
#26315=CARTESIAN_POINT ( 'NONE',  ( -19.83493014842161273, -96.36359511561902025, -9.389546401069701176 ) ) ;
#26323=DIRECTION ( 'NONE',  ( -0.2689078219309835593, 0.000000000000000000, 0.9631659168099411250 ) ) ;
#26325=CARTESIAN_POINT ( 'NONE',  ( -13.21936873900000009, -100.9405348700000076, -8.915374923630000836 ) ) ;
#26328=CARTESIAN_POINT ( 'NONE',  ( -12.15795451370000002, -100.5027207520000019, -10.78449129679999885 ) ) ;
#26332=CARTESIAN_POINT ( 'NONE',  ( -0.8253211953949340929, -101.6407018583229132, -15.98448082329617392 ) ) ;
#26337=CARTESIAN_POINT ( 'NONE',  ( -17.54428855099999751, -94.59276292389999696, 16.07755916609999858 ) ) ;
#26340=CARTESIAN_POINT ( 'NONE',  ( -17.39460856262869370, -93.41743724412515348, -21.38387721846088496 ) ) ;
#26342=CARTESIAN_POINT ( 'NONE',  ( 26.00969437890000080, -92.68289734370000588, 10.63460028110000088 ) ) ;
#26350=CARTESIAN_POINT ( 'NONE',  ( -18.90873350840000100, -92.90721294769998906, -21.12364821749999777 ) ) ;
#26352=ORIENTED_EDGE ( 'NONE', *, *, #26367, .F. ) ;
#26353=CARTESIAN_POINT ( 'NONE',  ( -6.045889172941522283, -101.5703832412493171, 14.87708822258295882 ) ) ;
#26354=CARTESIAN_POINT ( 'NONE',  ( 13.78466514429999812, -99.94549701829998867, -9.780229041529999279 ) ) ;
#26355=CARTESIAN_POINT ( 'NONE',  ( -19.64034669340000150, -92.70565393250001307, 20.70273603029999876 ) ) ;
#26358=CARTESIAN_POINT ( 'NONE',  ( 29.83826626095881451, -92.59055325466113118, 6.318856881893660571 ) ) ;
#26359=DIRECTION ( 'NONE',  ( 1.000000000000000000, 0.000000000000000000, 0.000000000000000000 ) ) ;
#26360=ORIENTED_EDGE ( 'NONE', *, *, #6207, .T. ) ;
#26363=CARTESIAN_POINT ( 'NONE',  ( -23.92783087366071015, -92.71346081468063005, -18.91319433822785001 ) ) ;
#26367=EDGE_CURVE ( 'NONE', #3830, #10205, #5801, .T. ) ;
#26372=CARTESIAN_POINT ( 'NONE',  ( 22.63183994989999803, -96.16784750700000473, -4.383698213610000671 ) ) ;
#26377=CARTESIAN_POINT ( 'NONE',  ( 15.54119309900000090, -100.8869817940000075, 1.981729577500000339 ) ) ;
#26381=CARTESIAN_POINT ( 'NONE',  ( -11.27245849040000003, -95.14589738820001230, -21.35309096379999971 ) ) ;
#26383=CARTESIAN_POINT ( 'NONE',  ( -14.42556421679999978, -111.0000000000000000, -2.978755036369999942 ) ) ;
#26388=CARTESIAN_POINT ( 'NONE',  ( 12.90947517493721719, -101.3586211803441159, -9.827147021456303477 ) ) ;
#26391=CARTESIAN_POINT ( 'NONE',  ( -16.14211878319999727, -101.0779259520000011, 3.133147776259999961 ) ) ;
#26392=ORIENTED_EDGE ( 'NONE', *, *, #15467, .F. ) ;
#26394=CARTESIAN_POINT ( 'NONE',  ( -14.44303431870000054, -92.83816993439999976, 26.18160581060000069 ) ) ;
#26397=TOROIDAL_SURFACE ( 'NONE', #6878, 10.00000000000000000, 1.000000000000000000 ) ;
#26399=CARTESIAN_POINT ( 'NONE',  ( 0.3642957135809999913, -101.1412505549999992, -16.16346332520000217 ) ) ;
#26405=ORIENTED_EDGE ( 'NONE', *, *, #16120, .F. ) ;
#26407=CARTESIAN_POINT ( 'NONE',  ( 14.93581056110000027, -101.1848541609999899, 3.234659781990000038 ) ) ;
#26409=CARTESIAN_POINT ( 'NONE',  ( -6.649722661318385519, -98.16872833778059260, 18.49410160609588871 ) ) ;
#26411=CARTESIAN_POINT ( 'NONE',  ( 27.93493094108533015, -92.53708507728566701, 12.24300196966718168 ) ) ;
#26412=CARTESIAN_POINT ( 'NONE',  ( 4.659867367963298257, -92.75430643208848380, -30.14196855148737342 ) ) ;
#26413=CARTESIAN_POINT ( 'NONE',  ( -5.273680924649999824, -107.3487944130000074, -9.653408180790000515 ) ) ;
#26415=CARTESIAN_POINT ( 'NONE',  ( 20.47275178710000176, -93.13207089429998575, 16.42312355550000191 ) ) ;
#26419=CARTESIAN_POINT ( 'NONE',  ( -6.736536556819999966, -101.1716782170000073, 14.21895496870000031 ) ) ;
#26420=ORIENTED_EDGE ( 'NONE', *, *, #28680, .F. ) ;
#26423=CARTESIAN_POINT ( 'NONE',  ( -12.57887770961745844, -100.9364580245582488, -10.76270985140424052 ) ) ;
#26424=ORIENTED_EDGE ( 'NONE', *, *, #26126, .F. ) ;
#26426=CARTESIAN_POINT ( 'NONE',  ( 24.80237488970000115, -93.63284696290000397, -3.743705429929999884 ) ) ;
#26428=CARTESIAN_POINT ( 'NONE',  ( -1.262698870129999928, -100.9763228559999959, -15.63141515150000238 ) ) ;
#26432=CARTESIAN_POINT ( 'NONE',  ( -19.51268635637469373, -92.50000000000000000, -23.44173519759771906 ) ) ;
#26433=AXIS2_PLACEMENT_3D ( 'NONE', #27589, #5562, #25255 ) ;
#26434=ORIENTED_EDGE ( 'NONE', *, *, #4942, .F. ) ;
#26439=CARTESIAN_POINT ( 'NONE',  ( 13.68659840514571613, -100.3041487038156134, -10.18120984587954503 ) ) ;
#26440=CARTESIAN_POINT ( 'NONE',  ( -17.80822692750000158, -101.1889999979999999, -18.25149456069999943 ) ) ;
#26445=CIRCLE ( 'NONE', #14795, 0.4999999999999988343 ) ;
#26452=CARTESIAN_POINT ( 'NONE',  ( -24.74383412450000108, -93.85715850789999593, -2.800417634270000011 ) ) ;
#26456=CARTESIAN_POINT ( 'NONE',  ( 15.98896817450000007, -100.8088109309999965, 4.269801629269999843 ) ) ;
#26470=CARTESIAN_POINT ( 'NONE',  ( -12.17069681629999955, -101.1292389600000092, -9.608835620689999857 ) ) ;
#26483=DIRECTION ( 'NONE',  ( 0.000000000000000000, 1.000000000000000000, 0.000000000000000000 ) ) ;
#26485=EDGE_CURVE ( 'NONE', #18453, #15088, #6615, .T. ) ;
#26488=VERTEX_POINT ( 'NONE', #24241 ) ;
#26489=CARTESIAN_POINT ( 'NONE',  ( 19.94073578940000147, -94.89419905519999077, 14.19046457500000002 ) ) ;
#26491=EDGE_LOOP ( 'NONE', ( #23602, #15696, #7886, #14113 ) ) ;
#26494=AXIS2_PLACEMENT_3D ( 'NONE', #23061, #22618, #3607 ) ;
#26495=CARTESIAN_POINT ( 'NONE',  ( 11.92167937070000150, -101.1848541609999899, -9.561966123969998677 ) ) ;
#26500=CARTESIAN_POINT ( 'NONE',  ( -1.247133441849999969, -101.2306315440000049, -16.16540283980000225 ) ) ;
#26501=CARTESIAN_POINT ( 'NONE',  ( 12.59582948049999906, -101.5964542560000012, -9.931670464719999813 ) ) ;
#26511=CARTESIAN_POINT ( 'NONE',  ( -1.044063374772672637, -92.50630337894764921, -30.48240144424680409 ) ) ;
#26514=CARTESIAN_POINT ( 'NONE',  ( -11.51095449373275237, -94.71798490447446284, -20.64293826046422353 ) ) ;
#26515=FACE_OUTER_BOUND ( 'NONE', #17295, .T. ) ;
#26520=CARTESIAN_POINT ( 'NONE',  ( 23.48647108369999614, -94.80026829410000744, -6.710788097320000034 ) ) ;
#26526=DIRECTION ( 'NONE',  ( 1.000000000000000000, 0.000000000000000000, 0.000000000000000000 ) ) ;
#26528=CARTESIAN_POINT ( 'NONE',  ( -17.00245937369999893, -99.64579666810000447, 3.307441295489999877 ) ) ;
#26529=CARTESIAN_POINT ( 'NONE',  ( -29.52258421500394547, -92.52048598158022230, 7.659457213237817363 ) ) ;
#26532=CARTESIAN_POINT ( 'NONE',  ( 8.712840316590000356, -92.70565333729999224, -27.17408075339999840 ) ) ;
#26539=CARTESIAN_POINT ( 'NONE',  ( -16.91317841180000059, -92.93841875540000785, 21.66141092870000051 ) ) ;
#26546=CARTESIAN_POINT ( 'NONE',  ( 0.2736767326270000411, -101.4829589650000088, -16.12588753389999852 ) ) ;
#26556=CARTESIAN_POINT ( 'NONE',  ( 28.21594761775847715, -92.66777315148628702, 11.58060234458442395 ) ) ;
#26559=CIRCLE ( 'NONE', #60, 16.00000000000000000 ) ;
#26567=CARTESIAN_POINT ( 'NONE',  ( -12.86054043281202830, -100.4507315467552928, -11.02681200338788337 ) ) ;
#26568=ORIENTED_EDGE ( 'NONE', *, *, #20681, .T. ) ;
#26570=CARTESIAN_POINT ( 'NONE',  ( 24.59609816880000110, -94.07620464469999888, -4.012350405089999406 ) ) ;
#26576=CARTESIAN_POINT ( 'NONE',  ( -15.29367271319999766, -101.2995961670000042, 4.428833737689999772 ) ) ;
#26585=VECTOR ( 'NONE', #1238, 1000.000000000000000 ) ;
#26589=EDGE_CURVE ( 'NONE', #23041, #16053, #16816, .T. ) ;
#26595=CARTESIAN_POINT ( 'NONE',  ( -24.11720358960000254, -94.18458606759999441, -3.273744814500000100 ) ) ;
#26600=CARTESIAN_POINT ( 'NONE',  ( -13.46646099420000020, -101.3150700380000018, -9.098099534850002001 ) ) ;
#26601=ORIENTED_EDGE ( 'NONE', *, *, #25050, .T. ) ;
#26603=CARTESIAN_POINT ( 'NONE',  ( 7.748442867550313196, -92.52498922770500656, 29.49944529545556904 ) ) ;
#26605=CARTESIAN_POINT ( 'NONE',  ( 0.4666096705872683770, -99.76647888976904710, -17.31214626689192215 ) ) ;
#26609=CARTESIAN_POINT ( 'NONE',  ( 24.73793100160000336, -93.48569568790000517, -11.30322088119999968 ) ) ;
#26613=CARTESIAN_POINT ( 'NONE',  ( -16.69422297484464934, -98.32621669506406192, 9.018748007586593118 ) ) ;
#26619=CARTESIAN_POINT ( 'NONE',  ( 15.63748056140000209, -111.0000000000000000, 3.386620984279999913 ) ) ;
#26621=ORIENTED_EDGE ( 'NONE', *, *, #12006, .T. ) ;
#26622=AXIS2_PLACEMENT_3D ( 'NONE', #14072, #16099, #9248 ) ;
#26632=ORIENTED_EDGE ( 'NONE', *, *, #12267, .F. ) ;
#26634=DIRECTION ( 'NONE',  ( 0.9723926833689966465, 0.000000000000000000, -0.2333505288839995140 ) ) ;
#26638=ORIENTED_EDGE ( 'NONE', *, *, #27912, .T. ) ;
#26639=CARTESIAN_POINT ( 'NONE',  ( 12.07601763839999975, -101.1284992150000051, -9.565697433850001374 ) ) ;
#26641=CARTESIAN_POINT ( 'NONE',  ( -16.36797140879999901, -92.98481302150000261, -21.06274368449999912 ) ) ;
#26643=DIRECTION ( 'NONE',  ( 0.000000000000000000, -1.000000000000000000, 0.000000000000000000 ) ) ;
#26644=ORIENTED_EDGE ( 'NONE', *, *, #15583, .T. ) ;
#26646=CARTESIAN_POINT ( 'NONE',  ( -5.873418876839999747, -101.3150700380000018, 15.15334698740000086 ) ) ;
#26659=CARTESIAN_POINT ( 'NONE',  ( 8.472249407519999664, -94.22763312370000222, -22.74885336210000020 ) ) ;
#26662=CARTESIAN_POINT ( 'NONE',  ( -14.79537251110000007, -100.9197086940000077, 5.022279785309999411 ) ) ;
#26669=CARTESIAN_POINT ( 'NONE',  ( 23.42164076090000080, -94.71481430550001335, -6.692246347430000242 ) ) ;
#26672=DIRECTION ( 'NONE',  ( 0.3928703629870108349, 0.000000000000000000, -0.9195938657290262386 ) ) ;
#26674=DIRECTION ( 'NONE',  ( 0.000000000000000000, 1.000000000000000000, 0.000000000000000000 ) ) ;
#26676=CARTESIAN_POINT ( 'NONE',  ( -3.067686975420000017, -99.66156977119999283, -17.02465262619999820 ) ) ;
#26678=CARTESIAN_POINT ( 'NONE',  ( 6.462050373635647382, -93.55106866495810891, -26.37547718614715109 ) ) ;
#26679=ADVANCED_FACE ( 'NONE', ( #815 ), #11039, .F. ) ;
#26686=CARTESIAN_POINT ( 'NONE',  ( 10.12141009259999969, -93.14733690340000294, -25.45251484410000131 ) ) ;
#26689=CARTESIAN_POINT ( 'NONE',  ( -13.06507290026208956, -92.68577957609070950, 27.56005317477162109 ) ) ;
#26693=CARTESIAN_POINT ( 'NONE',  ( -15.68860394770000077, -92.62749637799998936, 23.81420858470000113 ) ) ;
#26694=CYLINDRICAL_SURFACE ( 'NONE', #21942, 20.64285714289998808 ) ;
#26698=CARTESIAN_POINT ( 'NONE',  ( 0.4519837481779999666, -101.1191090859999946, -16.29812186430000054 ) ) ;
#26703=DIRECTION ( 'NONE',  ( 0.000000000000000000, 1.000000000000000000, 0.000000000000000000 ) ) ;
#26707=CARTESIAN_POINT ( 'NONE',  ( 28.44011693845432376, -92.82044061124386758, 11.01861317931760453 ) ) ;
#26709=CARTESIAN_POINT ( 'NONE',  ( -5.525815865670000271, -96.93384555590000673, 20.55834025889999950 ) ) ;
#26710=ORIENTED_EDGE ( 'NONE', *, *, #18579, .T. ) ;
#26716=CARTESIAN_POINT ( 'NONE',  ( -7.476488366829999954, -100.9137139110000021, 13.72916197330000010 ) ) ;
#26719=CARTESIAN_POINT ( 'NONE',  ( -12.56815284899212770, -100.9609609850154754, -10.74558065766072268 ) ) ;
#26723=ADVANCED_FACE ( 'NONE', ( #14326 ), #21178, .F. ) ;
#26725=CARTESIAN_POINT ( 'NONE',  ( 8.485272409089999357, -99.18305472260000499, 16.24294048750000030 ) ) ;
#26726=AXIS2_PLACEMENT_3D ( 'NONE', #10671, #19584, #6029 ) ;
#26727=DIRECTION ( 'NONE',  ( 0.000000000000000000, 1.000000000000000000, 0.000000000000000000 ) ) ;
#26728=CARTESIAN_POINT ( 'NONE',  ( -0.7106571652759999802, -98.65110728940000229, -18.63800496320000022 ) ) ;
#26730=CARTESIAN_POINT ( 'NONE',  ( -20.39705533554743866, -92.66777315149587935, -22.67620303909143686 ) ) ;
#26732=CARTESIAN_POINT ( 'NONE',  ( 11.89800671740000126, -101.6095085860000040, -10.74240160559999957 ) ) ;
#26734=CARTESIAN_POINT ( 'NONE',  ( 14.55779679992241071, -95.49497466763517650, 17.32786613936890419 ) ) ;
#26738=DIRECTION ( 'NONE',  ( 0.000000000000000000, 1.000000000000000000, 0.000000000000000000 ) ) ;
#26741=CARTESIAN_POINT ( 'NONE',  ( 24.72994412613420678, -93.38817447845305253, -12.39839833700887972 ) ) ;
#26742=CARTESIAN_POINT ( 'NONE',  ( 27.40661084094997690, -93.08996811606418476, 9.672291729878732980 ) ) ;
#26746=CARTESIAN_POINT ( 'NONE',  ( 8.097647218569999694, -101.1461874760000086, 13.98396581760000146 ) ) ;
#26747=ORIENTED_EDGE ( 'NONE', *, *, #21387, .T. ) ;
#26748=ADVANCED_FACE ( 'NONE', ( #27865 ), #1506, .F. ) ;
#26752=CARTESIAN_POINT ( 'NONE',  ( -24.67188499770000121, -93.87552273910000622, -2.728012672819999818 ) ) ;
#26754=B_SPLINE_CURVE_WITH_KNOTS ( 'NONE', 3,
 ( #3167, #25316, #20651, #18752, #9846, #20938, #5618, #850, #14234, #16555, #18460, #25452, #27344, #5198, #22981, #13736, #61, #22335, #27298, #8908, #6751, #24961, #16059, #11238, #355, #13582, #20593, #7334, #2381, #13431, #17819, #17964, #13877 ),
 .UNSPECIFIED., .F., .F.,
 ( 4, 2, 1, 1, 2, 2, 1, 1, 1, 2, 2, 2, 1, 1, 2, 2, 1, 1, 2, 2, 4 ),
 ( 0.000000000000000000, 0.06250000000008817946, 0.09375000000014409307, 0.1093750000001827011, 0.1171875000001962736, 0.1250000000002098599, 0.1875000000002195744, 0.2187500000002333134, 0.2343750000002418343, 0.2421875000002425005, 0.2500000000002431388, 0.3750000000002057798, 0.4375000000001912359, 0.4687500000001821876, 0.4843750000001772471, 0.5000000000001723066, 0.6250000000001494360, 0.6875000000001377787, 0.7187500000001278977, 0.7500000000001180167, 1.000000000000000000 ),
 .UNSPECIFIED. ) ;
#26757=CARTESIAN_POINT ( 'NONE',  ( 12.02192718879999944, -92.50000321470000131, 27.08489650960000006 ) ) ;
#26762=EDGE_CURVE ( 'NONE', #18376, #842, #5643, .T. ) ;
#26769=CARTESIAN_POINT ( 'NONE',  ( 24.75930092260000137, -93.04780269100000112, -15.39069302210000068 ) ) ;
#26770=DIRECTION ( 'NONE',  ( 1.000000000000000000, 0.000000000000000000, 0.000000000000000000 ) ) ;
#26772=CARTESIAN_POINT ( 'NONE',  ( -17.26556418046517294, -97.08920889912290875, 11.18720961792155499 ) ) ;
#26774=CIRCLE ( 'NONE', #25833, 18.64285714289999873 ) ;
#26776=DIRECTION ( 'NONE',  ( 1.000000000000000000, 0.000000000000000000, 0.000000000000000000 ) ) ;
#26777=CARTESIAN_POINT ( 'NONE',  ( -12.42802429090000160, -100.1785804069999983, -11.07820824309999885 ) ) ;
#26781=CARTESIAN_POINT ( 'NONE',  ( 26.98910893724515958, -92.53708507728568122, -14.20702159799850861 ) ) ;
#26787=CARTESIAN_POINT ( 'NONE',  ( -17.74112986619786625, -94.52292883268154355, 16.06143330243891043 ) ) ;
#26789=VERTEX_POINT ( 'NONE', #24350 ) ;
#26791=CARTESIAN_POINT ( 'NONE',  ( 19.60651196810000130, -94.52293239719999463, 13.72231888900000030 ) ) ;
#26792=CARTESIAN_POINT ( 'NONE',  ( -15.48259164459999937, -101.2306293330000102, 4.813005033020000489 ) ) ;
#26793=EDGE_CURVE ( 'NONE', #27440, #14137, #7525, .T. ) ;
#26796=CARTESIAN_POINT ( 'NONE',  ( -23.48465370626706772, -94.36683344921115690, -7.277453751676699056 ) ) ;
#26797=CARTESIAN_POINT ( 'NONE',  ( 11.77298154309999845, -101.2530993010000060, -9.604785791470000333 ) ) ;
#26801=CARTESIAN_POINT ( 'NONE',  ( 0.000000000000000000, -91.50000000000000000, 0.000000000000000000 ) ) ;
#26802=CARTESIAN_POINT ( 'NONE',  ( 13.96793549529999900, -99.58396362730000817, -10.31305845590000025 ) ) ;
#26805=CARTESIAN_POINT ( 'NONE',  ( -4.781896297090870718, -98.79895878316551716, -18.93514192741941571 ) ) ;
#26807=DIRECTION ( 'NONE',  ( 0.000000000000000000, 1.000000000000000000, 0.000000000000000000 ) ) ;
#26812=CARTESIAN_POINT ( 'NONE',  ( -23.81103214300399173, -92.84927079008255646, -19.06003205102011222 ) ) ;
#26814=CARTESIAN_POINT ( 'NONE',  ( 18.39062685420683252, -98.53908159012071621, 3.638000403930131021 ) ) ;
#26830=CARTESIAN_POINT ( 'NONE',  ( 5.873227382016245279, -93.41743724444744146, -26.93228196801963392 ) ) ;
#26835=CARTESIAN_POINT ( 'NONE',  ( 10.38935269913133830, -95.90275867109022556, -20.92386860843906504 ) ) ;
#26839=CARTESIAN_POINT ( 'NONE',  ( -12.46836486461607940, -92.52640451556476364, 27.83505318500035841 ) ) ;
#26842=CARTESIAN_POINT ( 'NONE',  ( -17.04762123990000333, -93.16621335700000373, 21.75328878690000423 ) ) ;
#26845=CARTESIAN_POINT ( 'NONE',  ( -15.96476880600000037, -99.60585778459999062, 6.856918404960000046 ) ) ;
#26846=CARTESIAN_POINT ( 'NONE',  ( 0.5238881141819999865, -100.0994409990000094, -17.21532606639999941 ) ) ;
#26847=FACE_OUTER_BOUND ( 'NONE', #16902, .T. ) ;
#26853=CARTESIAN_POINT ( 'NONE',  ( 28.41344044897496701, -92.80045754835145999, 11.08727913710079527 ) ) ;
#26855=VERTEX_POINT ( 'NONE', #16178 ) ;
#26861=CARTESIAN_POINT ( 'NONE',  ( -7.039259910420000210, -101.5964542560000012, 14.41325148729999839 ) ) ;
#26869=CARTESIAN_POINT ( 'NONE',  ( -5.417924262829999726, -95.55433883420000996, -21.95361216799999937 ) ) ;
#26870=DIRECTION ( 'NONE',  ( -0.9639181000863472626, 0.000000000000000000, 0.2661989788220960884 ) ) ;
#26874=CARTESIAN_POINT ( 'NONE',  ( 15.48475574042589287, -95.04500097814597837, 17.29312253357641183 ) ) ;
#26875=CARTESIAN_POINT ( 'NONE',  ( 7.181689689069999716, -111.0000000000000000, 15.80535034289999885 ) ) ;
#26876=CIRCLE ( 'NONE', #18027, 18.14285714289999873 ) ;
#26878=DIRECTION ( 'NONE',  ( -0.6983618402939030245, 0.000000000000000000, -0.7157448847329006547 ) ) ;
#26879=CARTESIAN_POINT ( 'NONE',  ( -11.32307664120000013, -101.1889999979999999, 9.421136869679999748 ) ) ;
#26881=CARTESIAN_POINT ( 'NONE',  ( 22.02115912736433145, -94.16483583581477035, 13.38915878678963622 ) ) ;
#26883=CARTESIAN_POINT ( 'NONE',  ( -29.76178938840000043, -93.00000000000000000, 6.669774538800000485 ) ) ;
#26884=ADVANCED_FACE ( 'NONE', ( #27274 ), #11666, .F. ) ;
#26892=CARTESIAN_POINT ( 'NONE',  ( 27.16500929229999883, -92.56290635029999692, 9.195763470240001070 ) ) ;
#26894=CARTESIAN_POINT ( 'NONE',  ( 26.75649127029999619, -101.1889999979999999, -13.26822602009999841 ) ) ;
#26897=CARTESIAN_POINT ( 'NONE',  ( 16.54149060430000162, -99.85455315880000171, 4.477554858519999570 ) ) ;
#26901=CARTESIAN_POINT ( 'NONE',  ( -15.31628404939999832, -99.57131247680000286, -8.300247877169999455 ) ) ;
#26903=CARTESIAN_POINT ( 'NONE',  ( 8.524613012669300716, -92.66455718075849290, 29.28448434949323342 ) ) ;
#26913=CARTESIAN_POINT ( 'NONE',  ( -16.98338203059941520, -97.76568412893885807, 9.980451257739110460 ) ) ;
#26914=ORIENTED_EDGE ( 'NONE', *, *, #28760, .F. ) ;
#26916=CARTESIAN_POINT ( 'NONE',  ( -3.243952255836194176, -98.17436949751105146, 20.08298429705580901 ) ) ;
#26917=CARTESIAN_POINT ( 'NONE',  ( -13.09874939020000006, -100.0482783049999966, -11.14007078999999933 ) ) ;
#26920=ORIENTED_EDGE ( 'NONE', *, *, #28215, .T. ) ;
#26922=ORIENTED_EDGE ( 'NONE', *, *, #18475, .F. ) ;
#26925=FACE_OUTER_BOUND ( 'NONE', #15390, .T. ) ;
#26926=DIRECTION ( 'NONE',  ( 0.000000000000000000, -1.000000000000000000, 0.000000000000000000 ) ) ;
#26927=CARTESIAN_POINT ( 'NONE',  ( 10.52519477159999894, -92.53453854219999641, 27.02797911619999738 ) ) ;
#26932=CARTESIAN_POINT ( 'NONE',  ( -27.56394947256076122, -93.41743724413561267, 0.2670232293074757957 ) ) ;
#26933=CARTESIAN_POINT ( 'NONE',  ( 20.46603143229999944, -94.22485786839999378, 13.79395319179999824 ) ) ;
#26936=CARTESIAN_POINT ( 'NONE',  ( -15.42268960139999834, -111.0000000000000000, 4.259183661149999800 ) ) ;
#26938=CARTESIAN_POINT ( 'NONE',  ( 12.47108311319999885, -101.4121386959999995, -9.987215287249998852 ) ) ;
#26939=CARTESIAN_POINT ( 'NONE',  ( -14.05781381009999897, -93.65023553250000532, -20.95136237079999830 ) ) ;
#26940=CARTESIAN_POINT ( 'NONE',  ( -23.50862727400000196, -94.59276292389999696, -3.692480628369999796 ) ) ;
#26942=CARTESIAN_POINT ( 'NONE',  ( -6.238095109968847751, -101.6484611540000031, 14.73393615897204079 ) ) ;
#26943=B_SPLINE_CURVE_WITH_KNOTS ( 'NONE', 3,
 ( #8462, #17365, #28573, #8608, #26110, #15010, #21594, #1653, #10626, #24057, #3961, #4097, #22030, #23923, #21879, #10771, #25968, #2078 ),
 .UNSPECIFIED., .F., .F.,
 ( 4, 2, 2, 2, 1, 1, 1, 1, 2, 2, 4 ),
 ( 0.000000000000000000, 0.2499999999999300004, 0.3749999999998957501, 0.4374999999998792632, 0.4687499999998714362, 0.4843749999998674949, 0.4921874999998651634, 0.4960937499998637756, 0.4980468749998633871, 0.4999999999998629985, 1.000000000000000000 ),
 .UNSPECIFIED. ) ;
#26944=CARTESIAN_POINT ( 'NONE',  ( -16.98520236649999759, -99.83167676440000093, 3.436659022809999797 ) ) ;
#26948=CARTESIAN_POINT ( 'NONE',  ( 28.66244647610000129, -111.0000000000000000, 10.42660836539999991 ) ) ;
#26950=DIRECTION ( 'NONE',  ( 1.000000000000000000, 0.000000000000000000, 0.000000000000000000 ) ) ;
#26951=CARTESIAN_POINT ( 'NONE',  ( -16.14562817639999892, -101.1889999979999999, 4.458832895280000486 ) ) ;
#26952=DIRECTION ( 'NONE',  ( 0.000000000000000000, 1.000000000000000000, 0.000000000000000000 ) ) ;
#26956=DIRECTION ( 'NONE',  ( 0.000000000000000000, -1.000000000000000000, 0.000000000000000000 ) ) ;
#26958=AXIS2_PLACEMENT_3D ( 'NONE', #10202, #25825, #10611 ) ;
#26961=CARTESIAN_POINT ( 'NONE',  ( -23.82156939022300435, -92.83160374580931773, -19.04685915412109409 ) ) ;
#26964=DIRECTION ( 'NONE',  ( 1.000000000000000000, 0.000000000000000000, 0.000000000000000000 ) ) ;
#26967=CARTESIAN_POINT ( 'NONE',  ( 26.02259374959999860, -91.50000000000000000, -15.90831903569999994 ) ) ;
#26971=VERTEX_POINT ( 'NONE', #19092 ) ;
#26978=CARTESIAN_POINT ( 'NONE',  ( 1.436102896439999999, -94.52419709919999491, 23.97566704719999819 ) ) ;
#26980=CARTESIAN_POINT ( 'NONE',  ( 0.7331063123750001242, -99.53431386179998697, -17.39857302659999760 ) ) ;
#26981=CARTESIAN_POINT ( 'NONE',  ( 11.59887401429227438, -98.07255008377731542, -16.87401357543511438 ) ) ;
#26982=EDGE_LOOP ( 'NONE', ( #3388, #12221, #22790, #16238 ) ) ;
#26985=CARTESIAN_POINT ( 'NONE',  ( -13.34153245340000105, -93.00000000000000000, 27.42724032409999779 ) ) ;
#26986=ORIENTED_EDGE ( 'NONE', *, *, #17771, .F. ) ;
#26992=CARTESIAN_POINT ( 'NONE',  ( -2.986711171310000079, -94.79581646409999962, 23.48470800579999818 ) ) ;
#26993=CARTESIAN_POINT ( 'NONE',  ( 0.6035559297369998966, -99.61736775859999682, -17.33444585840000229 ) ) ;
#26998=EDGE_CURVE ( 'NONE', #5288, #25651, #4723, .T. ) ;
#27001=CARTESIAN_POINT ( 'NONE',  ( 6.916458556970000338, -99.55609327400000552, 15.95096318659999746 ) ) ;
#27004=CARTESIAN_POINT ( 'NONE',  ( -17.54428855099999751, -94.59276292389999696, 16.07755916609999858 ) ) ;
#27005=CARTESIAN_POINT ( 'NONE',  ( 12.52242149219999945, -98.51737542899999767, 15.18253812500000066 ) ) ;
#27007=CARTESIAN_POINT ( 'NONE',  ( 9.015412349990000962, -94.52293239719999463, -22.16843899350000058 ) ) ;
#27010=CARTESIAN_POINT ( 'NONE',  ( -12.46823725472511590, -101.5409490181953487, -10.15889664027061734 ) ) ;
#27015=AXIS2_PLACEMENT_3D ( 'NONE', #16642, #11976, #25535 ) ;
#27016=FACE_OUTER_BOUND ( 'NONE', #4903, .T. ) ;
#27018=CARTESIAN_POINT ( 'NONE',  ( 0.3872225632639999526, -99.92967428129999519, -17.35613189629999908 ) ) ;
#27022=CARTESIAN_POINT ( 'NONE',  ( 15.62957910242984383, -94.97526614585484594, 17.28402939849175013 ) ) ;
#27023=EDGE_CURVE ( 'NONE', #21528, #22228, #11992, .T. ) ;
#27026=CYLINDRICAL_SURFACE ( 'NONE', #10934, 20.64285714290000584 ) ;
#27027=ADVANCED_FACE ( 'NONE', ( #12235 ), #10336, .T. ) ;
#27028=CARTESIAN_POINT ( 'NONE',  ( 24.64042015088250182, -93.08494709825269808, -15.48202326831530407 ) ) ;
#27030=ORIENTED_EDGE ( 'NONE', *, *, #6313, .T. ) ;
#27035=AXIS2_PLACEMENT_3D ( 'NONE', #28087, #23445, #21388 ) ;
#27036=CARTESIAN_POINT ( 'NONE',  ( 21.33283665240000104, -96.53848370399998657, 1.142368493430000020 ) ) ;
#27041=CARTESIAN_POINT ( 'NONE',  ( 16.76297209009999989, -99.69348480060000384, 4.363466760120000565 ) ) ;
#27045=CARTESIAN_POINT ( 'NONE',  ( -21.73574830329999941, -95.72998414210000817, -5.474907084429999848 ) ) ;
#27047=CARTESIAN_POINT ( 'NONE',  ( -30.44581475448487140, -92.66972459461456424, 1.817249682291065538 ) ) ;
#27049=CARTESIAN_POINT ( 'NONE',  ( -5.860725082736318647, -96.53847999719242523, 20.54378296970569906 ) ) ;
#27050=CARTESIAN_POINT ( 'NONE',  ( -11.82347332360000003, -101.2358105800000061, -9.579693020240000578 ) ) ;
#27053=CARTESIAN_POINT ( 'NONE',  ( 23.48645807289999965, -94.80026553589999594, -6.710790866570000013 ) ) ;
#27059=CARTESIAN_POINT ( 'NONE',  ( -17.49077503611597351, -96.32082629555334563, 12.61788199362829488 ) ) ;
#27062=CARTESIAN_POINT ( 'NONE',  ( -4.423592041350528525, -99.33527509803080591, 18.30618831894034670 ) ) ;
#27073=CARTESIAN_POINT ( 'NONE',  ( 2.683228843229999772, -93.81034071199999858, 24.85754899019999797 ) ) ;
#27074=AXIS2_PLACEMENT_3D ( 'NONE', #3013, #18591, #12153 ) ;
#27078=CARTESIAN_POINT ( 'NONE',  ( -11.77049175740000209, -94.59276292389999696, -20.68200892780000189 ) ) ;
#27080=VERTEX_POINT ( 'NONE', #17993 ) ;
#27084=CARTESIAN_POINT ( 'NONE',  ( -11.73664949370000166, -94.54719310899999130, -20.76899502859999913 ) ) ;
#27085=FACE_OUTER_BOUND ( 'NONE', #19908, .T. ) ;
#27089=ADVANCED_FACE ( 'NONE', ( #8071 ), #17591, .F. ) ;
#27090=CARTESIAN_POINT ( 'NONE',  ( -16.97397862119999701, -99.68179698959998802, 2.927883187840000012 ) ) ;
#27094=ORIENTED_EDGE ( 'NONE', *, *, #21643, .F. ) ;
#27097=DIRECTION ( 'NONE',  ( 0.000000000000000000, 1.000000000000000000, 0.000000000000000000 ) ) ;
#27105=CARTESIAN_POINT ( 'NONE',  ( 15.62925250406422428, -101.5740747342780139, 3.683045828202760497 ) ) ;
#27109=B_SPLINE_SURFACE_WITH_KNOTS ( 'NONE', 5, 5, ( 
 ( #10437, #5671, #21399, #28229, #23584, #26051, #6081, #3904, #14957 ),
 ( #21680, #16745, #25642, #5938, #23867, #14551, #16893, #23456, #3495 ),
 ( #21263, #1317, #27963, #5810, #14689, #3628, #1458, #10299, #17024 ),
 ( #25912, #14820, #4631, #8554, #2163, #26342, #137, #4186, #28800 ),
 ( #6368, #17457, #13061, #15235, #13214, #19771, #22122, #15836, #21970 ),
 ( #24447, #24154, #2021, #10860, #2461, #13355, #15541, #28652, #13502 ),
 ( #20074, #2607, #22414, #22259, #4482, #8683, #10999, #4340, #24747 ),
 ( #17894, #2306, #4782, #20219, #26933, #13661, #11315, #6973, #9132 ),
 ( #17601, #26489, #6526, #8986, #290, #11156, #26791, #15385, #18035 ) ),
 .UNSPECIFIED., .F., .F., .F.,
 ( 6, 3, 6 ),
 ( 6, 3, 6 ),
 ( 7.186332008800000004, 18.82033377109999961, 25.08217526889999860 ),
 ( 0.000000000000000000, 0.2500000000000000000, 0.5000000000000000000 ),
 .UNSPECIFIED. ) ;
#27123=CARTESIAN_POINT ( 'NONE',  ( 3.242442617403691330, -93.08384138313282108, -28.92776005519338511 ) ) ;
#27124=CARTESIAN_POINT ( 'NONE',  ( -29.13203926110000097, -92.50000647099999185, 5.968911360329999916 ) ) ;
#27128=CARTESIAN_POINT ( 'NONE',  ( -7.120447010050000358, -111.0000000000000000, 15.21641332169999927 ) ) ;
#27134=DIRECTION ( 'NONE',  ( 0.000000000000000000, 1.000000000000000000, 0.000000000000000000 ) ) ;
#27137=CARTESIAN_POINT ( 'NONE',  ( -18.24993397329999922, -95.76581571470001109, 13.57658235369999922 ) ) ;
#27139=AXIS2_PLACEMENT_3D ( 'NONE', #2196, #9027, #15272 ) ;
#27144=AXIS2_PLACEMENT_3D ( 'NONE', #13136, #14755, #10507 ) ;
#27148=CARTESIAN_POINT ( 'NONE',  ( 28.66244647610000129, -93.00000000000000000, 10.42660836539999991 ) ) ;
#27151=CARTESIAN_POINT ( 'NONE',  ( 12.42071132350000084, -98.30615006589998472, 14.97838199649999957 ) ) ;
#27154=CARTESIAN_POINT ( 'NONE',  ( -11.49546490490405048, -95.15473665344634924, -21.39080332819893471 ) ) ;
#27155=CARTESIAN_POINT ( 'NONE',  ( -20.43932202180000246, -94.59276292389999696, 12.18704577789999988 ) ) ;
#27156=CARTESIAN_POINT ( 'NONE',  ( 6.061325012380000210, -92.50000460620000808, 29.15556959710000129 ) ) ;
#27163=CARTESIAN_POINT ( 'NONE',  ( -0.7163235813839999855, -101.3256027139999986, -15.89054958740000068 ) ) ;
#27165=DIRECTION ( 'NONE',  ( 0.000000000000000000, 1.000000000000000000, 0.000000000000000000 ) ) ;
#27167=CARTESIAN_POINT ( 'NONE',  ( -15.32074598660000042, -101.1659465879999971, 4.659563583299999756 ) ) ;
#27168=CARTESIAN_POINT ( 'NONE',  ( -14.48558484980151206, -100.7167551675964603, -8.980145358784431764 ) ) ;
#27171=CARTESIAN_POINT ( 'NONE',  ( 11.85491415629929968, -101.4218099525233470, -10.99807908417638380 ) ) ;
#27173=CARTESIAN_POINT ( 'NONE',  ( 24.66243531188380089, -93.09721478938284633, -15.27777790653344958 ) ) ;
#27175=ORIENTED_EDGE ( 'NONE', *, *, #22963, .F. ) ;
#27176=DIRECTION ( 'NONE',  ( 0.000000000000000000, 1.000000000000000000, 0.000000000000000000 ) ) ;
#27182=CARTESIAN_POINT ( 'NONE',  ( -18.87095359252083782, -92.56168502752186100, 22.85581819520699653 ) ) ;
#27183=CARTESIAN_POINT ( 'NONE',  ( -18.99756495820000168, -92.50000000000000000, -23.62136188200000220 ) ) ;
#27185=CARTESIAN_POINT ( 'NONE',  ( -14.59383839804472416, -94.00303307107726880, -21.62085948234513211 ) ) ;
#27187=EDGE_CURVE ( 'NONE', #11758, #22088, #4352, .T. ) ;
#27188=CIRCLE ( 'NONE', #28548, 30.50000000000000000 ) ;
#27190=CARTESIAN_POINT ( 'NONE',  ( 16.63506097750000023, -100.0482783049999966, 4.353522604860000200 ) ) ;
#27191=EDGE_LOOP ( 'NONE', ( #11691, #16891, #16744, #1578, #20854, #19015, #18416, #26360, #1648, #12497, #21025, #11959, #649, #23109, #6687, #27823, #19741, #23567, #23954, #9519, #1520, #25, #16391, #19232, #18451, #5524, #23126, #12184 ) ) ;
#27192=CARTESIAN_POINT ( 'NONE',  ( -19.78028125209999999, -96.96081043319999537, -6.989363499150000436 ) ) ;
#27197=FACE_OUTER_BOUND ( 'NONE', #23114, .T. ) ;
#27202=CARTESIAN_POINT ( 'NONE',  ( -3.067686975420000017, -99.66156977119999283, -17.02465262619999820 ) ) ;
#27203=CARTESIAN_POINT ( 'NONE',  ( -17.14077040652199813, -97.41018742068575875, 10.60857521878771870 ) ) ;
#27204=ORIENTED_EDGE ( 'NONE', *, *, #24466, .F. ) ;
#27208=CARTESIAN_POINT ( 'NONE',  ( 7.905782043786379276, -101.5455496411810259, 13.99933444791012072 ) ) ;
#27209=CARTESIAN_POINT ( 'NONE',  ( -5.298192075760000286, -100.9197081840000010, 14.69882727599999939 ) ) ;
#27213=CARTESIAN_POINT ( 'NONE',  ( 26.33530480068390744, -92.82668962668526547, -15.38511375170930862 ) ) ;
#27216=CARTESIAN_POINT ( 'NONE',  ( -0.7975586053140000242, -96.07623048680000011, 23.00905320750000271 ) ) ;
#27217=CARTESIAN_POINT ( 'NONE',  ( 8.056208598280001354, -92.64865434429998459, 26.82756782219999891 ) ) ;
#27219=EDGE_CURVE ( 'NONE', #2458, #10205, #15716, .T. ) ;
#27220=CARTESIAN_POINT ( 'NONE',  ( -4.710490229966223907, -99.82487968069240480, 16.41387846790747673 ) ) ;
#27222=CARTESIAN_POINT ( 'NONE',  ( -24.78124722104226763, -94.60934249595302958, -3.488298834054989861 ) ) ;
#27230=CARTESIAN_POINT ( 'NONE',  ( -4.608126179330000127, -98.80330295420000652, -19.06616812880000111 ) ) ;
#27234=ORIENTED_EDGE ( 'NONE', *, *, #12072, .F. ) ;
#27235=DIRECTION ( 'NONE',  ( 0.000000000000000000, 1.000000000000000000, 0.000000000000000000 ) ) ;
#27247=CARTESIAN_POINT ( 'NONE',  ( 15.83435892164885139, -101.1884902310803795, 4.101762063882318010 ) ) ;
#27248=CARTESIAN_POINT ( 'NONE',  ( -13.32816333360000094, -99.92967571559999840, -11.12411022969999941 ) ) ;
#27256=CARTESIAN_POINT ( 'NONE',  ( 4.685572449352821245, -93.74883191391012360, 26.22100713583913034 ) ) ;
#27257=ORIENTED_EDGE ( 'NONE', *, *, #25673, .F. ) ;
#27258=EDGE_CURVE ( 'NONE', #7956, #9479, #2639, .T. ) ;
#27261=EDGE_LOOP ( 'NONE', ( #7748, #16996, #27994, #17427 ) ) ;
#27262=FACE_OUTER_BOUND ( 'NONE', #3800, .T. ) ;
#27264=EDGE_CURVE ( 'NONE', #14226, #11312, #2336, .T. ) ;
#27267=CARTESIAN_POINT ( 'NONE',  ( 7.202169761539999548, -101.2530994060000040, 13.37848089600000101 ) ) ;
#27274=FACE_OUTER_BOUND ( 'NONE', #92, .T. ) ;
#27281=DIRECTION ( 'NONE',  ( 0.9057388881967942673, 0.000000000000000000, 0.4238361315509041050 ) ) ;
#27283=CARTESIAN_POINT ( 'NONE',  ( -3.134349037060000231, -94.63960343439998724, 23.52861282910000185 ) ) ;
#27286=CARTESIAN_POINT ( 'NONE',  ( -7.893157158527718487, -99.84800943042134236, 15.42810193944218788 ) ) ;
#27290=CARTESIAN_POINT ( 'NONE',  ( 6.888451955769999913, -99.53431386179998697, 15.99365555089999802 ) ) ;
#27296=CARTESIAN_POINT ( 'NONE',  ( 15.04850482649999854, -97.41042756519999557, 15.29532899870000229 ) ) ;
#27298=CARTESIAN_POINT ( 'NONE',  ( 23.63266585800719355, -92.62938374233351624, -19.28077060567576240 ) ) ;
#27300=CARTESIAN_POINT ( 'NONE',  ( -8.034958860690000648, -100.1785804069999983, 14.58156101930000048 ) ) ;
#27301=DIRECTION ( 'NONE',  ( 0.000000000000000000, -1.000000000000000000, 0.000000000000000000 ) ) ;
#27312=CARTESIAN_POINT ( 'NONE',  ( -15.36947541530000017, -101.0685850650000077, 4.769133107380000069 ) ) ;
#27314=CARTESIAN_POINT ( 'NONE',  ( -19.01364933584116557, -98.08323605845289705, -7.561538557556316320 ) ) ;
#27319=CARTESIAN_POINT ( 'NONE',  ( 10.12409544680074269, -100.1470164126797044, 14.62208593278274726 ) ) ;
#27320=DIRECTION ( 'NONE',  ( 0.9839596076661281110, 0.000000000000000000, 0.1783913968820229901 ) ) ;
#27322=CARTESIAN_POINT ( 'NONE',  ( 6.563397635340000313, -101.1700440390000040, 13.82292916689999984 ) ) ;
#27323=CARTESIAN_POINT ( 'NONE',  ( -18.13313556475285537, -92.50000170997873283, -23.79371526278151094 ) ) ;
#27324=CARTESIAN_POINT ( 'NONE',  ( 7.921626121120000086, -101.0233750200000031, 13.74344063909999925 ) ) ;
#27330=CARTESIAN_POINT ( 'NONE',  ( 0.3669127390019999435, -92.63555401869999173, -30.25482938650000264 ) ) ;
#27331=CARTESIAN_POINT ( 'NONE',  ( 16.83483089839999991, -99.92967571559999840, 4.239603441799999928 ) ) ;
#27335=ORIENTED_EDGE ( 'NONE', *, *, #7224, .F. ) ;
#27336=CARTESIAN_POINT ( 'NONE',  ( -30.45665982967346253, -92.62800705134041834, 1.627016164164003964 ) ) ;
#27337=CARTESIAN_POINT ( 'NONE',  ( 0.6132859559569719954, -100.6338045025634784, -16.78345358886858207 ) ) ;
#27340=CARTESIAN_POINT ( 'NONE',  ( 23.54313657600000198, -94.98812477599999227, -6.784142512209999865 ) ) ;
#27344=CARTESIAN_POINT ( 'NONE',  ( 23.77988130051113203, -92.72722989462202747, -19.09888384160796804 ) ) ;
#27345=B_SPLINE_SURFACE_WITH_KNOTS ( 'NONE', 5, 5, ( 
 ( #1677, #21911, #6315, #24088, #5887, #10515, #19714, #1961, #23809 ),
 ( #3989, #28601, #8349, #8632, #14901, #26428, #21762, #6455, #8214 ),
 ( #28045, #16972, #6021, #15322, #24240, #4276, #19430, #13151, #1812 ),
 ( #8082, #26290, #14766, #19574, #4125, #19299, #26142, #3851, #22060 ),
 ( #28314, #2109, #3712, #28181, #17250, #19159, #25861, #12571, #21483 ),
 ( #15040, #1541, #23955, #27163, #20450, #19850, #13593, #20298, #24681 ) ),
 .UNSPECIFIED., .F., .F., .F.,
 ( 6, 6 ),
 ( 6, 3, 6 ),
 ( 4.816191416739999731, 6.255250589890000157 ),
 ( 0.000000000000000000, 0.2500000000000000000, 0.5000000000000000000 ),
 .UNSPECIFIED. ) ;
#27356=ORIENTED_EDGE ( 'NONE', *, *, #18879, .F. ) ;
#27357=EDGE_CURVE ( 'NONE', #20804, #23088, #2409, .T. ) ;
#27362=CARTESIAN_POINT ( 'NONE',  ( 5.750078808689999654, -92.99020741600000406, 26.05463881579999708 ) ) ;
#27364=CARTESIAN_POINT ( 'NONE',  ( 1.631276547419999945, -94.59276292389999696, 23.74086995720000104 ) ) ;
#27365=CARTESIAN_POINT ( 'NONE',  ( -27.66037319239678283, -93.38817447838401620, 0.4406502884517963792 ) ) ;
#27366=CARTESIAN_POINT ( 'NONE',  ( -23.24818410940000035, -92.50000000000000000, -18.83197690249999923 ) ) ;
#27373=CARTESIAN_POINT ( 'NONE',  ( -4.565529784469999797, -98.71594109849999654, -19.04035697939999849 ) ) ;
#27377=DIRECTION ( 'NONE',  ( 0.000000000000000000, 1.000000000000000000, 0.000000000000000000 ) ) ;
#27380=CARTESIAN_POINT ( 'NONE',  ( -15.04954741829999953, -101.1221263650000139, 3.331427410760000374 ) ) ;
#27383=ORIENTED_EDGE ( 'NONE', *, *, #15198, .F. ) ;
#27386=DIRECTION ( 'NONE',  ( 0.9639181000863472626, 0.000000000000000000, -0.2661989788220960884 ) ) ;
#27387=CARTESIAN_POINT ( 'NONE',  ( -7.911401155084729631, -100.0559847774123625, 15.33800364961746787 ) ) ;
#27388=ORIENTED_EDGE ( 'NONE', *, *, #6681, .T. ) ;
#27390=CARTESIAN_POINT ( 'NONE',  ( -10.66313611470000211, -93.32963169590000518, -23.55089348639999969 ) ) ;
#27393=CARTESIAN_POINT ( 'NONE',  ( 16.44482720124391406, -100.3617719035428024, 4.355606921756608685 ) ) ;
#27394=CARTESIAN_POINT ( 'NONE',  ( 13.80549142619667258, -99.84800943040862364, -10.47552699689475908 ) ) ;
#27398=EDGE_CURVE ( 'NONE', #23842, #7500, #11792, .T. ) ;
#27399=CIRCLE ( 'NONE', #18553, 18.14285714289999873 ) ;
#27402=CARTESIAN_POINT ( 'NONE',  ( 3.796526407979370354, -93.99435622736375251, 25.82530452799085552 ) ) ;
#27408=CARTESIAN_POINT ( 'NONE',  ( -6.072822415560001019, -101.2995922080000071, 14.71841970630000063 ) ) ;
#27410=CARTESIAN_POINT ( 'NONE',  ( -18.13877362739999910, -92.50000000000000000, -23.79298866759999598 ) ) ;
#27414=LINE ( 'NONE', #4966, #26017 ) ;
#27415=ORIENTED_EDGE ( 'NONE', *, *, #2168, .T. ) ;
#27417=CARTESIAN_POINT ( 'NONE',  ( 12.82422588410000053, -94.98812656910000385, -19.93894973960000172 ) ) ;
#27418=CARTESIAN_POINT ( 'NONE',  ( 18.32972815309999959, -98.73889367950000917, 3.377607424290000271 ) ) ;
#27420=CARTESIAN_POINT ( 'NONE',  ( 27.24068616960000000, -92.50000000000000000, -13.71841889620000110 ) ) ;
#27421=CARTESIAN_POINT ( 'NONE',  ( 16.52775595720000013, -99.70407914540000149, 4.748034318380000229 ) ) ;
#27429=CARTESIAN_POINT ( 'NONE',  ( -17.74180474119999573, -95.77233259950000388, 13.60688994350000058 ) ) ;
#27434=CYLINDRICAL_SURFACE ( 'NONE', #15426, 5.000000000000000888 ) ;
#27440=VERTEX_POINT ( 'NONE', #6956 ) ;
#27445=CARTESIAN_POINT ( 'NONE',  ( 10.26464537240000041, -99.91548165649999191, 14.76698580470000088 ) ) ;
#27447=FACE_OUTER_BOUND ( 'NONE', #22039, .T. ) ;
#27450=CARTESIAN_POINT ( 'NONE',  ( -7.963319289740001139, -100.1459902240000019, 14.96859886819999907 ) ) ;
#27451=CARTESIAN_POINT ( 'NONE',  ( -9.284696973382905227, -94.23451058009872838, -22.99616710519532248 ) ) ;
#27452=CARTESIAN_POINT ( 'NONE',  ( -22.29269500190000386, -94.98812477769999418, -8.065858985560000249 ) ) ;
#27453=CARTESIAN_POINT ( 'NONE',  ( 7.593737225439999960, -101.4247867140000068, 14.04833072269999938 ) ) ;
#27457=CARTESIAN_POINT ( 'NONE',  ( 11.57623580709999800, -97.32097376039999403, -18.02784085140000414 ) ) ;
#27460=CARTESIAN_POINT ( 'NONE',  ( 11.19714103559999963, -101.2141467319999890, -10.34781371220000068 ) ) ;
#27462=CARTESIAN_POINT ( 'NONE',  ( -17.58052253407977616, -92.66455718075977188, 24.92338817376557714 ) ) ;
#27464=AXIS2_PLACEMENT_3D ( 'NONE', #12461, #2114, #17544 ) ;
#27474=CARTESIAN_POINT ( 'NONE',  ( 6.796301404480000308, -101.1292389600000092, 13.93792919329999869 ) ) ;
#27475=CARTESIAN_POINT ( 'NONE',  ( 14.02725559393949162, -98.99956644197413880, -12.21074518355317728 ) ) ;
#27476=CARTESIAN_POINT ( 'NONE',  ( -11.34613726139999912, -94.73579816560000211, -20.70779685270000314 ) ) ;
#27481=LINE ( 'NONE', #26894, #24107 ) ;
#27486=EDGE_LOOP ( 'NONE', ( #2387, #22249, #24595, #17603 ) ) ;
#27490=CARTESIAN_POINT ( 'NONE',  ( -30.41021540318250871, -92.80045754832352145, 2.338836450776598852 ) ) ;
#27491=CARTESIAN_POINT ( 'NONE',  ( 0.4897868758944445289, -100.0863963177148150, -17.22661518339834075 ) ) ;
#27494=CARTESIAN_POINT ( 'NONE',  ( -11.76437930720000047, -100.8023006570000035, -10.51170590289999929 ) ) ;
#27500=CARTESIAN_POINT ( 'NONE',  ( 13.78600462180000008, -95.55433883439999931, -17.92375705869999791 ) ) ;
#27505=DIRECTION ( 'NONE',  ( 0.000000000000000000, -1.000000000000000000, 0.000000000000000000 ) ) ;
#27508=VECTOR ( 'NONE', #22154, 1000.000000000000000 ) ;
#27513=CARTESIAN_POINT ( 'NONE',  ( 1.338287881580000116, -94.89420189149998919, 24.43791688079999957 ) ) ;
#27514=CARTESIAN_POINT ( 'NONE',  ( 1.563038315939999867, -94.54718900769999834, 23.80456907980000025 ) ) ;
#27516=EDGE_CURVE ( 'NONE', #10282, #19075, #19999, .T. ) ;
#27521=CARTESIAN_POINT ( 'NONE',  ( 0.03460895995285280524, -93.66270333196790432, 25.99333972228773249 ) ) ;
#27526=VECTOR ( 'NONE', #18479, 1000.000000000000000 ) ;
#27534=DIRECTION ( 'NONE',  ( -0.1756244534809639490, 0.000000000000000000, -0.9844572369277969637 ) ) ;
#27535=CARTESIAN_POINT ( 'NONE',  ( -16.50371898579999907, -100.0989745039999832, 2.846197906239999575 ) ) ;
#27539=DIRECTION ( 'NONE',  ( -0.4862861358100839526, 0.000000000000000000, -0.8737996304181506746 ) ) ;
#27546=CARTESIAN_POINT ( 'NONE',  ( 16.42988691214025820, -100.3796496172251693, 4.355994341102395140 ) ) ;
#27547=CARTESIAN_POINT ( 'NONE',  ( 13.81100091409999919, -99.92967571559999840, -10.51865105429999936 ) ) ;
#27550=AXIS2_PLACEMENT_3D ( 'NONE', #10681, #6194, #12869 ) ;
#27555=CARTESIAN_POINT ( 'NONE',  ( 9.576796425482188013, -93.08693841336391017, 27.46382748655467410 ) ) ;
#27562=EDGE_CURVE ( 'NONE', #25484, #22871, #9780, .T. ) ;
#27565=EDGE_CURVE ( 'NONE', #7740, #26971, #22426, .T. ) ;
#27567=AXIS2_PLACEMENT_3D ( 'NONE', #15170, #6305, #17244 ) ;
#27570=CARTESIAN_POINT ( 'NONE',  ( -13.07115940794487052, -101.6174239712916716, -9.267504955542015921 ) ) ;
#27572=CARTESIAN_POINT ( 'NONE',  ( 7.358959778060000012, -101.1389411659999951, 13.51882459459999986 ) ) ;
#27573=VECTOR ( 'NONE', #28536, 1000.000000000000000 ) ;
#27580=ORIENTED_EDGE ( 'NONE', *, *, #1987, .T. ) ;
#27581=CARTESIAN_POINT ( 'NONE',  ( 29.71814534510813033, -92.87422005961060734, 6.861636527948729025 ) ) ;
#27587=DIRECTION ( 'NONE',  ( 0.000000000000000000, -1.000000000000000000, 0.000000000000000000 ) ) ;
#27589=CARTESIAN_POINT ( 'NONE',  ( 0.000000000000000000, 0.000000000000000000, 0.000000000000000000 ) ) ;
#27598=CYLINDRICAL_SURFACE ( 'NONE', #6458, 5.000000000000002665 ) ;
#27599=CARTESIAN_POINT ( 'NONE',  ( -13.46646172799999874, -101.3150705500000157, -9.098097921289998169 ) ) ;
#27601=B_SPLINE_SURFACE_WITH_KNOTS ( 'NONE', 5, 5, ( 
 ( #16482, #1071, #9911, #12368, #25929, #6650, #15662, #17870, #21556 ),
 ( #15513, #16906, #4460, #10449, #3642, #19368, #20047, #26066, #25797 ),
 ( #26769, #8016, #5953, #8279, #6801, #2139, #17725, #8152, #13328 ),
 ( #22233, #6095, #19890, #5825, #14836, #23739, #24564, #2283, #21276 ),
 ( #26609, #1332, #23884, #3782, #24422, #28774, #11130, #10175, #19093 ),
 ( #112, #8962, #27979, #14707, #23598, #12504, #12643, #21415, #1473 ),
 ( #17039, #10314, #19227, #28115, #1611, #28243, #17179, #14972, #3920 ),
 ( #12785, #21693, #22979, #3029, #11882, #848, #16105, #22680, #25005 ),
 ( #22542, #22387, #27053, #20196, #13930, #18311, #15811, #11289, #406 ) ),
 .UNSPECIFIED., .F., .F., .F.,
 ( 6, 3, 6 ),
 ( 6, 3, 6 ),
 ( 7.186332009700000079, 18.82032539240000091, 25.08217527269999891 ),
 ( 0.000000000000000000, 0.2500000000000000000, 0.5000000000000000000 ),
 .UNSPECIFIED. ) ;
#27604=CARTESIAN_POINT ( 'NONE',  ( 7.604558782770000747, -101.6481558220000068, 14.07757856980000000 ) ) ;
#27608=CARTESIAN_POINT ( 'NONE',  ( -9.249130345009998422, -111.0000000000000000, -19.10987009810000004 ) ) ;
#27609=CARTESIAN_POINT ( 'NONE',  ( 11.23915487290000037, -100.8869813350000015, -10.91500521270000057 ) ) ;
#27616=CARTESIAN_POINT ( 'NONE',  ( 14.28941763439999946, -93.00000000000000000, -3.575252188409999921 ) ) ;
#27621=FACE_OUTER_BOUND ( 'NONE', #27191, .T. ) ;
#27623=CARTESIAN_POINT ( 'NONE',  ( 7.102042752109999135, -101.5369810359999860, 14.33739825589999839 ) ) ;
#27626=CARTESIAN_POINT ( 'NONE',  ( -11.16211105210000021, -94.83053003919999924, -21.09958095109999832 ) ) ;
#27630=CARTESIAN_POINT ( 'NONE',  ( 23.58466923419999972, -94.98812477769999418, -2.405350023570000051 ) ) ;
#27632=CARTESIAN_POINT ( 'NONE',  ( -23.49132717730000053, -93.00000000000000000, -19.26887671769999955 ) ) ;
#27637=EDGE_CURVE ( 'NONE', #10282, #1710, #18703, .T. ) ;
#27641=CARTESIAN_POINT ( 'NONE',  ( 6.962669195700001090, -93.00000450890000536, -28.64060852350000275 ) ) ;
#27643=AXIS2_PLACEMENT_3D ( 'NONE', #15774, #20454, #26870 ) ;
#27647=CARTESIAN_POINT ( 'NONE',  ( 0.3872056760429999911, -111.0000000000000000, -17.35614698070000017 ) ) ;
#27648=CARTESIAN_POINT ( 'NONE',  ( 13.49546580460000023, -95.85308664759999431, -18.00277386639999833 ) ) ;
#27662=CARTESIAN_POINT ( 'NONE',  ( -5.121557230439998776, -99.75094652300001030, 17.11281665599999968 ) ) ;
#27663=CARTESIAN_POINT ( 'NONE',  ( -0.7205257401540000606, -101.6484611540000031, -15.98376809950000066 ) ) ;
#27667=CARTESIAN_POINT ( 'NONE',  ( -11.31667057079999950, -95.23931402160000914, -21.36056405359999744 ) ) ;
#27670=VERTEX_POINT ( 'NONE', #10391 ) ;
#27673=CARTESIAN_POINT ( 'NONE',  ( 26.73327912300000264, -92.84292488370000740, -12.41348515490000182 ) ) ;
#27674=CARTESIAN_POINT ( 'NONE',  ( 23.70295537799999863, -94.59276292389999696, -2.111841813949999924 ) ) ;
#27676=ORIENTED_EDGE ( 'NONE', *, *, #20883, .F. ) ;
#27678=CARTESIAN_POINT ( 'NONE',  ( -15.66925473879999764, -101.4673694920000031, 3.460543690009999729 ) ) ;
#27679=CARTESIAN_POINT ( 'NONE',  ( -5.969238273050000210, -101.2530993000000024, 13.97222956270000083 ) ) ;
#27682=DIRECTION ( 'NONE',  ( 0.000000000000000000, 1.000000000000000000, 0.000000000000000000 ) ) ;
#27685=ORIENTED_EDGE ( 'NONE', *, *, #3847, .T. ) ;
#27686=ADVANCED_FACE ( 'NONE', ( #8090 ), #11684, .F. ) ;
#27695=CARTESIAN_POINT ( 'NONE',  ( 6.584707521381107931, -93.38816055823026829, 26.86884258581816454 ) ) ;
#27701=CARTESIAN_POINT ( 'NONE',  ( -5.750261582500000301, -100.9405348700000076, 14.87178911969999895 ) ) ;
#27708=CARTESIAN_POINT ( 'NONE',  ( -29.76178938840000043, -93.00000000000000000, 6.669774538800000485 ) ) ;
#27709=VERTEX_POINT ( 'NONE', #7952 ) ;
#27717=ORIENTED_EDGE ( 'NONE', *, *, #11030, .T. ) ;
#27718=CYLINDRICAL_SURFACE ( 'NONE', #3450, 10.99999999999999822 ) ;
#27724=ADVANCED_FACE ( 'NONE', ( #17409 ), #15184, .T. ) ;
#27731=CARTESIAN_POINT ( 'NONE',  ( 6.962684791734604417, -92.86910576386146943, -28.64059324402698081 ) ) ;
#27737=CARTESIAN_POINT ( 'NONE',  ( 7.584268299279999681, -101.5369811529999993, 14.08825296820000084 ) ) ;
#27741=CARTESIAN_POINT ( 'NONE',  ( 11.43994181019999878, -100.8816831189999874, -10.88980295719999880 ) ) ;
#27748=CARTESIAN_POINT ( 'NONE',  ( 11.86685847370859470, -101.5019029711483682, -10.89638159996464850 ) ) ;
#27750=DIRECTION ( 'NONE',  ( 0.000000000000000000, -1.000000000000000000, 0.000000000000000000 ) ) ;
#27752=ORIENTED_EDGE ( 'NONE', *, *, #7012, .T. ) ;
#27754=CARTESIAN_POINT ( 'NONE',  ( 7.102042752109999135, -101.6484611540000031, 14.33739825589999839 ) ) ;
#27755=CARTESIAN_POINT ( 'NONE',  ( -4.556355293060001005E-12, -111.0000000000000000, 3.907985046680000915E-12 ) ) ;
#27756=CARTESIAN_POINT ( 'NONE',  ( 7.629218925470000023, -101.5342894280000081, 14.06592359269999903 ) ) ;
#27758=ADVANCED_FACE ( 'NONE', ( #83 ), #22886, .F. ) ;
#27759=CARTESIAN_POINT ( 'NONE',  ( -11.21692420940000012, -94.79902974079999467, -20.68495762359999901 ) ) ;
#27761=DIRECTION ( 'NONE',  ( -0.2287893768880245315, 0.000000000000000000, 0.9734759478401042720 ) ) ;
#27762=CARTESIAN_POINT ( 'NONE',  ( 0.000000000000000000, -92.50000000000000000, 0.000000000000000000 ) ) ;
#27770=CARTESIAN_POINT ( 'NONE',  ( 0.5962742269612683055, -100.4103893717004325, -16.96241722493727622 ) ) ;
#27772=CARTESIAN_POINT ( 'NONE',  ( 13.19836993693740901, -92.83160374581309782, 27.49641872786132168 ) ) ;
#27773=CARTESIAN_POINT ( 'NONE',  ( -13.26856174610000139, -93.91547326100000248, -20.89962974999999901 ) ) ;
#27788=CARTESIAN_POINT ( 'NONE',  ( -0.7116806507476617361, -101.2404586421512960, -15.78755322732534516 ) ) ;
#27792=EDGE_LOOP ( 'NONE', ( #12490, #12293, #9196, #19602, #4255, #18668 ) ) ;
#27795=CARTESIAN_POINT ( 'NONE',  ( 25.51708727519999798, -93.49005502320000005, -5.885575441059999413 ) ) ;
#27800=CARTESIAN_POINT ( 'NONE',  ( -16.61164113330000092, -100.3817456209999932, 3.144183042669999928 ) ) ;
#27808=ADVANCED_FACE ( 'NONE', ( #13163 ), #13010, .T. ) ;
#27814=VERTEX_POINT ( 'NONE', #22513 ) ;
#27815=PRODUCT_DEFINITION_CONTEXT ( 'detailed design', #23920, 'design' ) ;
#27818=CARTESIAN_POINT ( 'NONE',  ( 7.111342659921327858, -99.99762666413238321, 15.77675795231586697 ) ) ;
#27820=ORIENTED_EDGE ( 'NONE', *, *, #7639, .F. ) ;
#27822=CARTESIAN_POINT ( 'NONE',  ( -18.26355152109625379, -98.33636770627157375, 5.096710379585314143 ) ) ;
#27823=ORIENTED_EDGE ( 'NONE', *, *, #21286, .T. ) ;
#27824=DIRECTION ( 'NONE',  ( 0.4794255386042041156, 0.000000000000000000, 0.8775825618903722036 ) ) ;
#27825=CARTESIAN_POINT ( 'NONE',  ( -6.273729852859999845, -101.4254868729999970, 14.68495471219999970 ) ) ;
#27827=CARTESIAN_POINT ( 'NONE',  ( -3.253648539801173634, -97.41291607254315466, -20.33721584584428399 ) ) ;
#27829=CIRCLE ( 'NONE', #13871, 7.000000000000000000 ) ;
#27831=CARTESIAN_POINT ( 'NONE',  ( -13.17202554217881172, -101.5620304352245000, -9.196801823362664052 ) ) ;
#27837=CARTESIAN_POINT ( 'NONE',  ( 14.84965784370000108, -101.2530993010000060, 3.216001622850000352 ) ) ;
#27849=ORIENTED_EDGE ( 'NONE', *, *, #6763, .F. ) ;
#27852=CARTESIAN_POINT ( 'NONE',  ( -13.08859102019999909, -101.0314399550000104, -8.948266247160001186 ) ) ;
#27857=CARTESIAN_POINT ( 'NONE',  ( -7.700314492880000472, -100.7430069139999915, 14.58460939829999958 ) ) ;
#27859=CARTESIAN_POINT ( 'NONE',  ( 3.969098514279999712, -92.85282594270000800, 28.21540908839999773 ) ) ;
#27861=CARTESIAN_POINT ( 'NONE',  ( 7.611014957459999231, -101.5361728780000021, 14.07441484610000160 ) ) ;
#27865=FACE_OUTER_BOUND ( 'NONE', #25846, .T. ) ;
#27866=FACE_OUTER_BOUND ( 'NONE', #632, .T. ) ;
#27871=CARTESIAN_POINT ( 'NONE',  ( -18.27190991239999818, -94.89419557770000324, 16.28310526140000292 ) ) ;
#27875=CARTESIAN_POINT ( 'NONE',  ( -0.1711623186869999924, -101.1411470200000053, -15.38827638959999966 ) ) ;
#27877=CARTESIAN_POINT ( 'NONE',  ( 15.82520484449999998, -101.1659666750000071, 2.449319158209999792 ) ) ;
#27883=CARTESIAN_POINT ( 'NONE',  ( 6.651374809830000068, -101.0640712160000021, 14.66145036780000055 ) ) ;
#27886=CARTESIAN_POINT ( 'NONE',  ( -11.80897046999999844, -94.89420189129998562, -21.43714095509999851 ) ) ;
#27887=CARTESIAN_POINT ( 'NONE',  ( -0.7205257401540000606, -101.6484611540000031, -15.98376809950000066 ) ) ;
#27888=CARTESIAN_POINT ( 'NONE',  ( 6.867289776849999861, -92.50000000000000000, 29.52484619129999643 ) ) ;
#27896=CARTESIAN_POINT ( 'NONE',  ( 0.000000000000000000, -94.59276292389999696, 0.000000000000000000 ) ) ;
#27899=EDGE_CURVE ( 'NONE', #28309, #23896, #2619, .T. ) ;
#27905=CARTESIAN_POINT ( 'NONE',  ( 0.3082441019822620976, -101.4241070620154233, -16.17049741965218956 ) ) ;
#27906=CARTESIAN_POINT ( 'NONE',  ( 6.592724576960000249, -99.70407914540000149, 15.88227091829999971 ) ) ;
#27907=CARTESIAN_POINT ( 'NONE',  ( 13.35210321545571333, -92.71346081467784472, 27.42209601977759093 ) ) ;
#27909=CARTESIAN_POINT ( 'NONE',  ( 7.584268328590000330, -111.0000000000000000, 14.08825304710000026 ) ) ;
#27912=EDGE_CURVE ( 'NONE', #24436, #14792, #8699, .T. ) ;
#27914=B_SPLINE_CURVE_WITH_KNOTS ( 'NONE', 3,
 ( #20890, #27154, #805, #14183 ),
 .UNSPECIFIED., .F., .F.,
 ( 4, 4 ),
 ( 0.000000000000000000, 1.000000000000000000 ),
 .UNSPECIFIED. ) ;
#27915=CARTESIAN_POINT ( 'NONE',  ( -14.64568814080000081, -101.2530993010000060, 4.044604232330000215 ) ) ;
#27921=EDGE_LOOP ( 'NONE', ( #13812, #24347, #14530, #4921, #17618, #14986 ) ) ;
#27925=CARTESIAN_POINT ( 'NONE',  ( -27.96632252730000090, -92.66001714109999909, 1.737774121780000014 ) ) ;
#27933=CARTESIAN_POINT ( 'NONE',  ( -29.76178938840000043, -111.0000000000000000, 6.669774538800000485 ) ) ;
#27937=ORIENTED_EDGE ( 'NONE', *, *, #25132, .F. ) ;
#27942=CARTESIAN_POINT ( 'NONE',  ( -16.17838246639999866, -100.4713644509999995, 2.927895792630000216 ) ) ;
#27944=CARTESIAN_POINT ( 'NONE',  ( -5.998097866333861994, -101.1962283502516158, 14.03978137420685890 ) ) ;
#27946=CARTESIAN_POINT ( 'NONE',  ( 20.36577900666061325, -98.12113811797581775, -1.382477163405677389 ) ) ;
#27948=CARTESIAN_POINT ( 'NONE',  ( -7.717204813168451416, -100.8945630372283517, 14.68338577015975233 ) ) ;
#27949=ORIENTED_EDGE ( 'NONE', *, *, #19452, .F. ) ;
#27955=CARTESIAN_POINT ( 'NONE',  ( 6.656876267563871963, -101.0147714271303698, 15.09013656268733072 ) ) ;
#27957=DIRECTION ( 'NONE',  ( -0.3790931394101558771, -0.6121731929912518355, -0.6939253370752848094 ) ) ;
#27962=EDGE_LOOP ( 'NONE', ( #15428, #21089, #8887, #18981 ) ) ;
#27963=CARTESIAN_POINT ( 'NONE',  ( 27.45142615009999787, -92.87863191399999607, 9.755964952359999387 ) ) ;
#27964=CARTESIAN_POINT ( 'NONE',  ( -5.298188773579999733, -100.9197086960000007, 14.69882804600000092 ) ) ;
#27967=DIRECTION ( 'NONE',  ( 0.000000000000000000, 1.000000000000000000, 0.000000000000000000 ) ) ;
#27969=EDGE_CURVE ( 'NONE', #8453, #25457, #9640, .T. ) ;
#27976=CARTESIAN_POINT ( 'NONE',  ( -13.22728828230000175, -99.73367660430000115, -11.16491717010000073 ) ) ;
#27979=CARTESIAN_POINT ( 'NONE',  ( 24.22375112459999968, -93.90388142510001046, -8.961400531120000679 ) ) ;
#27980=ORIENTED_EDGE ( 'NONE', *, *, #12172, .F. ) ;
#27984=CONICAL_SURFACE ( 'NONE', #2875, 13.13304743849999667, 0.9119902906770002149 ) ;
#27992=B_SPLINE_SURFACE_WITH_KNOTS ( 'NONE', 5, 5, ( 
 ( #27599, #5296, #7770, #11973, #25533, #14316, #5572, #14456, #12257 ),
 ( #23349, #3393, #25680, #18974, #27852, #1764, #3662, #21715, #16926 ),
 ( #1634, #3941, #16782, #8445, #24040, #10198, #4078, #7904, #10603 ),
 ( #25819, #28138, #17347, #12806, #5705, #8298, #26240, #12946, #21299 ),
 ( #12526, #14589, #12665, #10063, #21437, #5974, #3805, #21577, #14993 ),
 ( #14725, #21859, #23491, #8172, #17202, #1496, #19114, #1350, #3530 ) ),
 .UNSPECIFIED., .F., .F., .F.,
 ( 6, 6 ),
 ( 6, 3, 6 ),
 ( 4.816191416729999730, 6.255250589890000157 ),
 ( 0.000000000000000000, 0.2500000000000000000, 0.5000000000000000000 ),
 .UNSPECIFIED. ) ;
#27994=ORIENTED_EDGE ( 'NONE', *, *, #19369, .T. ) ;
#27997=CARTESIAN_POINT ( 'NONE',  ( -25.37284092810000047, -111.0000000000000000, 2.543411731580000001 ) ) ;
#27999=ORIENTED_EDGE ( 'NONE', *, *, #19311, .F. ) ;
#28001=CARTESIAN_POINT ( 'NONE',  ( 9.165534020729998232, -98.33329995120000433, 16.60371393490000003 ) ) ;
#28005=CARTESIAN_POINT ( 'NONE',  ( -8.176071803510000180, -99.94549701829998867, 14.79262394269999881 ) ) ;
#28006=CARTESIAN_POINT ( 'NONE',  ( -1.526193099469999925, -100.8869807189999932, -15.59252015110000045 ) ) ;
#28007=CARTESIAN_POINT ( 'NONE',  ( 11.86655840719999944, -101.3150700380000018, -11.10431293650000129 ) ) ;
#28009=ORIENTED_EDGE ( 'NONE', *, *, #23307, .T. ) ;
#28010=CARTESIAN_POINT ( 'NONE',  ( 13.05506823074590450, -101.2145573445107232, -9.820936334222084341 ) ) ;
#28018=CARTESIAN_POINT ( 'NONE',  ( -18.16554934440000224, -94.32610680340000897, 17.27505836280000295 ) ) ;
#28019=CARTESIAN_POINT ( 'NONE',  ( -17.56889148192910355, -92.66777315148752336, 24.93158845175500460 ) ) ;
#28022=FACE_OUTER_BOUND ( 'NONE', #12744, .T. ) ;
#28023=CARTESIAN_POINT ( 'NONE',  ( 27.10195004252156892, -92.50000267095391848, -12.39581383284575722 ) ) ;
#28024=CARTESIAN_POINT ( 'NONE',  ( 15.19718069640000024, -101.1364147039999892, 2.131293228500000581 ) ) ;
#28030=CARTESIAN_POINT ( 'NONE',  ( 6.750186163829999586, -101.4829589650000088, 14.64766651940000131 ) ) ;
#28031=CARTESIAN_POINT ( 'NONE',  ( 15.53854631970000000, -101.2063419769999939, 3.759158181819999722 ) ) ;
#28032=CARTESIAN_POINT ( 'NONE',  ( -11.51095922780000080, -94.71799100319999809, -20.64292660030000093 ) ) ;
#28033=CARTESIAN_POINT ( 'NONE',  ( 4.438282752932665609, -92.81370807104723042, -30.17535407529405589 ) ) ;
#28035=CARTESIAN_POINT ( 'NONE',  ( -6.544663280410000006, -97.83383802230000015, 18.86537983400000229 ) ) ;
#28036=CARTESIAN_POINT ( 'NONE',  ( 1.723886190540000030, -92.49999926799999628, -29.27157131740000295 ) ) ;
#28038=AXIS2_PLACEMENT_3D ( 'NONE', #13181, #8525, #17426 ) ;
#28042=CARTESIAN_POINT ( 'NONE',  ( -5.390284282690000595, -100.8869817940000075, 14.71056662440000018 ) ) ;
#28045=CARTESIAN_POINT ( 'NONE',  ( -1.099649763710000006, -101.5317765570000006, -16.05045154129999929 ) ) ;
#28048=CARTESIAN_POINT ( 'NONE',  ( 15.11157726140000079, -100.8815367389999977, 4.163621051679999852 ) ) ;
#28054=CARTESIAN_POINT ( 'NONE',  ( 24.04216374601140771, -94.35876167748494936, -8.283021781734792199 ) ) ;
#28059=EDGE_LOOP ( 'NONE', ( #7927, #5409, #14943, #1694, #27820, #3962, #10641 ) ) ;
#28064=ADVANCED_FACE ( 'NONE', ( #28022 ), #10561, .T. ) ;
#28065=DIRECTION ( 'NONE',  ( 0.7436828042389473925, 0.000000000000000000, -0.6685326369589560391 ) ) ;
#28070=CARTESIAN_POINT ( 'NONE',  ( -17.92889229695188291, -97.41291607277516107, -10.13624181689873716 ) ) ;
#28076=CARTESIAN_POINT ( 'NONE',  ( -7.333297298759998917, -94.59276292389999696, -22.63874378639999563 ) ) ;
#28078=CARTESIAN_POINT ( 'NONE',  ( -16.78472755060580113, -98.73470581871430340, -7.771690127070184140 ) ) ;
#28082=CARTESIAN_POINT ( 'NONE',  ( -12.52932295349999947, -101.5216621940000152, -9.967556391629999624 ) ) ;
#28084=DIRECTION ( 'NONE',  ( -0.000000000000000000, 1.000000000000000000, 0.000000000000000000 ) ) ;
#28087=CARTESIAN_POINT ( 'NONE',  ( 11.70455088819999823, -101.1889999979999999, 8.942783294160001617 ) ) ;
#28092=CARTESIAN_POINT ( 'NONE',  ( 6.662036864477173026, -100.9510322837155627, 15.14271383432438789 ) ) ;
#28095=ADVANCED_FACE ( 'NONE', ( #25521 ), #13347, .F. ) ;
#28096=ORIENTED_EDGE ( 'NONE', *, *, #23951, .F. ) ;
#28100=DIRECTION ( 'NONE',  ( 1.000000000000000000, 0.000000000000000000, 0.000000000000000000 ) ) ;
#28102=ORIENTED_EDGE ( 'NONE', *, *, #9646, .T. ) ;
#28106=AXIS2_PLACEMENT_3D ( 'NONE', #14233, #13932, #14369 ) ;
#28107=DIRECTION ( 'NONE',  ( 1.000000000000000000, 0.000000000000000000, 0.000000000000000000 ) ) ;
#28113=CARTESIAN_POINT ( 'NONE',  ( 13.27522782530000001, -100.4731125450000064, -9.288511226849999858 ) ) ;
#28114=FACE_OUTER_BOUND ( 'NONE', #23555, .T. ) ;
#28115=CARTESIAN_POINT ( 'NONE',  ( 23.95450574879999905, -94.06807348049999007, -8.162316271139999913 ) ) ;
#28116=EDGE_LOOP ( 'NONE', ( #1157, #24071, #19386, #2917 ) ) ;
#28118=CARTESIAN_POINT ( 'NONE',  ( 14.19394421396252071, -96.53847999818489711, -15.96643556996691515 ) ) ;
#28122=CARTESIAN_POINT ( 'NONE',  ( -18.59081129359999807, -92.50000000000000000, 24.17915911369999904 ) ) ;
#28126=ADVANCED_FACE ( 'NONE', ( #19234 ), #16635, .F. ) ;
#28127=B_SPLINE_CURVE_WITH_KNOTS ( 'NONE', 5,
 ( #10247, #19301, #14640, #14903, #21215, #12717 ),
 .UNSPECIFIED., .F., .F.,
 ( 6, 6 ),
 ( 0.000000000000000000, 1.000000000000000000 ),
 .UNSPECIFIED. ) ;
#28130=B_SPLINE_CURVE_WITH_KNOTS ( 'NONE', 5,
 ( #22415, #26792, #1873, #24006, #13215, #13503, #22123, #28520, #2462 ),
 .UNSPECIFIED., .F., .F.,
 ( 6, 3, 6 ),
 ( 0.000000000000000000, 0.5000000000000000000, 1.000000000000000000 ),
 .UNSPECIFIED. ) ;
#28138=CARTESIAN_POINT ( 'NONE',  ( -13.09607815989999935, -101.5026188610000020, -9.231260805549998949 ) ) ;
#28142=CARTESIAN_POINT ( 'NONE',  ( -1.589809170069999888, -93.96464232220000667, 24.84966672209999672 ) ) ;
#28147=CARTESIAN_POINT ( 'NONE',  ( -28.39119738240000146, -92.85282594270000800, -2.408934254250000073 ) ) ;
#28148=CARTESIAN_POINT ( 'NONE',  ( -15.55828293390000105, -101.6484611540000031, 3.733608462140000306 ) ) ;
#28150=AXIS2_PLACEMENT_3D ( 'NONE', #12687, #8058, #21597 ) ;
#28151=CARTESIAN_POINT ( 'NONE',  ( -8.852567479250000204, -98.72068567929999006, -16.20451607640000091 ) ) ;
#28154=CARTESIAN_POINT ( 'NONE',  ( -18.05296197570000061, -94.57749224630001095, 16.11416072500000141 ) ) ;
#28159=CARTESIAN_POINT ( 'NONE',  ( 0.05945881221699999414, -101.4908759489999994, -16.03087095909999960 ) ) ;
#28167=CARTESIAN_POINT ( 'NONE',  ( 6.497518321730000324, -100.8455998110000138, 14.66870431030000077 ) ) ;
#28168=CARTESIAN_POINT ( 'NONE',  ( 15.35292075490000130, -101.1617736559999940, 3.478357854820000039 ) ) ;
#28171=LINE ( 'NONE', #25984, #3200 ) ;
#28173=CARTESIAN_POINT ( 'NONE',  ( 0.2582735113180000264, -92.50000947299999154, -29.99035778690000242 ) ) ;
#28175=CARTESIAN_POINT ( 'NONE',  ( -0.6842253573819999657, -101.2530993000000024, -15.17849927279999989 ) ) ;
#28181=CARTESIAN_POINT ( 'NONE',  ( -0.8151688476029999020, -101.3256027080000052, -15.88609378809999839 ) ) ;
#28185=CARTESIAN_POINT ( 'NONE',  ( 13.63898564678551217, -92.59735406129850332, 27.28055442926964247 ) ) ;
#28188=FACE_OUTER_BOUND ( 'NONE', #9936, .T. ) ;
#28200=CARTESIAN_POINT ( 'NONE',  ( 15.21476480610000159, -100.7776802639999971, 4.291817874450000403 ) ) ;
#28201=ORIENTED_EDGE ( 'NONE', *, *, #2488, .T. ) ;
#28211=B_SPLINE_SURFACE_WITH_KNOTS ( 'NONE', 5, 5, ( 
 ( #20781, #2859, #690, #18444, #27330, #9678, #18589, #28173, #21336 ),
 ( #21473, #10646, #3838, #28449, #6156, #19560, #21751, #8484, #28036 ),
 ( #1950, #17386, #15167, #25853, #8206, #1528, #10374, #28302, #8621 ),
 ( #26280, #15028, #12703, #10791, #6301, #24077, #23941, #21618, #4116 ),
 ( #12988, #16965, #8076, #3980, #1803, #14892, #19289, #21897, #19706 ),
 ( #14627, #19149, #28592, #8335, #17238, #17527, #26132, #5745, #5876 ),
 ( #23527, #14754, #3563, #17094, #12839, #12418, #25986, #10506, #1391 ),
 ( #6012, #10235, #1669, #23658, #19420, #3701, #12561, #23803, #22050 ),
 ( #9202, #13135, #6445, #15310, #18115, #19991, #27007, #4414, #4264 ) ),
 .UNSPECIFIED., .F., .F., .F.,
 ( 6, 3, 6 ),
 ( 6, 3, 6 ),
 ( 7.186332009330000048, 18.82032539060000076, 25.08217526979999690 ),
 ( 0.000000000000000000, 0.2500000000000000000, 0.5000000000000000000 ),
 .UNSPECIFIED. ) ;
#28214=CARTESIAN_POINT ( 'NONE',  ( -12.20497308240000045, -100.9364576079999978, -10.26977901770000123 ) ) ;
#28215=EDGE_CURVE ( 'NONE', #13014, #23896, #12245, .T. ) ;
#28216=CARTESIAN_POINT ( 'NONE',  ( 22.87124123144904075, -93.20709273738651746, 15.22480860173989292 ) ) ;
#28217=CARTESIAN_POINT ( 'NONE',  ( -7.050140110103686908, -101.5829753080988951, 14.41921209752971933 ) ) ;
#28221=CARTESIAN_POINT ( 'NONE',  ( 16.41935458950000282, -101.1889999979999999, 3.555952033500000109 ) ) ;
#28226=DIRECTION ( 'NONE',  ( 1.000000000000000000, 0.000000000000000000, 0.000000000000000000 ) ) ;
#28229=CARTESIAN_POINT ( 'NONE',  ( 29.48758676550000146, -92.76843000840000286, 7.141489252159999523 ) ) ;
#28232=CARTESIAN_POINT ( 'NONE',  ( -2.033096837813636260, -98.16872835121394303, -19.54781630589999963 ) ) ;
#28234=CARTESIAN_POINT ( 'NONE',  ( -29.51923111000500199, -92.73901256242717750, -0.4406596607846700042 ) ) ;
#28235=CARTESIAN_POINT ( 'NONE',  ( -23.24818218629999933, -92.50000942380000879, -18.83198054589999870 ) ) ;
#28238=EDGE_LOOP ( 'NONE', ( #25152, #6893, #13097, #19445, #15979 ) ) ;
#28239=EDGE_CURVE ( 'NONE', #27670, #25484, #26876, .T. ) ;
#28241=CARTESIAN_POINT ( 'NONE',  ( 13.69115815750000031, -100.1275643909999928, -9.470476298019999462 ) ) ;
#28242=CARTESIAN_POINT ( 'NONE',  ( -18.87095359170000108, -92.56168502750000471, 22.85581819720000141 ) ) ;
#28243=CARTESIAN_POINT ( 'NONE',  ( 23.60984797820000125, -93.86380869110000447, -8.186449766750000023 ) ) ;
#28246=CARTESIAN_POINT ( 'NONE',  ( 29.87796749985422551, -92.54938211466324560, 6.129015425175801113 ) ) ;
#28248=ORIENTED_EDGE ( 'NONE', *, *, #4237, .T. ) ;
#28252=FACE_OUTER_BOUND ( 'NONE', #6810, .T. ) ;
#28260=ORIENTED_EDGE ( 'NONE', *, *, #16687, .F. ) ;
#28264=VERTEX_POINT ( 'NONE', #28122 ) ;
#28265=CARTESIAN_POINT ( 'NONE',  ( 9.220169834260000030, -98.40144667389999711, 16.53004056780000042 ) ) ;
#28268=CARTESIAN_POINT ( 'NONE',  ( -2.813068680090000218, -100.0569316250000043, -17.72190955770000187 ) ) ;
#28275=CARTESIAN_POINT ( 'NONE',  ( 13.28061171819887498, -100.9510322836353566, -9.864576516243763749 ) ) ;
#28276=DIRECTION ( 'NONE',  ( 1.000000000000000000, 0.000000000000000000, 0.000000000000000000 ) ) ;
#28278=CARTESIAN_POINT ( 'NONE',  ( 10.08117464879999936, -95.77248565549999171, -19.95701232960000127 ) ) ;
#28294=CARTESIAN_POINT ( 'NONE',  ( 6.684844807969999358, -101.1412505549999992, 14.72083923979999831 ) ) ;
#28295=CARTESIAN_POINT ( 'NONE',  ( 15.35098429600000003, -101.1417990620000040, 3.558396942789999962 ) ) ;
#28300=CARTESIAN_POINT ( 'NONE',  ( -5.767817971120000387, -96.58372172840000758, 20.50849305530000066 ) ) ;
#28302=CARTESIAN_POINT ( 'NONE',  ( 3.175154110669999863, -92.54030566109999256, -28.53399386439999930 ) ) ;
#28304=CARTESIAN_POINT ( 'NONE',  ( 6.730370301866488880, -101.4085864805377355, 14.71977399093492522 ) ) ;
#28305=CARTESIAN_POINT ( 'NONE',  ( -6.781378104809999030, -101.5369810359999860, 14.49182221120000058 ) ) ;
#28308=CARTESIAN_POINT ( 'NONE',  ( -12.64133138332632811, -100.8061861236792112, -10.84778541818321607 ) ) ;
#28309=VERTEX_POINT ( 'NONE', #12929 ) ;
#28310=CARTESIAN_POINT ( 'NONE',  ( 26.78516883749999877, -92.58502644580001117, -10.10571434189999884 ) ) ;
#28313=EDGE_CURVE ( 'NONE', #6421, #10170, #2246, .T. ) ;
#28314=CARTESIAN_POINT ( 'NONE',  ( -0.8498591013580000242, -101.6484611580000035, -15.97793793410000340 ) ) ;
#28318=DIRECTION ( 'NONE',  ( 0.000000000000000000, -1.000000000000000000, 0.000000000000000000 ) ) ;
#28321=TOROIDAL_SURFACE ( 'NONE', #22775, 21.14285714289999873, 0.5000000000000000000 ) ;
#28326=CARTESIAN_POINT ( 'NONE',  ( 24.73953371475964147, -92.49999918154817635, 14.89633460343937799 ) ) ;
#28327=CARTESIAN_POINT ( 'NONE',  ( 7.939780906490000234, -101.1889999979999999, 14.74863990870000130 ) ) ;
#28334=ADVANCED_FACE ( 'NONE', ( #1896 ), #10883, .F. ) ;
#28336=AXIS2_PLACEMENT_3D ( 'NONE', #26109, #3820, #16945 ) ;
#28337=DIRECTION ( 'NONE',  ( 0.000000000000000000, 1.000000000000000000, 0.000000000000000000 ) ) ;
#28345=CARTESIAN_POINT ( 'NONE',  ( 7.102042752109999135, -101.1889999979999999, 14.33739825589999839 ) ) ;
#28355=CARTESIAN_POINT ( 'NONE',  ( -11.98370860700000051, -101.2530993010000060, -9.340542411159999503 ) ) ;
#28356=CARTESIAN_POINT ( 'NONE',  ( -7.898777529207614556, -100.4010812938397521, 15.03135312487839137 ) ) ;
#28357=ORIENTED_EDGE ( 'NONE', *, *, #24293, .T. ) ;
#28358=CIRCLE ( 'NONE', #2793, 0.5000000000000008882 ) ;
#28365=CARTESIAN_POINT ( 'NONE',  ( 6.982153158335030696, -100.1517898586307496, 15.69801493785662849 ) ) ;
#28368=CARTESIAN_POINT ( 'NONE',  ( -29.47186832370000076, -93.00000450890000536, -0.4149655844399999793 ) ) ;
#28373=CARTESIAN_POINT ( 'NONE',  ( -5.969238273219999336, -101.2530993000000024, 13.97222956260000082 ) ) ;
#28374=ADVANCED_FACE ( 'NONE', ( #4502 ), #23642, .F. ) ;
#28381=CARTESIAN_POINT ( 'NONE',  ( -18.93875617240000153, -93.07693985719998864, -21.17499315530000104 ) ) ;
#28385=CARTESIAN_POINT ( 'NONE',  ( 13.59944669439999920, -100.1512121650000040, -9.587914801669999321 ) ) ;
#28389=CARTESIAN_POINT ( 'NONE',  ( 0.3872056760440000245, -101.1889999979999999, -17.35614698070000017 ) ) ;
#28391=PLANE ( 'NONE',  #23461 ) ;
#28395=CARTESIAN_POINT ( 'NONE',  ( -0.1180621203445222367, -92.72059904818335951, -30.49977178675158029 ) ) ;
#28399=ADVANCED_FACE ( 'NONE', ( #15114 ), #11523, .F. ) ;
#28403=ORIENTED_EDGE ( 'NONE', *, *, #19731, .T. ) ;
#28408=CARTESIAN_POINT ( 'NONE',  ( 11.96443931099999958, -96.83683775170000274, 17.18597302079999878 ) ) ;
#28410=CARTESIAN_POINT ( 'NONE',  ( -14.12278956529999974, -93.04972065580000162, -23.64156151090000080 ) ) ;
#28417=CARTESIAN_POINT ( 'NONE',  ( 0.000000000000000000, -107.5000000000000000, 0.000000000000000000 ) ) ;
#28418=ORIENTED_EDGE ( 'NONE', *, *, #15047, .F. ) ;
#28420=CARTESIAN_POINT ( 'NONE',  ( 13.59220273991967609, -100.4872618013039158, -10.06240860112436941 ) ) ;
#28424=CARTESIAN_POINT ( 'NONE',  ( 9.273496252050001942, -94.57749834670001121, -22.35125233299999792 ) ) ;
#28427=AXIS2_PLACEMENT_3D ( 'NONE', #7713, #14112, #21110 ) ;
#28440=CARTESIAN_POINT ( 'NONE',  ( 7.181689937160000703, -99.92967571559999840, 15.80535030819999953 ) ) ;
#28441=CARTESIAN_POINT ( 'NONE',  ( 15.72706581430000128, -101.2251655520000071, 3.980808227969999447 ) ) ;
#28444=ORIENTED_EDGE ( 'NONE', *, *, #20364, .T. ) ;
#28446=CARTESIAN_POINT ( 'NONE',  ( 6.008696179649185787, -92.50638022835023833, -29.90261591053662471 ) ) ;
#28449=CARTESIAN_POINT ( 'NONE',  ( 1.937685342960000057, -92.76004107139999633, -29.70233978819999976 ) ) ;
#28451=B_SPLINE_SURFACE_WITH_KNOTS ( 'NONE', 5, 5, ( 
 ( #5586, #8315, #6135, #23510, #28154, #23638, #23366, #27871, #5723 ),
 ( #16803, #10215, #15009, #25696, #3547, #19129, #28018, #25967, #8056 ),
 ( #8187, #23779, #12684, #21593, #10488, #13264, #4245, #13117, #8889 ),
 ( #20272, #21878, #4682, #9042, #12964, #6282, #24356, #24653, #4396 ),
 ( #13563, #22469, #22172, #11216, #26539, #2513, #26842, #1931, #11368 ),
 ( #340, #8740, #15148, #26693, #24498, #19683, #24056, #6734, #2212 ),
 ( #4096, #17948, #6582, #22029, #15443, #9183, #20124, #10770, #2077 ),
 ( #15599, #17509, #28572, #28700, #8607, #41, #26394, #17802, #17657 ),
 ( #6424, #15287, #26260, #24209, #10916, #19824, #11055, #19971, #4531 ) ),
 .UNSPECIFIED., .F., .F., .F.,
 ( 6, 3, 6 ),
 ( 6, 3, 6 ),
 ( 54.97253517989999949, 63.48927009810000044, 72.86859331460000533 ),
 ( 0.000000000000000000, 0.2500000000000000000, 0.5000000000000000000 ),
 .UNSPECIFIED. ) ;
#28452=CARTESIAN_POINT ( 'NONE',  ( 6.877703509944694815, -101.5829753080977298, 14.50225318756008974 ) ) ;
#28453=CARTESIAN_POINT ( 'NONE',  ( -6.729715370570000132, -101.1284992150000051, 13.85798327430000043 ) ) ;
#28455=LINE ( 'NONE', #23807, #21349 ) ;
#28458=CARTESIAN_POINT ( 'NONE',  ( 24.64041555829999908, -93.75379239679999444, -3.870821881539999954 ) ) ;
#28459=CARTESIAN_POINT ( 'NONE',  ( 11.24690583532123256, -93.66270333200120035, -23.43420612766421485 ) ) ;
#28463=CARTESIAN_POINT ( 'NONE',  ( -20.71870563330397275, -92.77481473461477890, -22.38281498381969925 ) ) ;
#28469=CARTESIAN_POINT ( 'NONE',  ( 23.96368475870000125, -92.50000000000000000, 8.717328305520000598 ) ) ;
#28478=B_SPLINE_CURVE_WITH_KNOTS ( 'NONE', 3,
 ( #4141, #6475, #22074, #6628, #85, #26881, #4727, #8786, #17698, #15489, #24399, #4436, #8935, #6920, #2257, #24538, #19727, #13607, #13166, #17845, #9086, #11103, #20016, #19866, #15786, #2121, #15336, #24253, #4292, #13306, #26742, #22211, #6777, #22515, #4579, #13458, #11409 ),
 .UNSPECIFIED., .F., .F.,
 ( 4, 2, 2, 1, 1, 1, 2, 2, 2, 2, 1, 1, 1, 2, 2, 2, 2, 1, 1, 1, 2, 2, 4 ),
 ( 0.000000000000000000, 0.1250000000000152656, 0.1875000000000219269, 0.2187500000000252576, 0.2343750000000270339, 0.2421875000000283662, 0.2460937500000285050, 0.2500000000000286438, 0.3750000000000290323, 0.4375000000000291434, 0.4687500000000289213, 0.4843750000000290878, 0.4921875000000295874, 0.4960937500000296985, 0.5000000000000298650, 0.6250000000000226485, 0.6875000000000187628, 0.7187500000000167644, 0.7343750000000157652, 0.7421875000000152101, 0.7460937500000150990, 0.7500000000000148770, 1.000000000000000000 ),
 .UNSPECIFIED. ) ;
#28486=ORIENTED_EDGE ( 'NONE', *, *, #9296, .F. ) ;
#28492=CARTESIAN_POINT ( 'NONE',  ( -7.498699138939999287, -94.79581646409999962, -22.45487619560000070 ) ) ;
#28494=CARTESIAN_POINT ( 'NONE',  ( -20.30783661097642678, -96.61062616337834186, -6.202245570597845870 ) ) ;
#28495=CARTESIAN_POINT ( 'NONE',  ( -13.14229091329999832, -100.8869817940000075, -8.528547626079999944 ) ) ;
#28496=EDGE_CURVE ( 'NONE', #5829, #8703, #20694, .T. ) ;
#28499=CARTESIAN_POINT ( 'NONE',  ( 16.08037959500000014, -101.1889999979999999, 2.354223078750000031 ) ) ;
#28500=CARTESIAN_POINT ( 'NONE',  ( -11.76437930720000047, -100.8023006570000035, -10.51170590289999929 ) ) ;
#28502=CARTESIAN_POINT ( 'NONE',  ( -7.701451075213345376, -100.9229461894397843, 14.66641892369707278 ) ) ;
#28511=CARTESIAN_POINT ( 'NONE',  ( -30.31271238969999970, -92.50000000000000000, 0.1252161350790000072 ) ) ;
#28513=CARTESIAN_POINT ( 'NONE',  ( 12.03044342970000002, -92.63020460699999603, 27.45853671740000124 ) ) ;
#28517=CARTESIAN_POINT ( 'NONE',  ( -19.83822443902547050, -96.11102763504688085, 9.124294855013181049 ) ) ;
#28518=ORIENTED_EDGE ( 'NONE', *, *, #21102, .T. ) ;
#28520=CARTESIAN_POINT ( 'NONE',  ( -14.86197364899999940, -100.8869795979999964, 4.957594172660000353 ) ) ;
#28526=CARTESIAN_POINT ( 'NONE',  ( -23.49132533670000100, -92.92146929989999649, -19.26888038349999732 ) ) ;
#28529=CARTESIAN_POINT ( 'NONE',  ( -6.065234971653478802, -101.5839620086842388, 14.85812437776191963 ) ) ;
#28530=CARTESIAN_POINT ( 'NONE',  ( 13.74656640350000103, -99.97545561319999763, -9.830828057420001542 ) ) ;
#28531=CARTESIAN_POINT ( 'NONE',  ( -18.75664408759999802, -92.68584073459999217, 22.80736227010000050 ) ) ;
#28532=ADVANCED_FACE ( 'NONE', ( #7988 ), #14810, .T. ) ;
#28536=DIRECTION ( 'NONE',  ( 0.000000000000000000, 1.000000000000000000, 0.000000000000000000 ) ) ;
#28540=CARTESIAN_POINT ( 'NONE',  ( -24.15983059781524389, -92.58347372262571184, -18.61592446762897879 ) ) ;
#28541=CARTESIAN_POINT ( 'NONE',  ( 14.05983645159999895, -99.53431386179998697, -10.27466725399999881 ) ) ;
#28543=CARTESIAN_POINT ( 'NONE',  ( -0.8786661444248782260, -92.52249206705035078, -30.48734580142448536 ) ) ;
#28546=CARTESIAN_POINT ( 'NONE',  ( 0.000000000000000000, -102.5000000000000000, 0.000000000000000000 ) ) ;
#28548=AXIS2_PLACEMENT_3D ( 'NONE', #8855, #4361, #15410 ) ;
#28549=CARTESIAN_POINT ( 'NONE',  ( 21.19481781799999709, -97.14975610550000340, -2.160707968160000103 ) ) ;
#28556=CARTESIAN_POINT ( 'NONE',  ( -13.14595372920000038, -93.06132229930000221, -23.62747770269999847 ) ) ;
#28558=CARTESIAN_POINT ( 'NONE',  ( 8.188637977920000921, -100.9197082849999987, 13.30686163390000054 ) ) ;
#28559=CARTESIAN_POINT ( 'NONE',  ( -30.40445704718852227, -92.82044061123613687, 2.412276836114850553 ) ) ;
#28565=CARTESIAN_POINT ( 'NONE',  ( 13.63352270484119977, -100.4103893717064437, -10.10970819179740587 ) ) ;
#28572=CARTESIAN_POINT ( 'NONE',  ( -14.17503812420000031, -92.50889039439999806, 25.96392922189999908 ) ) ;
#28573=CARTESIAN_POINT ( 'NONE',  ( -20.62204820664130978, -93.91746156109596200, 13.70703326616601636 ) ) ;
#28574=ORIENTED_EDGE ( 'NONE', *, *, #4741, .T. ) ;
#28577=CARTESIAN_POINT ( 'NONE',  ( 0.7851461961000000267, -99.77922884479998800, -17.12662525980000083 ) ) ;
#28583=ORIENTED_EDGE ( 'NONE', *, *, #4173, .T. ) ;
#28585=CARTESIAN_POINT ( 'NONE',  ( 15.59178597810000078, -101.4254868729999970, 3.450949677659999715 ) ) ;
#28586=CARTESIAN_POINT ( 'NONE',  ( -5.914019803513142826, -97.43430234653058619, 19.69980648870009787 ) ) ;
#28589=CARTESIAN_POINT ( 'NONE',  ( 5.670030758810195692, -92.54383083955174527, -29.96833535579921204 ) ) ;
#28591=LINE ( 'NONE', #26413, #16264 ) ;
#28592=CARTESIAN_POINT ( 'NONE',  ( 8.096956726469999310, -93.90388142500000868, -24.52623309450000377 ) ) ;
#28594=CARTESIAN_POINT ( 'NONE',  ( -6.853461900220000125, -101.5369810359999860, 14.45809094780000059 ) ) ;
#28597=CARTESIAN_POINT ( 'NONE',  ( -12.56783578032861115, -100.9616911410483056, -10.74506713166292116 ) ) ;
#28600=CARTESIAN_POINT ( 'NONE',  ( 26.92509574520000015, -92.51556042380001088, -10.07865068210000103 ) ) ;
#28601=CARTESIAN_POINT ( 'NONE',  ( -1.161294068250000144, -101.3399913430000083, -16.09112164460000116 ) ) ;
#28605=CARTESIAN_POINT ( 'NONE',  ( -20.85953344891709449, -92.82668962667167989, -22.25151384493802809 ) ) ;
#28609=CARTESIAN_POINT ( 'NONE',  ( 16.30128245607246740, -94.65384004866649548, 17.22816601156467087 ) ) ;
#28616=ORIENTED_EDGE ( 'NONE', *, *, #22419, .F. ) ;
#28622=CARTESIAN_POINT ( 'NONE',  ( -25.65917880860000011, -93.81709628030000658, -2.425942638370000015 ) ) ;
#28625=CIRCLE ( 'NONE', #10015, 29.91857981989999971 ) ;
#28629=VERTEX_POINT ( 'NONE', #7216 ) ;
#28635=ADVANCED_FACE ( 'NONE', ( #11710 ), #1765, .T. ) ;
#28636=CARTESIAN_POINT ( 'NONE',  ( -15.46754588249999962, -101.3256027139999986, 3.711833783079999449 ) ) ;
#28640=CARTESIAN_POINT ( 'NONE',  ( -12.36870887870000146, -101.2063419769999939, -10.12880706900000050 ) ) ;
#28642=CARTESIAN_POINT ( 'NONE',  ( -13.15684669475222535, -99.57060688045895347, -11.33663430084732937 ) ) ;
#28643=ORIENTED_EDGE ( 'NONE', *, *, #10049, .F. ) ;
#28648=FACE_OUTER_BOUND ( 'NONE', #24188, .T. ) ;
#28650=CARTESIAN_POINT ( 'NONE',  ( -19.07296793847176275, -97.32367535544746318, 6.861303669024300333 ) ) ;
#28652=CARTESIAN_POINT ( 'NONE',  ( 21.78490392830000033, -93.61368451529999390, 12.86422805260000146 ) ) ;
#28658=CARTESIAN_POINT ( 'NONE',  ( 12.45454819569999927, -101.6484611540000031, -10.04451848439999928 ) ) ;
#28659=CARTESIAN_POINT ( 'NONE',  ( -16.42874499639999897, -93.07154530329999886, -21.42660670609999940 ) ) ;
#28664=CARTESIAN_POINT ( 'NONE',  ( 12.51978528759999953, -101.0678230150000019, -9.676466934249999596 ) ) ;
#28666=CARTESIAN_POINT ( 'NONE',  ( -11.76876535810587043, -94.80026864432733191, -21.40432527480584923 ) ) ;
#28672=B_SPLINE_CURVE_WITH_KNOTS ( 'NONE', 5,
 ( #6540, #19784, #17912, #4355, #24169, #22580, #28666, #8698, #17614 ),
 .UNSPECIFIED., .F., .F.,
 ( 6, 3, 6 ),
 ( 0.000000000000000000, 0.5000000000000000000, 1.000000000000000000 ),
 .UNSPECIFIED. ) ;
#28675=CARTESIAN_POINT ( 'NONE',  ( -0.4977272150621083191, -92.58608763743626469, -30.49593994900164162 ) ) ;
#28680=EDGE_CURVE ( 'NONE', #23314, #6421, #13274, .T. ) ;
#28681=CARTESIAN_POINT ( 'NONE',  ( 23.54314922829999901, -94.98812769020000246, -6.784139722789999993 ) ) ;
#28688=CARTESIAN_POINT ( 'NONE',  ( -8.810772439400000877, -95.92349949569999978, -20.47205490330000188 ) ) ;
#28689=CARTESIAN_POINT ( 'NONE',  ( 8.023929893669999203, -101.0253300669999987, 13.24802822849999906 ) ) ;
#28692=CARTESIAN_POINT ( 'NONE',  ( -29.41500720700000215, -92.50000000000000000, 8.062713625770001613 ) ) ;
#28694=CARTESIAN_POINT ( 'NONE',  ( 8.666173000869999754, -92.85282594270000800, -27.14333248820000222 ) ) ;
#28700=CARTESIAN_POINT ( 'NONE',  ( -14.23620810470000109, -92.53807957989999977, 26.01251215649999793 ) ) ;
#28705=CARTESIAN_POINT ( 'NONE',  ( 0.6376817541279999890, -100.7833805400000102, -15.89997782040000018 ) ) ;
#28707=CARTESIAN_POINT ( 'NONE',  ( 15.76357705000000209, -101.5369810359999860, 2.742715859449999627 ) ) ;
#28708=CIRCLE ( 'NONE', #14089, 29.91857981989999971 ) ;
#28711=DIRECTION ( 'NONE',  ( 1.000000000000000000, 0.000000000000000000, 0.000000000000000000 ) ) ;
#28712=LINE ( 'NONE', #10929, #19470 ) ;
#28717=CARTESIAN_POINT ( 'NONE',  ( 15.74335372270872746, -101.5555610555564101, 2.854262349832874079 ) ) ;
#28718=CARTESIAN_POINT ( 'NONE',  ( -5.553447374120000113, -96.83679384949999758, 20.51777214570000041 ) ) ;
#28720=CARTESIAN_POINT ( 'NONE',  ( -19.51835093920258757, -96.93405628829036402, 8.497249192397697826 ) ) ;
#28722=AXIS2_PLACEMENT_3D ( 'NONE', #28546, #8582, #17485 ) ;
#28724=CARTESIAN_POINT ( 'NONE',  ( -1.604070449259999753, -100.9197075889999979, -15.54198650660000069 ) ) ;
#28725=CARTESIAN_POINT ( 'NONE',  ( -6.623023768749999540, -101.1411470200000053, 13.89158803029999945 ) ) ;
#28728=CARTESIAN_POINT ( 'NONE',  ( -12.66900072054220772, -100.7538407675254035, -10.87939260405267738 ) ) ;
#28729=ORIENTED_EDGE ( 'NONE', *, *, #12711, .T. ) ;
#28733=CARTESIAN_POINT ( 'NONE',  ( 7.761187578059999481, -99.03691213880000532, 16.30863471170000167 ) ) ;
#28736=B_SPLINE_CURVE_WITH_KNOTS ( 'NONE', 3,
 ( #3436, #16681, #16401, #20791, #27491, #1135, #9836, #10245, #18886, #14227, #12015, #7381, #7807, #14362, #7946, #16833, #27770, #992, #5338, #12159, #16247, #23255, #23116, #27337, #5189, #5473, #844, #16548, #25722, #25585, #5613, #23393, #7542, #3162, #12302, #21343, #14493, #25158, #19020, #5751, #18603, #21074, #14074, #11878, #14638, #23535, #1402, #1264, #27905, #9973, #22976, #21211, #3573, #12430, #3023, #9688, #25310, #20933, #18746 ),
 .UNSPECIFIED., .F., .F.,
 ( 4, 2, 1, 1, 2, 2, 2, 2, 1, 1, 2, 2, 2, 2, 2, 2, 2, 1, 1, 2, 2, 2, 1, 1, 2, 2, 2, 1, 2, 2, 2, 2, 2, 4 ),
 ( 0.000000000000000000, 0.06249999999985383914, 0.09374999999978189669, 0.1093749999997448569, 0.1171874999997315620, 0.1249999999997182809, 0.1874999999995992372, 0.2187499999995454747, 0.2343749999995239919, 0.2421874999995143329, 0.2460937499995147215, 0.2499999999995151101, 0.3124999999997628564, 0.3437499999998855360, 0.3750000000000082712, 0.4375000000002447487, 0.4687500000003571587, 0.4843750000004051759, 0.4921875000004216072, 0.4960937500004218847, 0.5000000000004221068, 0.5625000000003723688, 0.5937500000003522738, 0.6093750000003471667, 0.6171875000003433920, 0.6250000000003395062, 0.6875000000002615685, 0.7187500000002227107, 0.7343750000002021716, 0.7500000000001816325, 0.8125000000001308953, 0.8437500000001064704, 0.8750000000000820455, 1.000000000000000000 ),
 .UNSPECIFIED. ) ;
#28739=CARTESIAN_POINT ( 'NONE',  ( -14.64568764270000045, -101.2530996969999961, 4.044604081960000208 ) ) ;
#28740=CARTESIAN_POINT ( 'NONE',  ( -8.001416342079998856, -100.4792519539999915, 14.07906887139999874 ) ) ;
#28741=LINE ( 'NONE', #235, #16472 ) ;
#28746=CARTESIAN_POINT ( 'NONE',  ( 24.74241209330589797, -93.18010901132686286, -14.18012848625775746 ) ) ;
#28750=AXIS2_PLACEMENT_3D ( 'NONE', #22872, #25481, #16294 ) ;
#28753=DIRECTION ( 'NONE',  ( 0.000000000000000000, 1.000000000000000000, 0.000000000000000000 ) ) ;
#28756=CARTESIAN_POINT ( 'NONE',  ( -25.14533824960000175, -93.65023553229998754, -2.072119361189999953 ) ) ;
#28760=EDGE_CURVE ( 'NONE', #20241, #8703, #27829, .T. ) ;
#28762=CARTESIAN_POINT ( 'NONE',  ( 16.03799742140000006, -100.8746138070000029, 4.294561568749999836 ) ) ;
#28770=CARTESIAN_POINT ( 'NONE',  ( 0.5880502493170355338, -99.62767017963351179, -17.32703895575575004 ) ) ;
#28774=CARTESIAN_POINT ( 'NONE',  ( 24.36857893470000036, -92.99570653130000153, -11.25322410160000075 ) ) ;
#28775=PLANE ( 'NONE',  #2981 ) ;
#28777=CARTESIAN_POINT ( 'NONE',  ( 14.31067114689999897, -98.53908914310000000, -12.11010054220000143 ) ) ;
#28779=CARTESIAN_POINT ( 'NONE',  ( -15.44795072159999982, -101.4309506800000094, 4.757508573860000034 ) ) ;
#28783=CARTESIAN_POINT ( 'NONE',  ( -13.28489450998225685, -99.84800943042500876, -11.12833488179714081 ) ) ;
#28784=ORIENTED_EDGE ( 'NONE', *, *, #24311, .F. ) ;
#28791=CIRCLE ( 'NONE', #23691, 29.91857981989999971 ) ;
#28793=DIRECTION ( 'NONE',  ( 0.4794255386042042266, 0.000000000000000000, 0.8775825618903720926 ) ) ;
#28798=CARTESIAN_POINT ( 'NONE',  ( -19.25397897833660821, -97.06701639843478802, 7.326875019138189948 ) ) ;
#28800=CARTESIAN_POINT ( 'NONE',  ( 25.83673624310000250, -92.67327661130001104, 10.43148741010000080 ) ) ;
ENDSEC;
END-ISO-10303-21;
